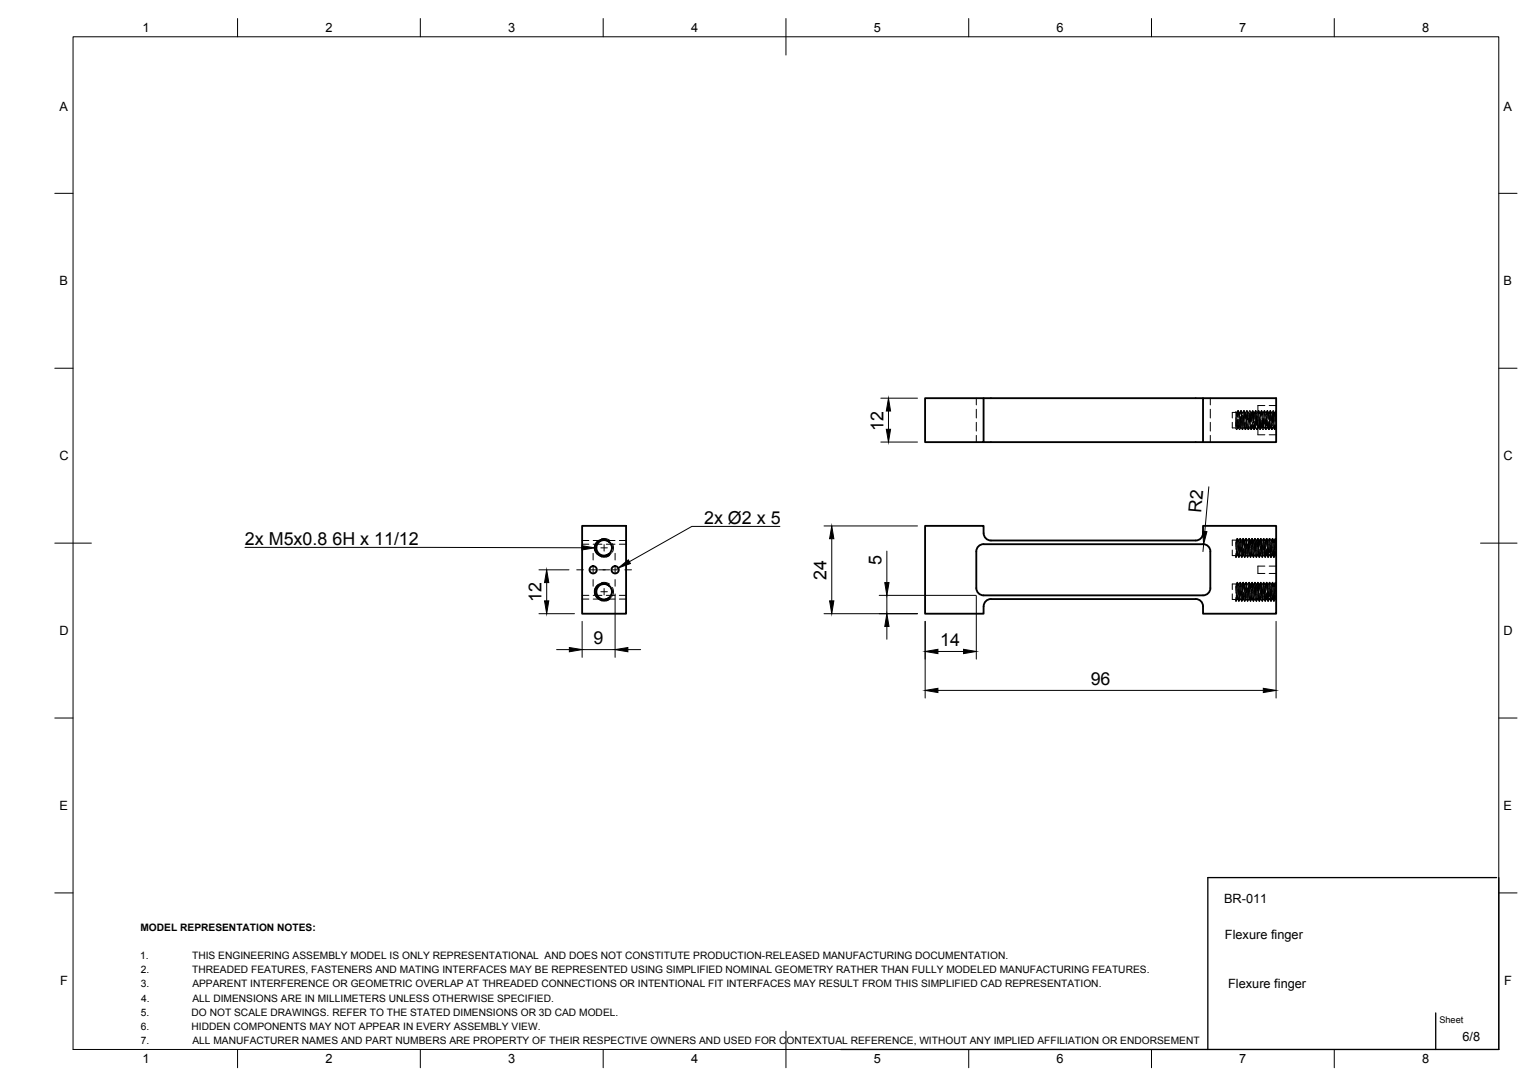
ISO-10303-21;
HEADER;
/* Generated by software containing ST-Developer
 * from STEP Tools, Inc. (www.steptools.com) 
 */

FILE_DESCRIPTION(
/* description */ ('Independent pair of monolithic parallel-leaf compliant finger modules.
 Shared native part/module instances; external gripper actuator outsid
e scope. Whole-mm geometry,1mm webs,56mm straight span,12mm depth,32mm
 nominal contact gap. Undeformed CAD reference; material condition, el
astic range, fatigue and gripping force unassigned.'),
/* implementation_level */ '2;1');

FILE_NAME(
/* name */ 'Flexure finger.step',
/* time_stamp */ '2026-11-07T22:36:16-08:00',
/* author */ (''),
/* organization */ (''),
/* preprocessor_version */ 'ST-DEVELOPER v20.2',
/* originating_system */ 'Autodesk Translation Framework v15.17.0.0',
/* authorisation */ '');

FILE_SCHEMA (('AUTOMOTIVE_DESIGN { 1 0 10303 214 3 1 1 }'));
ENDSEC;

DATA;
#10=MECHANICAL_DESIGN_GEOMETRIC_PRESENTATION_REPRESENTATION('',(#330),#13801);
#56=B_SPLINE_SURFACE_WITH_KNOTS('',3,3,((#7071,#7072,#7073,#7074,#7075,
#7076,#7077,#7078,#7079,#7080,#7081,#7082,#7083,#7084,#7085,#7086,#7087,
#7088,#7089,#7090,#7091,#7092,#7093,#7094,#7095,#7096,#7097,#7098,#7099,
#7100,#7101,#7102,#7103,#7104,#7105,#7106,#7107,#7108,#7109,#7110,#7111,
#7112,#7113,#7114,#7115,#7116,#7117,#7118,#7119,#7120,#7121,#7122,#7123,
#7124,#7125,#7126,#7127,#7128,#7129,#7130,#7131,#7132,#7133,#7134,#7135,
#7136,#7137,#7138,#7139,#7140,#7141,#7142,#7143,#7144,#7145,#7146,#7147,
#7148,#7149,#7150,#7151,#7152,#7153,#7154,#7155,#7156,#7157,#7158,#7159,
#7160,#7161,#7162),(#7163,#7164,#7165,#7166,#7167,#7168,#7169,#7170,#7171,
#7172,#7173,#7174,#7175,#7176,#7177,#7178,#7179,#7180,#7181,#7182,#7183,
#7184,#7185,#7186,#7187,#7188,#7189,#7190,#7191,#7192,#7193,#7194,#7195,
#7196,#7197,#7198,#7199,#7200,#7201,#7202,#7203,#7204,#7205,#7206,#7207,
#7208,#7209,#7210,#7211,#7212,#7213,#7214,#7215,#7216,#7217,#7218,#7219,
#7220,#7221,#7222,#7223,#7224,#7225,#7226,#7227,#7228,#7229,#7230,#7231,
#7232,#7233,#7234,#7235,#7236,#7237,#7238,#7239,#7240,#7241,#7242,#7243,
#7244,#7245,#7246,#7247,#7248,#7249,#7250,#7251,#7252,#7253,#7254),(#7255,
#7256,#7257,#7258,#7259,#7260,#7261,#7262,#7263,#7264,#7265,#7266,#7267,
#7268,#7269,#7270,#7271,#7272,#7273,#7274,#7275,#7276,#7277,#7278,#7279,
#7280,#7281,#7282,#7283,#7284,#7285,#7286,#7287,#7288,#7289,#7290,#7291,
#7292,#7293,#7294,#7295,#7296,#7297,#7298,#7299,#7300,#7301,#7302,#7303,
#7304,#7305,#7306,#7307,#7308,#7309,#7310,#7311,#7312,#7313,#7314,#7315,
#7316,#7317,#7318,#7319,#7320,#7321,#7322,#7323,#7324,#7325,#7326,#7327,
#7328,#7329,#7330,#7331,#7332,#7333,#7334,#7335,#7336,#7337,#7338,#7339,
#7340,#7341,#7342,#7343,#7344,#7345,#7346),(#7347,#7348,#7349,#7350,#7351,
#7352,#7353,#7354,#7355,#7356,#7357,#7358,#7359,#7360,#7361,#7362,#7363,
#7364,#7365,#7366,#7367,#7368,#7369,#7370,#7371,#7372,#7373,#7374,#7375,
#7376,#7377,#7378,#7379,#7380,#7381,#7382,#7383,#7384,#7385,#7386,#7387,
#7388,#7389,#7390,#7391,#7392,#7393,#7394,#7395,#7396,#7397,#7398,#7399,
#7400,#7401,#7402,#7403,#7404,#7405,#7406,#7407,#7408,#7409,#7410,#7411,
#7412,#7413,#7414,#7415,#7416,#7417,#7418,#7419,#7420,#7421,#7422,#7423,
#7424,#7425,#7426,#7427,#7428,#7429,#7430,#7431,#7432,#7433,#7434,#7435,
#7436,#7437,#7438)),.UNSPECIFIED.,.F.,.F.,.F.,(4,4),(4,1,1,1,1,1,1,1,1,
1,1,1,1,1,1,1,1,1,1,1,1,1,1,1,1,1,1,1,1,1,1,1,1,1,1,1,1,1,1,1,1,1,1,1,1,
1,1,1,1,1,1,1,1,1,1,1,1,1,1,1,1,1,1,1,1,1,1,1,1,1,1,1,1,1,1,1,1,1,1,1,1,
1,1,1,1,1,1,1,1,4),(0.,0.0511532338502008),(11.8669242345263,12.8602116589039,
13.8534990832815,14.8467865076592,15.8400739320368,16.8333613564144,17.826648780792,
18.8199362051697,19.8132236295473,20.8065110539249,21.7997984783025,22.7930859026802,
23.7863733270578,24.7796607514354,25.772948175813,26.7662356001907,27.7595230245683,
28.7528104489459,29.7460978733235,30.7393852977012,31.7326727220788,32.7259601464564,
33.719247570834,34.7125349952117,35.7058224195893,36.6991098439669,37.6923972683445,
38.6856846927222,39.6789721170998,40.6722595414774,41.6655469658551,42.6588343902327,
43.6521218146103,44.6454092389879,45.6386966633656,46.6319840877432,47.6252715121208,
48.6185589364984,49.6118463608761,50.6051337852537,51.5984212096313,52.5917086340089,
53.5849960583866,54.5782834827642,55.5715709071418,56.5648583315194,57.5581457558971,
58.5514331802747,59.5447206046523,60.5380080290299,61.5312954534076,62.5245828777852,
63.5178703021628,64.5111577265404,65.5044451509181,66.4977325752957,67.4910199996733,
68.4843074240509,69.4775948484286,70.4708822728062,71.4641696971838,72.4574571215614,
73.4507445459391,74.4440319703167,75.4373193946943,76.430606819072,77.4238942434496,
78.4171816678272,79.4104690922048,80.4037565165825,81.3970439409601,82.3903313653377,
83.3836187897153,84.376906214093,85.3701936384706,86.3634810628482,87.3567684872258,
88.3500559116035,89.3433433359811,90.3366307603587,91.3299181847363,92.323205609114,
93.3164930334916,94.3097804578692,95.3030678822468,96.2963553066245,97.2896427310021,
98.2829301553797,99.2762175797573,100.269505004135),.UNSPECIFIED.);
#57=B_SPLINE_SURFACE_WITH_KNOTS('',3,3,((#7555,#7556,#7557,#7558,#7559,
#7560,#7561,#7562,#7563,#7564,#7565,#7566,#7567,#7568,#7569,#7570,#7571,
#7572,#7573,#7574,#7575,#7576,#7577,#7578,#7579,#7580,#7581,#7582,#7583,
#7584,#7585,#7586,#7587,#7588,#7589,#7590,#7591,#7592,#7593,#7594,#7595,
#7596,#7597,#7598,#7599,#7600,#7601,#7602,#7603,#7604,#7605,#7606,#7607,
#7608,#7609,#7610,#7611,#7612,#7613,#7614,#7615,#7616,#7617,#7618,#7619,
#7620,#7621,#7622,#7623,#7624,#7625,#7626,#7627,#7628,#7629,#7630,#7631,
#7632,#7633,#7634,#7635,#7636,#7637,#7638,#7639,#7640,#7641,#7642,#7643,
#7644,#7645,#7646),(#7647,#7648,#7649,#7650,#7651,#7652,#7653,#7654,#7655,
#7656,#7657,#7658,#7659,#7660,#7661,#7662,#7663,#7664,#7665,#7666,#7667,
#7668,#7669,#7670,#7671,#7672,#7673,#7674,#7675,#7676,#7677,#7678,#7679,
#7680,#7681,#7682,#7683,#7684,#7685,#7686,#7687,#7688,#7689,#7690,#7691,
#7692,#7693,#7694,#7695,#7696,#7697,#7698,#7699,#7700,#7701,#7702,#7703,
#7704,#7705,#7706,#7707,#7708,#7709,#7710,#7711,#7712,#7713,#7714,#7715,
#7716,#7717,#7718,#7719,#7720,#7721,#7722,#7723,#7724,#7725,#7726,#7727,
#7728,#7729,#7730,#7731,#7732,#7733,#7734,#7735,#7736,#7737,#7738),(#7739,
#7740,#7741,#7742,#7743,#7744,#7745,#7746,#7747,#7748,#7749,#7750,#7751,
#7752,#7753,#7754,#7755,#7756,#7757,#7758,#7759,#7760,#7761,#7762,#7763,
#7764,#7765,#7766,#7767,#7768,#7769,#7770,#7771,#7772,#7773,#7774,#7775,
#7776,#7777,#7778,#7779,#7780,#7781,#7782,#7783,#7784,#7785,#7786,#7787,
#7788,#7789,#7790,#7791,#7792,#7793,#7794,#7795,#7796,#7797,#7798,#7799,
#7800,#7801,#7802,#7803,#7804,#7805,#7806,#7807,#7808,#7809,#7810,#7811,
#7812,#7813,#7814,#7815,#7816,#7817,#7818,#7819,#7820,#7821,#7822,#7823,
#7824,#7825,#7826,#7827,#7828,#7829,#7830),(#7831,#7832,#7833,#7834,#7835,
#7836,#7837,#7838,#7839,#7840,#7841,#7842,#7843,#7844,#7845,#7846,#7847,
#7848,#7849,#7850,#7851,#7852,#7853,#7854,#7855,#7856,#7857,#7858,#7859,
#7860,#7861,#7862,#7863,#7864,#7865,#7866,#7867,#7868,#7869,#7870,#7871,
#7872,#7873,#7874,#7875,#7876,#7877,#7878,#7879,#7880,#7881,#7882,#7883,
#7884,#7885,#7886,#7887,#7888,#7889,#7890,#7891,#7892,#7893,#7894,#7895,
#7896,#7897,#7898,#7899,#7900,#7901,#7902,#7903,#7904,#7905,#7906,#7907,
#7908,#7909,#7910,#7911,#7912,#7913,#7914,#7915,#7916,#7917,#7918,#7919,
#7920,#7921,#7922)),.UNSPECIFIED.,.F.,.F.,.F.,(4,4),(4,1,1,1,1,1,1,1,1,
1,1,1,1,1,1,1,1,1,1,1,1,1,1,1,1,1,1,1,1,1,1,1,1,1,1,1,1,1,1,1,1,1,1,1,1,
1,1,1,1,1,1,1,1,1,1,1,1,1,1,1,1,1,1,1,1,1,1,1,1,1,1,1,1,1,1,1,1,1,1,1,1,
1,1,1,1,1,1,1,1,4),(0.,0.0511532338502008),(14.3986268518923,15.3919142762699,
16.3852017006476,17.3784891250252,18.3717765494028,19.3650639737804,20.3583513981581,
21.3516388225357,22.3449262469133,23.3382136712909,24.3315010956686,25.3247885200462,
26.3180759444238,27.3113633688014,28.3046507931791,29.2979382175567,30.2912256419343,
31.284513066312,32.2778004906896,33.2710879150672,34.2643753394448,35.2576627638225,
36.2509501882001,37.2442376125777,38.2375250369553,39.230812461333,40.2240998857106,
41.2173873100882,42.2106747344658,43.2039621588435,44.1972495832211,45.1905370075987,
46.1838244319763,47.177111856354,48.1703992807316,49.1636867051092,50.1569741294868,
51.1502615538645,52.1435489782421,53.1368364026197,54.1301238269973,55.123411251375,
56.1166986757526,57.1099861001302,58.1032735245078,59.0965609488855,60.0898483732631,
61.0831357976407,62.0764232220183,63.069710646396,64.0629980707736,65.0562854951512,
66.0495729195289,67.0428603439065,68.0361477682841,69.0294351926617,70.0227226170393,
71.016010041417,72.0092974657946,73.0025848901722,73.9958723145499,74.9891597389275,
75.9824471633051,76.9757345876827,77.9690220120604,78.962309436438,79.9555968608156,
80.9488842851932,81.9421717095709,82.9354591339485,83.9287465583261,84.9220339827037,
85.9153214070814,86.908608831459,87.9018962558366,88.8951836802142,89.8884711045919,
90.8817585289695,91.8750459533471,92.8683333777248,93.8616208021024,94.85490822648,
95.8481956508576,96.8414830752353,97.8347704996129,98.8280579239905,99.8213453483681,
100.814632772746,101.807920197123,102.801207621501),.UNSPECIFIED.);
#58=B_SPLINE_SURFACE_WITH_KNOTS('',3,3,((#8239,#8240,#8241,#8242,#8243,
#8244,#8245,#8246,#8247,#8248,#8249,#8250,#8251,#8252,#8253,#8254,#8255,
#8256,#8257,#8258,#8259,#8260,#8261,#8262,#8263,#8264,#8265,#8266,#8267,
#8268,#8269,#8270,#8271,#8272,#8273,#8274,#8275,#8276,#8277,#8278,#8279,
#8280,#8281,#8282,#8283,#8284,#8285,#8286,#8287,#8288,#8289,#8290,#8291,
#8292,#8293,#8294,#8295,#8296,#8297,#8298,#8299,#8300,#8301,#8302,#8303,
#8304,#8305,#8306,#8307,#8308,#8309,#8310,#8311,#8312,#8313,#8314,#8315,
#8316,#8317,#8318,#8319,#8320,#8321,#8322,#8323,#8324,#8325,#8326,#8327,
#8328,#8329,#8330),(#8331,#8332,#8333,#8334,#8335,#8336,#8337,#8338,#8339,
#8340,#8341,#8342,#8343,#8344,#8345,#8346,#8347,#8348,#8349,#8350,#8351,
#8352,#8353,#8354,#8355,#8356,#8357,#8358,#8359,#8360,#8361,#8362,#8363,
#8364,#8365,#8366,#8367,#8368,#8369,#8370,#8371,#8372,#8373,#8374,#8375,
#8376,#8377,#8378,#8379,#8380,#8381,#8382,#8383,#8384,#8385,#8386,#8387,
#8388,#8389,#8390,#8391,#8392,#8393,#8394,#8395,#8396,#8397,#8398,#8399,
#8400,#8401,#8402,#8403,#8404,#8405,#8406,#8407,#8408,#8409,#8410,#8411,
#8412,#8413,#8414,#8415,#8416,#8417,#8418,#8419,#8420,#8421,#8422),(#8423,
#8424,#8425,#8426,#8427,#8428,#8429,#8430,#8431,#8432,#8433,#8434,#8435,
#8436,#8437,#8438,#8439,#8440,#8441,#8442,#8443,#8444,#8445,#8446,#8447,
#8448,#8449,#8450,#8451,#8452,#8453,#8454,#8455,#8456,#8457,#8458,#8459,
#8460,#8461,#8462,#8463,#8464,#8465,#8466,#8467,#8468,#8469,#8470,#8471,
#8472,#8473,#8474,#8475,#8476,#8477,#8478,#8479,#8480,#8481,#8482,#8483,
#8484,#8485,#8486,#8487,#8488,#8489,#8490,#8491,#8492,#8493,#8494,#8495,
#8496,#8497,#8498,#8499,#8500,#8501,#8502,#8503,#8504,#8505,#8506,#8507,
#8508,#8509,#8510,#8511,#8512,#8513,#8514),(#8515,#8516,#8517,#8518,#8519,
#8520,#8521,#8522,#8523,#8524,#8525,#8526,#8527,#8528,#8529,#8530,#8531,
#8532,#8533,#8534,#8535,#8536,#8537,#8538,#8539,#8540,#8541,#8542,#8543,
#8544,#8545,#8546,#8547,#8548,#8549,#8550,#8551,#8552,#8553,#8554,#8555,
#8556,#8557,#8558,#8559,#8560,#8561,#8562,#8563,#8564,#8565,#8566,#8567,
#8568,#8569,#8570,#8571,#8572,#8573,#8574,#8575,#8576,#8577,#8578,#8579,
#8580,#8581,#8582,#8583,#8584,#8585,#8586,#8587,#8588,#8589,#8590,#8591,
#8592,#8593,#8594,#8595,#8596,#8597,#8598,#8599,#8600,#8601,#8602,#8603,
#8604,#8605,#8606)),.UNSPECIFIED.,.F.,.F.,.F.,(4,4),(4,1,1,1,1,1,1,1,1,
1,1,1,1,1,1,1,1,1,1,1,1,1,1,1,1,1,1,1,1,1,1,1,1,1,1,1,1,1,1,1,1,1,1,1,1,
1,1,1,1,1,1,1,1,1,1,1,1,1,1,1,1,1,1,1,1,1,1,1,1,1,1,1,1,1,1,1,1,1,1,1,1,
1,1,1,1,1,1,1,1,4),(0.,0.0511532338502008),(11.8669242345263,12.8602116589039,
13.8534990832815,14.8467865076592,15.8400739320368,16.8333613564144,17.826648780792,
18.8199362051697,19.8132236295473,20.8065110539249,21.7997984783025,22.7930859026802,
23.7863733270578,24.7796607514354,25.772948175813,26.7662356001907,27.7595230245683,
28.7528104489459,29.7460978733235,30.7393852977012,31.7326727220788,32.7259601464564,
33.719247570834,34.7125349952117,35.7058224195893,36.6991098439669,37.6923972683445,
38.6856846927222,39.6789721170998,40.6722595414774,41.6655469658551,42.6588343902327,
43.6521218146103,44.6454092389879,45.6386966633656,46.6319840877432,47.6252715121208,
48.6185589364984,49.6118463608761,50.6051337852537,51.5984212096313,52.5917086340089,
53.5849960583866,54.5782834827642,55.5715709071418,56.5648583315194,57.5581457558971,
58.5514331802747,59.5447206046523,60.5380080290299,61.5312954534076,62.5245828777852,
63.5178703021628,64.5111577265404,65.5044451509181,66.4977325752957,67.4910199996733,
68.4843074240509,69.4775948484286,70.4708822728062,71.4641696971838,72.4574571215614,
73.4507445459391,74.4440319703167,75.4373193946943,76.430606819072,77.4238942434496,
78.4171816678272,79.4104690922048,80.4037565165825,81.3970439409601,82.3903313653377,
83.3836187897153,84.376906214093,85.3701936384706,86.3634810628482,87.3567684872258,
88.3500559116035,89.3433433359811,90.3366307603587,91.3299181847363,92.323205609114,
93.3164930334916,94.3097804578692,95.3030678822468,96.2963553066245,97.2896427310021,
98.2829301553797,99.2762175797573,100.269505004135),.UNSPECIFIED.);
#59=B_SPLINE_SURFACE_WITH_KNOTS('',3,3,((#8723,#8724,#8725,#8726,#8727,
#8728,#8729,#8730,#8731,#8732,#8733,#8734,#8735,#8736,#8737,#8738,#8739,
#8740,#8741,#8742,#8743,#8744,#8745,#8746,#8747,#8748,#8749,#8750,#8751,
#8752,#8753,#8754,#8755,#8756,#8757,#8758,#8759,#8760,#8761,#8762,#8763,
#8764,#8765,#8766,#8767,#8768,#8769,#8770,#8771,#8772,#8773,#8774,#8775,
#8776,#8777,#8778,#8779,#8780,#8781,#8782,#8783,#8784,#8785,#8786,#8787,
#8788,#8789,#8790,#8791,#8792,#8793,#8794,#8795,#8796,#8797,#8798,#8799,
#8800,#8801,#8802,#8803,#8804,#8805,#8806,#8807,#8808,#8809,#8810,#8811,
#8812,#8813,#8814),(#8815,#8816,#8817,#8818,#8819,#8820,#8821,#8822,#8823,
#8824,#8825,#8826,#8827,#8828,#8829,#8830,#8831,#8832,#8833,#8834,#8835,
#8836,#8837,#8838,#8839,#8840,#8841,#8842,#8843,#8844,#8845,#8846,#8847,
#8848,#8849,#8850,#8851,#8852,#8853,#8854,#8855,#8856,#8857,#8858,#8859,
#8860,#8861,#8862,#8863,#8864,#8865,#8866,#8867,#8868,#8869,#8870,#8871,
#8872,#8873,#8874,#8875,#8876,#8877,#8878,#8879,#8880,#8881,#8882,#8883,
#8884,#8885,#8886,#8887,#8888,#8889,#8890,#8891,#8892,#8893,#8894,#8895,
#8896,#8897,#8898,#8899,#8900,#8901,#8902,#8903,#8904,#8905,#8906),(#8907,
#8908,#8909,#8910,#8911,#8912,#8913,#8914,#8915,#8916,#8917,#8918,#8919,
#8920,#8921,#8922,#8923,#8924,#8925,#8926,#8927,#8928,#8929,#8930,#8931,
#8932,#8933,#8934,#8935,#8936,#8937,#8938,#8939,#8940,#8941,#8942,#8943,
#8944,#8945,#8946,#8947,#8948,#8949,#8950,#8951,#8952,#8953,#8954,#8955,
#8956,#8957,#8958,#8959,#8960,#8961,#8962,#8963,#8964,#8965,#8966,#8967,
#8968,#8969,#8970,#8971,#8972,#8973,#8974,#8975,#8976,#8977,#8978,#8979,
#8980,#8981,#8982,#8983,#8984,#8985,#8986,#8987,#8988,#8989,#8990,#8991,
#8992,#8993,#8994,#8995,#8996,#8997,#8998),(#8999,#9000,#9001,#9002,#9003,
#9004,#9005,#9006,#9007,#9008,#9009,#9010,#9011,#9012,#9013,#9014,#9015,
#9016,#9017,#9018,#9019,#9020,#9021,#9022,#9023,#9024,#9025,#9026,#9027,
#9028,#9029,#9030,#9031,#9032,#9033,#9034,#9035,#9036,#9037,#9038,#9039,
#9040,#9041,#9042,#9043,#9044,#9045,#9046,#9047,#9048,#9049,#9050,#9051,
#9052,#9053,#9054,#9055,#9056,#9057,#9058,#9059,#9060,#9061,#9062,#9063,
#9064,#9065,#9066,#9067,#9068,#9069,#9070,#9071,#9072,#9073,#9074,#9075,
#9076,#9077,#9078,#9079,#9080,#9081,#9082,#9083,#9084,#9085,#9086,#9087,
#9088,#9089,#9090)),.UNSPECIFIED.,.F.,.F.,.F.,(4,4),(4,1,1,1,1,1,1,1,1,
1,1,1,1,1,1,1,1,1,1,1,1,1,1,1,1,1,1,1,1,1,1,1,1,1,1,1,1,1,1,1,1,1,1,1,1,
1,1,1,1,1,1,1,1,1,1,1,1,1,1,1,1,1,1,1,1,1,1,1,1,1,1,1,1,1,1,1,1,1,1,1,1,
1,1,1,1,1,1,1,1,4),(0.,0.0511532338502008),(14.3986268518923,15.3919142762699,
16.3852017006476,17.3784891250252,18.3717765494028,19.3650639737804,20.3583513981581,
21.3516388225357,22.3449262469133,23.3382136712909,24.3315010956686,25.3247885200462,
26.3180759444238,27.3113633688014,28.3046507931791,29.2979382175567,30.2912256419343,
31.284513066312,32.2778004906896,33.2710879150672,34.2643753394448,35.2576627638225,
36.2509501882001,37.2442376125777,38.2375250369553,39.230812461333,40.2240998857106,
41.2173873100882,42.2106747344658,43.2039621588435,44.1972495832211,45.1905370075987,
46.1838244319763,47.177111856354,48.1703992807316,49.1636867051092,50.1569741294868,
51.1502615538645,52.1435489782421,53.1368364026197,54.1301238269973,55.123411251375,
56.1166986757526,57.1099861001302,58.1032735245078,59.0965609488855,60.0898483732631,
61.0831357976407,62.0764232220183,63.069710646396,64.0629980707736,65.0562854951512,
66.0495729195289,67.0428603439065,68.0361477682841,69.0294351926617,70.0227226170393,
71.016010041417,72.0092974657946,73.0025848901722,73.9958723145499,74.9891597389275,
75.9824471633051,76.9757345876827,77.9690220120604,78.962309436438,79.9555968608156,
80.9488842851932,81.9421717095709,82.9354591339485,83.9287465583261,84.9220339827037,
85.9153214070814,86.908608831459,87.9018962558366,88.8951836802142,89.8884711045919,
90.8817585289695,91.8750459533471,92.8683333777248,93.8616208021024,94.85490822648,
95.8481956508576,96.8414830752353,97.8347704996129,98.8280579239905,99.8213453483681,
100.814632772746,101.807920197123,102.801207621501),.UNSPECIFIED.);
#62=B_SPLINE_CURVE_WITH_KNOTS('',3,(#4900,#4901,#4902,#4903,#4904,#4905,
#4906,#4907,#4908,#4909,#4910,#4911,#4912,#4913,#4914,#4915,#4916,#4917,
#4918),.UNSPECIFIED.,.F.,.F.,(4,3,3,3,3,3,4),(82.9907454093912,83.4361436477206,
84.4294310720982,85.4227184964758,86.4160059208535,87.4092933452311,88.4025807696087),
 .UNSPECIFIED.);
#63=B_SPLINE_CURVE_WITH_KNOTS('',3,(#4922,#4923,#4924,#4925),
 .UNSPECIFIED.,.F.,.F.,(4,4),(-86.3937979737193,-85.5224480267573),
 .UNSPECIFIED.);
#64=B_SPLINE_CURVE_WITH_KNOTS('',3,(#4929,#4930,#4931,#4932,#4933,#4934,
#4935,#4936,#4937,#4938,#4939,#4940,#4941,#4942,#4943,#4944,#4945,#4946,
#4947,#4948,#4949,#4950,#4951,#4952,#4953),.UNSPECIFIED.,.F.,.F.,(4,3,3,
3,3,3,3,3,4),(-85.5224480267573,-85.4227184964758,-84.4294310720982,-83.4361436477206,
-82.442856223343,-81.4495687989653,-80.4562813745877,-79.4629939502101,
-79.2392627195777),.UNSPECIFIED.);
#65=B_SPLINE_CURVE_WITH_KNOTS('',3,(#4958,#4959,#4960,#4961,#4962,#4963,
#4964,#4965,#4966,#4967,#4968,#4969,#4970,#4971,#4972,#4973,#4974,#4975,
#4976,#4977,#4978,#4979),.UNSPECIFIED.,.F.,.F.,(4,3,3,3,3,3,3,4),(76.7075601022116,
77.4764191014548,78.4697065258324,79.4629939502101,80.4562813745877,81.4495687989653,
82.442856223343,82.9907454093912),.UNSPECIFIED.);
#66=B_SPLINE_CURVE_WITH_KNOTS('',3,(#4980,#4981,#4982,#4983,#4984,#4985,
#4986,#4987,#4988,#4989,#4990,#4991,#4992,#4993,#4994,#4995,#4996,#4997,
#4998,#4999,#5000,#5001),.UNSPECIFIED.,.F.,.F.,(4,3,3,3,3,3,3,4),(-79.2392627195777,
-78.4697065258324,-77.4764191014548,-76.4831316770772,-75.4898442526996,
-74.4965568283219,-73.5032694039443,-72.9560774123981),.UNSPECIFIED.);
#67=B_SPLINE_CURVE_WITH_KNOTS('',3,(#5006,#5007,#5008,#5009,#5010,#5011,
#5012,#5013,#5014,#5015,#5016,#5017,#5018,#5019,#5020,#5021,#5022,#5023,
#5024,#5025,#5026,#5027,#5028,#5029,#5030),.UNSPECIFIED.,.F.,.F.,(4,3,3,
3,3,3,3,3,4),(70.424374795032,70.5234071308114,71.516694555189,72.5099819795667,
73.5032694039443,74.4965568283219,75.4898442526996,76.4831316770772,76.7075601022116),
 .UNSPECIFIED.);
#68=B_SPLINE_CURVE_WITH_KNOTS('',3,(#5031,#5032,#5033,#5034,#5035,#5036,
#5037,#5038,#5039,#5040,#5041,#5042,#5043,#5044,#5045,#5046,#5047,#5048,
#5049,#5050,#5051,#5052),.UNSPECIFIED.,.F.,.F.,(4,3,3,3,3,3,3,4),(-72.9560774123981,
-72.5099819795667,-71.516694555189,-70.5234071308114,-69.5301197064338,
-68.5368322820562,-67.5435448576786,-66.6728921052185),.UNSPECIFIED.);
#69=B_SPLINE_CURVE_WITH_KNOTS('',3,(#5057,#5058,#5059,#5060,#5061,#5062,
#5063,#5064,#5065,#5066,#5067,#5068,#5069,#5070,#5071,#5072,#5073,#5074,
#5075,#5076,#5077,#5078),.UNSPECIFIED.,.F.,.F.,(4,3,3,3,3,3,3,4),(64.1411894878524,
64.5636825845457,65.5569700089233,66.5502574333009,67.5435448576786,68.5368322820562,
69.5301197064338,70.424374795032),.UNSPECIFIED.);
#70=B_SPLINE_CURVE_WITH_KNOTS('',3,(#5079,#5080,#5081,#5082,#5083,#5084,
#5085,#5086,#5087,#5088,#5089,#5090,#5091,#5092,#5093,#5094,#5095,#5096,
#5097,#5098,#5099,#5100,#5101,#5102,#5103),.UNSPECIFIED.,.F.,.F.,(4,3,3,
3,3,3,3,3,4),(-66.6728921052185,-66.550257433301,-65.5569700089233,-64.5636825845457,
-63.5703951601681,-62.5771077357904,-61.5838203114128,-60.5905328870352,
-60.3897067980389),.UNSPECIFIED.);
#71=B_SPLINE_CURVE_WITH_KNOTS('',3,(#5108,#5109,#5110,#5111,#5112,#5113,
#5114,#5115,#5116,#5117,#5118,#5119,#5120,#5121,#5122,#5123,#5124,#5125,
#5126,#5127,#5128,#5129),.UNSPECIFIED.,.F.,.F.,(4,3,3,3,3,3,3,4),(57.8580041806728,
58.6039580382799,59.5972454626575,60.5905328870352,61.5838203114128,62.5771077357904,
63.570395160168,64.1411894878524),.UNSPECIFIED.);
#72=B_SPLINE_CURVE_WITH_KNOTS('',3,(#5130,#5131,#5132,#5133,#5134,#5135,
#5136,#5137,#5138,#5139,#5140,#5141,#5142,#5143,#5144,#5145,#5146,#5147,
#5148,#5149,#5150,#5151),.UNSPECIFIED.,.F.,.F.,(4,3,3,3,3,3,3,4),(-60.3897067980389,
-59.5972454626576,-58.6039580382799,-57.6106706139023,-56.6173831895247,
-55.624095765147,-54.6308083407694,-54.1065214908593),.UNSPECIFIED.);
#73=B_SPLINE_CURVE_WITH_KNOTS('',3,(#5156,#5157,#5158,#5159,#5160,#5161,
#5162,#5163,#5164,#5165,#5166,#5167,#5168,#5169,#5170,#5171,#5172,#5173,
#5174,#5175,#5176,#5177,#5178,#5179,#5180),.UNSPECIFIED.,.F.,.F.,(4,3,3,
3,3,3,3,3,4),(51.5748188734932,51.6509460676365,52.6442334920142,53.6375209163918,
54.6308083407694,55.624095765147,56.6173831895247,57.6106706139023,57.8580041806728),
 .UNSPECIFIED.);
#74=B_SPLINE_CURVE_WITH_KNOTS('',3,(#5181,#5182,#5183,#5184,#5185,#5186,
#5187,#5188,#5189,#5190,#5191,#5192,#5193,#5194,#5195,#5196,#5197,#5198,
#5199,#5200,#5201,#5202),.UNSPECIFIED.,.F.,.F.,(4,3,3,3,3,3,3,4),(-54.1065214908593,
-53.6375209163918,-52.6442334920142,-51.6509460676365,-50.6576586432589,
-49.6643712188813,-48.6710837945037,-47.8233361836797),.UNSPECIFIED.);
#75=B_SPLINE_CURVE_WITH_KNOTS('',3,(#5207,#5208,#5209,#5210,#5211,#5212,
#5213,#5214,#5215,#5216,#5217,#5218,#5219,#5220,#5221,#5222,#5223,#5224,
#5225,#5226,#5227,#5228),.UNSPECIFIED.,.F.,.F.,(4,3,3,3,3,3,3,4),(45.2916335663136,
45.6912215213708,46.6845089457484,47.677796370126,48.6710837945037,49.6643712188813,
50.6576586432589,51.5748188734932),.UNSPECIFIED.);
#76=B_SPLINE_CURVE_WITH_KNOTS('',3,(#5229,#5230,#5231,#5232,#5233,#5234,
#5235,#5236,#5237,#5238,#5239,#5240,#5241,#5242,#5243,#5244,#5245,#5246,
#5247,#5248,#5249,#5250,#5251,#5252,#5253),.UNSPECIFIED.,.F.,.F.,(4,3,3,
3,3,3,3,3,4),(-47.8233361836797,-47.677796370126,-46.6845089457484,-45.6912215213708,
-44.6979340969932,-43.7046466726155,-42.7113592482379,-41.7180718238603,
-41.5401508765001),.UNSPECIFIED.);
#77=B_SPLINE_CURVE_WITH_KNOTS('',3,(#5258,#5259,#5260,#5261,#5262,#5263,
#5264,#5265,#5266,#5267,#5268,#5269,#5270,#5271,#5272,#5273,#5274,#5275,
#5276,#5277,#5278,#5279),.UNSPECIFIED.,.F.,.F.,(4,3,3,3,3,3,3,4),(39.008448259134,
39.731496975105,40.7247843994827,41.7180718238603,42.7113592482379,43.7046466726155,
44.6979340969932,45.2916335663136),.UNSPECIFIED.);
#78=B_SPLINE_CURVE_WITH_KNOTS('',3,(#5280,#5281,#5282,#5283,#5284,#5285,
#5286,#5287,#5288,#5289,#5290,#5291,#5292,#5293,#5294,#5295,#5296,#5297,
#5298,#5299,#5300,#5301),.UNSPECIFIED.,.F.,.F.,(4,3,3,3,3,3,3,4),(-41.5401508765001,
-40.7247843994827,-39.731496975105,-38.7382095507274,-37.7449221263498,
-36.7516347019722,-35.7583472775945,-35.2569655693205),.UNSPECIFIED.);
#79=B_SPLINE_CURVE_WITH_KNOTS('',3,(#5306,#5307,#5308,#5309,#5310,#5311,
#5312,#5313,#5314,#5315,#5316,#5317,#5318,#5319,#5320,#5321,#5322,#5323,
#5324,#5325,#5326,#5327,#5328,#5329,#5330),.UNSPECIFIED.,.F.,.F.,(4,3,3,
3,3,3,3,3,4),(32.7252629519544,32.7784850044617,33.7717724288393,34.7650598532169,
35.7583472775945,36.7516347019722,37.7449221263498,38.7382095507274,39.008448259134),
 .UNSPECIFIED.);
#80=B_SPLINE_CURVE_WITH_KNOTS('',3,(#5331,#5332,#5333,#5334,#5335,#5336,
#5337,#5338,#5339,#5340,#5341,#5342,#5343,#5344,#5345,#5346,#5347,#5348,
#5349,#5350,#5351,#5352),.UNSPECIFIED.,.F.,.F.,(4,3,3,3,3,3,3,4),(-35.2569655693205,
-34.7650598532169,-33.7717724288393,-32.7784850044617,-31.785197580084,
-30.7919101557064,-29.7986227313288,-28.973780262141),.UNSPECIFIED.);
#81=B_SPLINE_CURVE_WITH_KNOTS('',3,(#5357,#5358,#5359,#5360,#5361,#5362,
#5363,#5364,#5365,#5366,#5367,#5368,#5369,#5370,#5371,#5372,#5373,#5374,
#5375,#5376,#5377,#5378),.UNSPECIFIED.,.F.,.F.,(4,3,3,3,3,3,3,4),(26.4420776447749,
26.8187604581959,27.8120478825735,28.8053353069512,29.7986227313288,30.7919101557064,
31.785197580084,32.7252629519544),.UNSPECIFIED.);
#82=B_SPLINE_CURVE_WITH_KNOTS('',3,(#5379,#5380,#5381,#5382,#5383,#5384,
#5385,#5386,#5387,#5388,#5389,#5390,#5391,#5392,#5393,#5394,#5395,#5396,
#5397,#5398,#5399,#5400,#5401,#5402,#5403),.UNSPECIFIED.,.F.,.F.,(4,3,3,
3,3,3,3,3,4),(-28.973780262141,-28.8053353069512,-27.8120478825735,-26.8187604581959,
-25.8254730338183,-24.8321856094406,-23.838898185063,-22.8456107606854,
-22.6905949549614),.UNSPECIFIED.);
#83=B_SPLINE_CURVE_WITH_KNOTS('',3,(#5408,#5409,#5410,#5411,#5412,#5413,
#5414,#5415,#5416,#5417,#5418,#5419,#5420,#5421,#5422,#5423,#5424,#5425,
#5426,#5427,#5428,#5429),.UNSPECIFIED.,.F.,.F.,(4,3,3,3,3,3,3,4),(20.1588923375953,
20.8590359119301,21.8523233363078,22.8456107606854,23.838898185063,24.8321856094406,
25.8254730338183,26.4420776447749),.UNSPECIFIED.);
#84=B_SPLINE_CURVE_WITH_KNOTS('',3,(#5430,#5431,#5432,#5433,#5434,#5435,
#5436,#5437,#5438,#5439,#5440,#5441,#5442,#5443,#5444,#5445,#5446,#5447,
#5448,#5449,#5450,#5451),.UNSPECIFIED.,.F.,.F.,(4,3,3,3,3,3,3,4),(-22.6905949549614,
-21.8523233363078,-20.8590359119301,-19.8657484875525,-18.8724610631749,
-17.8791736387973,-16.8858862144196,-16.4074096477818),.UNSPECIFIED.);
#85=B_SPLINE_CURVE_WITH_KNOTS('',3,(#5456,#5457,#5458,#5459,#5460,#5461,
#5462,#5463,#5464,#5465,#5466,#5467,#5468,#5469,#5470,#5471,#5472,#5473,
#5474,#5475,#5476,#5477,#5478,#5479,#5480),.UNSPECIFIED.,.F.,.F.,(4,3,3,
3,3,3,3,3,4),(13.8757070304157,13.9060239412868,14.8993113656644,15.892598790042,
16.8858862144196,17.8791736387973,18.8724610631749,19.8657484875525,20.1588923375953),
 .UNSPECIFIED.);
#86=B_SPLINE_CURVE_WITH_KNOTS('',3,(#5481,#5482,#5483,#5484,#5485,#5486,
#5487,#5488,#5489,#5490,#5491,#5492,#5493,#5494,#5495,#5496,#5497,#5498,
#5499,#5500,#5501,#5502),.UNSPECIFIED.,.F.,.F.,(4,3,3,3,3,3,3,4),(-16.4074096477818,
-15.892598790042,-14.8993113656644,-13.9060239412868,-12.9127365169091,
-11.9194490925315,-10.9261616681539,-10.1242243406022),.UNSPECIFIED.);
#87=B_SPLINE_CURVE_WITH_KNOTS('',3,(#5508,#5509,#5510,#5511,#5512,#5513,
#5514,#5515,#5516,#5517,#5518,#5519,#5520),.UNSPECIFIED.,.F.,.F.,(4,3,3,
3,4),(-3.84103903342261,-2.97986227313288,-1.98657484875525,-0.993287424377625,
0.),.UNSPECIFIED.);
#88=B_SPLINE_CURVE_WITH_KNOTS('',3,(#5523,#5524,#5525,#5526,#5527,#5528,
#5529,#5530,#5531,#5532,#5533,#5534,#5535,#5536,#5537,#5538,#5539,#5540,
#5541),.UNSPECIFIED.,.F.,.F.,(4,3,3,3,3,3,4),(2.00878279588941,2.97986227313288,
3.9731496975105,4.96643712188813,5.95972454626575,6.95301197064338,7.5925217232361),
 .UNSPECIFIED.);
#89=B_SPLINE_CURVE_WITH_KNOTS('',3,(#5547,#5548,#5549,#5550,#5551,#5552),
 .UNSPECIFIED.,.F.,.F.,(4,1,1,4),(97.3893722612836,98.2829301553797,99.2762175797573,
100.269505004135),.UNSPECIFIED.);
#90=B_SPLINE_CURVE_WITH_KNOTS('',3,(#5555,#5556,#5557,#5558,#5559,#5560,
#5561),.UNSPECIFIED.,.F.,.F.,(4,1,1,1,4),(97.3893722612836,97.8347704996129,
98.8280579239905,99.8213453483681,100.792424825612),.UNSPECIFIED.);
#91=B_SPLINE_CURVE_WITH_KNOTS('',3,(#5566,#5567,#5568,#5569,#5570,#5571,
#5572,#5573,#5574,#5575,#5576),.UNSPECIFIED.,.F.,.F.,(4,1,1,1,1,1,1,1,4),
(91.106186954104,91.3299181847363,92.323205609114,93.3164930334916,94.3097804578692,
95.3030678822468,96.2963553066245,97.2896427310021,97.3893722612836),
 .UNSPECIFIED.);
#92=B_SPLINE_CURVE_WITH_KNOTS('',3,(#5577,#5578,#5579,#5580,#5581,#5582,
#5583,#5584,#5585,#5586),.UNSPECIFIED.,.F.,.F.,(4,1,1,1,1,1,1,4),(91.106186954104,
91.8750459533471,92.8683333777248,93.8616208021024,94.85490822648,95.8481956508576,
96.8414830752353,97.3893722612836),.UNSPECIFIED.);
#93=B_SPLINE_CURVE_WITH_KNOTS('',3,(#5591,#5592,#5593,#5594,#5595,#5596,
#5597,#5598,#5599,#5600),.UNSPECIFIED.,.F.,.F.,(4,1,1,1,1,1,1,4),(84.8230016469244,
85.3701936384706,86.3634810628482,87.3567684872258,88.3500559116035,89.3433433359811,
90.3366307603587,91.106186954104),.UNSPECIFIED.);
#94=B_SPLINE_CURVE_WITH_KNOTS('',3,(#5601,#5602,#5603,#5604,#5605,#5606,
#5607,#5608,#5609,#5610,#5611),.UNSPECIFIED.,.F.,.F.,(4,1,1,1,1,1,1,1,4),
(84.8230016469244,84.9220339827037,85.9153214070814,86.908608831459,87.9018962558366,
88.8951836802142,89.8884711045919,90.8817585289695,91.106186954104),
 .UNSPECIFIED.);
#95=B_SPLINE_CURVE_WITH_KNOTS('',3,(#5616,#5617,#5618,#5619,#5620,#5621,
#5622,#5623,#5624,#5625),.UNSPECIFIED.,.F.,.F.,(4,1,1,1,1,1,1,4),(78.5398163397448,
79.4104690922048,80.4037565165825,81.3970439409601,82.3903313653377,83.3836187897153,
84.376906214093,84.8230016469244),.UNSPECIFIED.);
#96=B_SPLINE_CURVE_WITH_KNOTS('',3,(#5626,#5627,#5628,#5629,#5630,#5631,
#5632,#5633,#5634,#5635),.UNSPECIFIED.,.F.,.F.,(4,1,1,1,1,1,1,4),(78.5398163397448,
78.962309436438,79.9555968608156,80.9488842851932,81.9421717095709,82.9354591339485,
83.9287465583261,84.8230016469244),.UNSPECIFIED.);
#97=B_SPLINE_CURVE_WITH_KNOTS('',3,(#5640,#5641,#5642,#5643,#5644,#5645,
#5646,#5647,#5648,#5649,#5650),.UNSPECIFIED.,.F.,.F.,(4,1,1,1,1,1,1,1,4),
(72.2566310325652,72.4574571215614,73.4507445459391,74.4440319703167,75.4373193946943,
76.430606819072,77.4238942434496,78.4171816678272,78.5398163397448),
 .UNSPECIFIED.);
#98=B_SPLINE_CURVE_WITH_KNOTS('',3,(#5651,#5652,#5653,#5654,#5655,#5656,
#5657,#5658,#5659,#5660),.UNSPECIFIED.,.F.,.F.,(4,1,1,1,1,1,1,4),(72.2566310325652,
73.0025848901722,73.9958723145499,74.9891597389275,75.9824471633051,76.9757345876827,
77.9690220120604,78.5398163397448),.UNSPECIFIED.);
#99=B_SPLINE_CURVE_WITH_KNOTS('',3,(#5665,#5666,#5667,#5668,#5669,#5670,
#5671,#5672,#5673,#5674),.UNSPECIFIED.,.F.,.F.,(4,1,1,1,1,1,1,4),(65.9734457253856,
66.4977325752957,67.4910199996733,68.4843074240509,69.4775948484286,70.4708822728062,
71.4641696971838,72.2566310325652),.UNSPECIFIED.);
#100=B_SPLINE_CURVE_WITH_KNOTS('',3,(#5675,#5676,#5677,#5678,#5679,#5680,
#5681,#5682,#5683,#5684,#5685),.UNSPECIFIED.,.F.,.F.,(4,1,1,1,1,1,1,1,4),
(65.9734457253856,66.0495729195289,67.0428603439065,68.0361477682841,69.0294351926617,
70.0227226170393,71.016010041417,72.0092974657946,72.2566310325652),
 .UNSPECIFIED.);
#101=B_SPLINE_CURVE_WITH_KNOTS('',3,(#5690,#5691,#5692,#5693,#5694,#5695,
#5696,#5697,#5698,#5699),.UNSPECIFIED.,.F.,.F.,(4,1,1,1,1,1,1,4),(59.690260418206,
60.5380080290299,61.5312954534076,62.5245828777852,63.5178703021628,64.5111577265404,
65.5044451509181,65.9734457253856),.UNSPECIFIED.);
#102=B_SPLINE_CURVE_WITH_KNOTS('',3,(#5700,#5701,#5702,#5703,#5704,#5705,
#5706,#5707,#5708,#5709),.UNSPECIFIED.,.F.,.F.,(4,1,1,1,1,1,1,4),(59.690260418206,
60.0898483732631,61.0831357976407,62.0764232220183,63.069710646396,64.0629980707736,
65.0562854951512,65.9734457253856),.UNSPECIFIED.);
#103=B_SPLINE_CURVE_WITH_KNOTS('',3,(#5714,#5715,#5716,#5717,#5718,#5719,
#5720,#5721,#5722,#5723,#5724),.UNSPECIFIED.,.F.,.F.,(4,1,1,1,1,1,1,1,4),
(53.4070751110264,53.5849960583866,54.5782834827642,55.5715709071418,56.5648583315194,
57.5581457558971,58.5514331802747,59.5447206046523,59.690260418206),
 .UNSPECIFIED.);
#104=B_SPLINE_CURVE_WITH_KNOTS('',3,(#5725,#5726,#5727,#5728,#5729,#5730,
#5731,#5732,#5733,#5734),.UNSPECIFIED.,.F.,.F.,(4,1,1,1,1,1,1,4),(53.4070751110264,
54.1301238269973,55.123411251375,56.1166986757526,57.1099861001302,58.1032735245078,
59.0965609488855,59.690260418206),.UNSPECIFIED.);
#105=B_SPLINE_CURVE_WITH_KNOTS('',3,(#5739,#5740,#5741,#5742,#5743,#5744,
#5745,#5746,#5747,#5748),.UNSPECIFIED.,.F.,.F.,(4,1,1,1,1,1,1,4),(47.1238898038468,
47.6252715121208,48.6185589364984,49.6118463608761,50.6051337852537,51.5984212096313,
52.5917086340089,53.4070751110264),.UNSPECIFIED.);
#106=B_SPLINE_CURVE_WITH_KNOTS('',3,(#5749,#5750,#5751,#5752,#5753,#5754,
#5755,#5756,#5757,#5758,#5759),.UNSPECIFIED.,.F.,.F.,(4,1,1,1,1,1,1,1,4),
(47.1238898038468,47.177111856354,48.1703992807316,49.1636867051092,50.1569741294868,
51.1502615538645,52.1435489782421,53.1368364026197,53.4070751110264),
 .UNSPECIFIED.);
#107=B_SPLINE_CURVE_WITH_KNOTS('',3,(#5764,#5765,#5766,#5767,#5768,#5769,
#5770,#5771,#5772,#5773),.UNSPECIFIED.,.F.,.F.,(4,1,1,1,1,1,1,4),(40.8407044966673,
41.6655469658551,42.6588343902327,43.6521218146103,44.6454092389879,45.6386966633656,
46.6319840877432,47.1238898038468),.UNSPECIFIED.);
#108=B_SPLINE_CURVE_WITH_KNOTS('',3,(#5774,#5775,#5776,#5777,#5778,#5779,
#5780,#5781,#5782,#5783),.UNSPECIFIED.,.F.,.F.,(4,1,1,1,1,1,1,4),(40.8407044966672,
41.2173873100882,42.2106747344658,43.2039621588435,44.1972495832211,45.1905370075987,
46.1838244319763,47.1238898038468),.UNSPECIFIED.);
#109=B_SPLINE_CURVE_WITH_KNOTS('',3,(#5788,#5789,#5790,#5791,#5792,#5793,
#5794,#5795,#5796,#5797,#5798),.UNSPECIFIED.,.F.,.F.,(4,1,1,1,1,1,1,1,4),
(34.5575191894876,34.7125349952117,35.7058224195893,36.6991098439669,37.6923972683445,
38.6856846927222,39.6789721170998,40.6722595414774,40.8407044966673),
 .UNSPECIFIED.);
#110=B_SPLINE_CURVE_WITH_KNOTS('',3,(#5799,#5800,#5801,#5802,#5803,#5804,
#5805,#5806,#5807,#5808),.UNSPECIFIED.,.F.,.F.,(4,1,1,1,1,1,1,4),(34.5575191894876,
35.2576627638225,36.2509501882001,37.2442376125777,38.2375250369553,39.230812461333,
40.2240998857106,40.8407044966672),.UNSPECIFIED.);
#111=B_SPLINE_CURVE_WITH_KNOTS('',3,(#5813,#5814,#5815,#5816,#5817,#5818,
#5819,#5820,#5821,#5822),.UNSPECIFIED.,.F.,.F.,(4,1,1,1,1,1,1,4),(28.2743338823081,
28.7528104489459,29.7460978733235,30.7393852977012,31.7326727220788,32.7259601464564,
33.719247570834,34.5575191894876),.UNSPECIFIED.);
#112=B_SPLINE_CURVE_WITH_KNOTS('',3,(#5823,#5824,#5825,#5826,#5827,#5828,
#5829,#5830,#5831,#5832,#5833),.UNSPECIFIED.,.F.,.F.,(4,1,1,1,1,1,1,1,4),
(28.2743338823081,28.3046507931791,29.2979382175567,30.2912256419343,31.284513066312,
32.2778004906896,33.2710879150672,34.2643753394448,34.5575191894876),
 .UNSPECIFIED.);
#113=B_SPLINE_CURVE_WITH_KNOTS('',3,(#5838,#5839,#5840,#5841,#5842,#5843,
#5844,#5845,#5846,#5847),.UNSPECIFIED.,.F.,.F.,(4,1,1,1,1,1,1,4),(21.9911485751285,
22.7930859026802,23.7863733270578,24.7796607514354,25.772948175813,26.7662356001907,
27.7595230245683,28.2743338823081),.UNSPECIFIED.);
#114=B_SPLINE_CURVE_WITH_KNOTS('',3,(#5848,#5849,#5850,#5851,#5852,#5853,
#5854,#5855,#5856,#5857),.UNSPECIFIED.,.F.,.F.,(4,1,1,1,1,1,1,4),(21.9911485751285,
22.3449262469133,23.3382136712909,24.3315010956686,25.3247885200462,26.3180759444238,
27.3113633688014,28.2743338823081),.UNSPECIFIED.);
#115=B_SPLINE_CURVE_WITH_KNOTS('',3,(#5863,#5864,#5865,#5866,#5867),
 .UNSPECIFIED.,.F.,.F.,(4,1,4),(14.3986268518923,15.3919142762699,15.7079632679489),
 .UNSPECIFIED.);
#116=B_SPLINE_CURVE_WITH_KNOTS('',3,(#5870,#5871,#5872,#5873,#5874),
 .UNSPECIFIED.,.F.,.F.,(4,1,4),(13.8757070304157,14.8467865076592,15.7079632679489),
 .UNSPECIFIED.);
#117=B_SPLINE_CURVE_WITH_KNOTS('',3,(#5880,#5881,#5882,#5883,#5884,#5885,
#5886,#5887,#5888,#5889,#5890,#5891,#5892,#5893,#5894,#5895,#5896,#5897,
#5898),.UNSPECIFIED.,.F.,.F.,(4,3,3,3,3,3,4),(82.9907454093912,83.4361436477206,
84.4294310720982,85.4227184964758,86.4160059208535,87.4092933452311,88.4025807696087),
 .UNSPECIFIED.);
#118=B_SPLINE_CURVE_WITH_KNOTS('',3,(#5902,#5903,#5904,#5905),
 .UNSPECIFIED.,.F.,.F.,(4,4),(-86.3937979737193,-85.5224480267573),
 .UNSPECIFIED.);
#119=B_SPLINE_CURVE_WITH_KNOTS('',3,(#5909,#5910,#5911,#5912,#5913,#5914,
#5915,#5916,#5917,#5918,#5919,#5920,#5921,#5922,#5923,#5924,#5925,#5926,
#5927,#5928,#5929,#5930,#5931,#5932,#5933),.UNSPECIFIED.,.F.,.F.,(4,3,3,
3,3,3,3,3,4),(-85.5224480267573,-85.4227184964758,-84.4294310720982,-83.4361436477206,
-82.442856223343,-81.4495687989653,-80.4562813745877,-79.4629939502101,
-79.2392627195777),.UNSPECIFIED.);
#120=B_SPLINE_CURVE_WITH_KNOTS('',3,(#5938,#5939,#5940,#5941,#5942,#5943,
#5944,#5945,#5946,#5947,#5948,#5949,#5950,#5951,#5952,#5953,#5954,#5955,
#5956,#5957,#5958,#5959),.UNSPECIFIED.,.F.,.F.,(4,3,3,3,3,3,3,4),(76.7075601022116,
77.4764191014548,78.4697065258324,79.4629939502101,80.4562813745877,81.4495687989653,
82.442856223343,82.9907454093912),.UNSPECIFIED.);
#121=B_SPLINE_CURVE_WITH_KNOTS('',3,(#5960,#5961,#5962,#5963,#5964,#5965,
#5966,#5967,#5968,#5969,#5970,#5971,#5972,#5973,#5974,#5975,#5976,#5977,
#5978,#5979,#5980,#5981),.UNSPECIFIED.,.F.,.F.,(4,3,3,3,3,3,3,4),(-79.2392627195777,
-78.4697065258324,-77.4764191014548,-76.4831316770772,-75.4898442526996,
-74.4965568283219,-73.5032694039443,-72.9560774123981),.UNSPECIFIED.);
#122=B_SPLINE_CURVE_WITH_KNOTS('',3,(#5986,#5987,#5988,#5989,#5990,#5991,
#5992,#5993,#5994,#5995,#5996,#5997,#5998,#5999,#6000,#6001,#6002,#6003,
#6004,#6005,#6006,#6007,#6008,#6009,#6010),.UNSPECIFIED.,.F.,.F.,(4,3,3,
3,3,3,3,3,4),(70.424374795032,70.5234071308114,71.516694555189,72.5099819795667,
73.5032694039443,74.4965568283219,75.4898442526996,76.4831316770772,76.7075601022116),
 .UNSPECIFIED.);
#123=B_SPLINE_CURVE_WITH_KNOTS('',3,(#6011,#6012,#6013,#6014,#6015,#6016,
#6017,#6018,#6019,#6020,#6021,#6022,#6023,#6024,#6025,#6026,#6027,#6028,
#6029,#6030,#6031,#6032),.UNSPECIFIED.,.F.,.F.,(4,3,3,3,3,3,3,4),(-72.9560774123981,
-72.5099819795667,-71.516694555189,-70.5234071308114,-69.5301197064338,
-68.5368322820562,-67.5435448576786,-66.6728921052185),.UNSPECIFIED.);
#124=B_SPLINE_CURVE_WITH_KNOTS('',3,(#6037,#6038,#6039,#6040,#6041,#6042,
#6043,#6044,#6045,#6046,#6047,#6048,#6049,#6050,#6051,#6052,#6053,#6054,
#6055,#6056,#6057,#6058),.UNSPECIFIED.,.F.,.F.,(4,3,3,3,3,3,3,4),(64.1411894878524,
64.5636825845457,65.5569700089233,66.5502574333009,67.5435448576786,68.5368322820562,
69.5301197064338,70.424374795032),.UNSPECIFIED.);
#125=B_SPLINE_CURVE_WITH_KNOTS('',3,(#6059,#6060,#6061,#6062,#6063,#6064,
#6065,#6066,#6067,#6068,#6069,#6070,#6071,#6072,#6073,#6074,#6075,#6076,
#6077,#6078,#6079,#6080,#6081,#6082,#6083),.UNSPECIFIED.,.F.,.F.,(4,3,3,
3,3,3,3,3,4),(-66.6728921052185,-66.550257433301,-65.5569700089233,-64.5636825845457,
-63.5703951601681,-62.5771077357904,-61.5838203114128,-60.5905328870352,
-60.3897067980389),.UNSPECIFIED.);
#126=B_SPLINE_CURVE_WITH_KNOTS('',3,(#6088,#6089,#6090,#6091,#6092,#6093,
#6094,#6095,#6096,#6097,#6098,#6099,#6100,#6101,#6102,#6103,#6104,#6105,
#6106,#6107,#6108,#6109),.UNSPECIFIED.,.F.,.F.,(4,3,3,3,3,3,3,4),(57.8580041806728,
58.6039580382799,59.5972454626575,60.5905328870352,61.5838203114128,62.5771077357904,
63.570395160168,64.1411894878524),.UNSPECIFIED.);
#127=B_SPLINE_CURVE_WITH_KNOTS('',3,(#6110,#6111,#6112,#6113,#6114,#6115,
#6116,#6117,#6118,#6119,#6120,#6121,#6122,#6123,#6124,#6125,#6126,#6127,
#6128,#6129,#6130,#6131),.UNSPECIFIED.,.F.,.F.,(4,3,3,3,3,3,3,4),(-60.3897067980389,
-59.5972454626576,-58.6039580382799,-57.6106706139023,-56.6173831895247,
-55.624095765147,-54.6308083407694,-54.1065214908593),.UNSPECIFIED.);
#128=B_SPLINE_CURVE_WITH_KNOTS('',3,(#6136,#6137,#6138,#6139,#6140,#6141,
#6142,#6143,#6144,#6145,#6146,#6147,#6148,#6149,#6150,#6151,#6152,#6153,
#6154,#6155,#6156,#6157,#6158,#6159,#6160),.UNSPECIFIED.,.F.,.F.,(4,3,3,
3,3,3,3,3,4),(51.5748188734932,51.6509460676365,52.6442334920142,53.6375209163918,
54.6308083407694,55.624095765147,56.6173831895247,57.6106706139023,57.8580041806728),
 .UNSPECIFIED.);
#129=B_SPLINE_CURVE_WITH_KNOTS('',3,(#6161,#6162,#6163,#6164,#6165,#6166,
#6167,#6168,#6169,#6170,#6171,#6172,#6173,#6174,#6175,#6176,#6177,#6178,
#6179,#6180,#6181,#6182),.UNSPECIFIED.,.F.,.F.,(4,3,3,3,3,3,3,4),(-54.1065214908593,
-53.6375209163918,-52.6442334920142,-51.6509460676365,-50.6576586432589,
-49.6643712188813,-48.6710837945037,-47.8233361836797),.UNSPECIFIED.);
#130=B_SPLINE_CURVE_WITH_KNOTS('',3,(#6187,#6188,#6189,#6190,#6191,#6192,
#6193,#6194,#6195,#6196,#6197,#6198,#6199,#6200,#6201,#6202,#6203,#6204,
#6205,#6206,#6207,#6208),.UNSPECIFIED.,.F.,.F.,(4,3,3,3,3,3,3,4),(45.2916335663136,
45.6912215213708,46.6845089457484,47.677796370126,48.6710837945037,49.6643712188813,
50.6576586432589,51.5748188734932),.UNSPECIFIED.);
#131=B_SPLINE_CURVE_WITH_KNOTS('',3,(#6209,#6210,#6211,#6212,#6213,#6214,
#6215,#6216,#6217,#6218,#6219,#6220,#6221,#6222,#6223,#6224,#6225,#6226,
#6227,#6228,#6229,#6230,#6231,#6232,#6233),.UNSPECIFIED.,.F.,.F.,(4,3,3,
3,3,3,3,3,4),(-47.8233361836797,-47.677796370126,-46.6845089457484,-45.6912215213708,
-44.6979340969932,-43.7046466726155,-42.7113592482379,-41.7180718238603,
-41.5401508765001),.UNSPECIFIED.);
#132=B_SPLINE_CURVE_WITH_KNOTS('',3,(#6238,#6239,#6240,#6241,#6242,#6243,
#6244,#6245,#6246,#6247,#6248,#6249,#6250,#6251,#6252,#6253,#6254,#6255,
#6256,#6257,#6258,#6259),.UNSPECIFIED.,.F.,.F.,(4,3,3,3,3,3,3,4),(39.008448259134,
39.731496975105,40.7247843994827,41.7180718238603,42.7113592482379,43.7046466726155,
44.6979340969932,45.2916335663136),.UNSPECIFIED.);
#133=B_SPLINE_CURVE_WITH_KNOTS('',3,(#6260,#6261,#6262,#6263,#6264,#6265,
#6266,#6267,#6268,#6269,#6270,#6271,#6272,#6273,#6274,#6275,#6276,#6277,
#6278,#6279,#6280,#6281),.UNSPECIFIED.,.F.,.F.,(4,3,3,3,3,3,3,4),(-41.5401508765001,
-40.7247843994827,-39.731496975105,-38.7382095507274,-37.7449221263498,
-36.7516347019722,-35.7583472775945,-35.2569655693205),.UNSPECIFIED.);
#134=B_SPLINE_CURVE_WITH_KNOTS('',3,(#6286,#6287,#6288,#6289,#6290,#6291,
#6292,#6293,#6294,#6295,#6296,#6297,#6298,#6299,#6300,#6301,#6302,#6303,
#6304,#6305,#6306,#6307,#6308,#6309,#6310),.UNSPECIFIED.,.F.,.F.,(4,3,3,
3,3,3,3,3,4),(32.7252629519544,32.7784850044617,33.7717724288393,34.7650598532169,
35.7583472775945,36.7516347019722,37.7449221263498,38.7382095507274,39.008448259134),
 .UNSPECIFIED.);
#135=B_SPLINE_CURVE_WITH_KNOTS('',3,(#6311,#6312,#6313,#6314,#6315,#6316,
#6317,#6318,#6319,#6320,#6321,#6322,#6323,#6324,#6325,#6326,#6327,#6328,
#6329,#6330,#6331,#6332),.UNSPECIFIED.,.F.,.F.,(4,3,3,3,3,3,3,4),(-35.2569655693205,
-34.7650598532169,-33.7717724288393,-32.7784850044617,-31.785197580084,
-30.7919101557064,-29.7986227313288,-28.973780262141),.UNSPECIFIED.);
#136=B_SPLINE_CURVE_WITH_KNOTS('',3,(#6337,#6338,#6339,#6340,#6341,#6342,
#6343,#6344,#6345,#6346,#6347,#6348,#6349,#6350,#6351,#6352,#6353,#6354,
#6355,#6356,#6357,#6358),.UNSPECIFIED.,.F.,.F.,(4,3,3,3,3,3,3,4),(26.4420776447749,
26.8187604581959,27.8120478825735,28.8053353069512,29.7986227313288,30.7919101557064,
31.785197580084,32.7252629519544),.UNSPECIFIED.);
#137=B_SPLINE_CURVE_WITH_KNOTS('',3,(#6359,#6360,#6361,#6362,#6363,#6364,
#6365,#6366,#6367,#6368,#6369,#6370,#6371,#6372,#6373,#6374,#6375,#6376,
#6377,#6378,#6379,#6380,#6381,#6382,#6383),.UNSPECIFIED.,.F.,.F.,(4,3,3,
3,3,3,3,3,4),(-28.973780262141,-28.8053353069512,-27.8120478825735,-26.8187604581959,
-25.8254730338183,-24.8321856094406,-23.838898185063,-22.8456107606854,
-22.6905949549614),.UNSPECIFIED.);
#138=B_SPLINE_CURVE_WITH_KNOTS('',3,(#6388,#6389,#6390,#6391,#6392,#6393,
#6394,#6395,#6396,#6397,#6398,#6399,#6400,#6401,#6402,#6403,#6404,#6405,
#6406,#6407,#6408,#6409),.UNSPECIFIED.,.F.,.F.,(4,3,3,3,3,3,3,4),(20.1588923375953,
20.8590359119301,21.8523233363078,22.8456107606854,23.838898185063,24.8321856094406,
25.8254730338183,26.4420776447749),.UNSPECIFIED.);
#139=B_SPLINE_CURVE_WITH_KNOTS('',3,(#6410,#6411,#6412,#6413,#6414,#6415,
#6416,#6417,#6418,#6419,#6420,#6421,#6422,#6423,#6424,#6425,#6426,#6427,
#6428,#6429,#6430,#6431),.UNSPECIFIED.,.F.,.F.,(4,3,3,3,3,3,3,4),(-22.6905949549614,
-21.8523233363078,-20.8590359119301,-19.8657484875525,-18.8724610631749,
-17.8791736387973,-16.8858862144196,-16.4074096477818),.UNSPECIFIED.);
#140=B_SPLINE_CURVE_WITH_KNOTS('',3,(#6436,#6437,#6438,#6439,#6440,#6441,
#6442,#6443,#6444,#6445,#6446,#6447,#6448,#6449,#6450,#6451,#6452,#6453,
#6454,#6455,#6456,#6457,#6458,#6459,#6460),.UNSPECIFIED.,.F.,.F.,(4,3,3,
3,3,3,3,3,4),(13.8757070304157,13.9060239412868,14.8993113656644,15.892598790042,
16.8858862144196,17.8791736387973,18.8724610631749,19.8657484875525,20.1588923375953),
 .UNSPECIFIED.);
#141=B_SPLINE_CURVE_WITH_KNOTS('',3,(#6461,#6462,#6463,#6464,#6465,#6466,
#6467,#6468,#6469,#6470,#6471,#6472,#6473,#6474,#6475,#6476,#6477,#6478,
#6479,#6480,#6481,#6482),.UNSPECIFIED.,.F.,.F.,(4,3,3,3,3,3,3,4),(-16.4074096477818,
-15.892598790042,-14.8993113656644,-13.9060239412868,-12.9127365169091,
-11.9194490925315,-10.9261616681539,-10.1242243406022),.UNSPECIFIED.);
#142=B_SPLINE_CURVE_WITH_KNOTS('',3,(#6488,#6489,#6490,#6491,#6492,#6493,
#6494,#6495,#6496,#6497,#6498,#6499,#6500),.UNSPECIFIED.,.F.,.F.,(4,3,3,
3,4),(-3.84103903342261,-2.97986227313288,-1.98657484875525,-0.993287424377625,
0.),.UNSPECIFIED.);
#143=B_SPLINE_CURVE_WITH_KNOTS('',3,(#6503,#6504,#6505,#6506,#6507,#6508,
#6509,#6510,#6511,#6512,#6513,#6514,#6515,#6516,#6517,#6518,#6519,#6520,
#6521),.UNSPECIFIED.,.F.,.F.,(4,3,3,3,3,3,4),(2.00878279588941,2.97986227313288,
3.9731496975105,4.96643712188813,5.95972454626575,6.95301197064338,7.5925217232361),
 .UNSPECIFIED.);
#144=B_SPLINE_CURVE_WITH_KNOTS('',3,(#6527,#6528,#6529,#6530,#6531,#6532),
 .UNSPECIFIED.,.F.,.F.,(4,1,1,4),(97.3893722612836,98.2829301553797,99.2762175797573,
100.269505004135),.UNSPECIFIED.);
#145=B_SPLINE_CURVE_WITH_KNOTS('',3,(#6535,#6536,#6537,#6538,#6539,#6540,
#6541),.UNSPECIFIED.,.F.,.F.,(4,1,1,1,4),(97.3893722612836,97.8347704996129,
98.8280579239905,99.8213453483681,100.792424825612),.UNSPECIFIED.);
#146=B_SPLINE_CURVE_WITH_KNOTS('',3,(#6546,#6547,#6548,#6549,#6550,#6551,
#6552,#6553,#6554,#6555,#6556),.UNSPECIFIED.,.F.,.F.,(4,1,1,1,1,1,1,1,4),
(91.106186954104,91.3299181847363,92.323205609114,93.3164930334916,94.3097804578692,
95.3030678822468,96.2963553066245,97.2896427310021,97.3893722612836),
 .UNSPECIFIED.);
#147=B_SPLINE_CURVE_WITH_KNOTS('',3,(#6557,#6558,#6559,#6560,#6561,#6562,
#6563,#6564,#6565,#6566),.UNSPECIFIED.,.F.,.F.,(4,1,1,1,1,1,1,4),(91.106186954104,
91.8750459533471,92.8683333777248,93.8616208021024,94.85490822648,95.8481956508576,
96.8414830752353,97.3893722612836),.UNSPECIFIED.);
#148=B_SPLINE_CURVE_WITH_KNOTS('',3,(#6571,#6572,#6573,#6574,#6575,#6576,
#6577,#6578,#6579,#6580),.UNSPECIFIED.,.F.,.F.,(4,1,1,1,1,1,1,4),(84.8230016469244,
85.3701936384706,86.3634810628482,87.3567684872258,88.3500559116035,89.3433433359811,
90.3366307603587,91.106186954104),.UNSPECIFIED.);
#149=B_SPLINE_CURVE_WITH_KNOTS('',3,(#6581,#6582,#6583,#6584,#6585,#6586,
#6587,#6588,#6589,#6590,#6591),.UNSPECIFIED.,.F.,.F.,(4,1,1,1,1,1,1,1,4),
(84.8230016469244,84.9220339827037,85.9153214070814,86.908608831459,87.9018962558366,
88.8951836802142,89.8884711045919,90.8817585289695,91.106186954104),
 .UNSPECIFIED.);
#150=B_SPLINE_CURVE_WITH_KNOTS('',3,(#6596,#6597,#6598,#6599,#6600,#6601,
#6602,#6603,#6604,#6605),.UNSPECIFIED.,.F.,.F.,(4,1,1,1,1,1,1,4),(78.5398163397448,
79.4104690922048,80.4037565165825,81.3970439409601,82.3903313653377,83.3836187897153,
84.376906214093,84.8230016469244),.UNSPECIFIED.);
#151=B_SPLINE_CURVE_WITH_KNOTS('',3,(#6606,#6607,#6608,#6609,#6610,#6611,
#6612,#6613,#6614,#6615),.UNSPECIFIED.,.F.,.F.,(4,1,1,1,1,1,1,4),(78.5398163397448,
78.962309436438,79.9555968608156,80.9488842851932,81.9421717095709,82.9354591339485,
83.9287465583261,84.8230016469244),.UNSPECIFIED.);
#152=B_SPLINE_CURVE_WITH_KNOTS('',3,(#6620,#6621,#6622,#6623,#6624,#6625,
#6626,#6627,#6628,#6629,#6630),.UNSPECIFIED.,.F.,.F.,(4,1,1,1,1,1,1,1,4),
(72.2566310325652,72.4574571215614,73.4507445459391,74.4440319703167,75.4373193946943,
76.430606819072,77.4238942434496,78.4171816678272,78.5398163397448),
 .UNSPECIFIED.);
#153=B_SPLINE_CURVE_WITH_KNOTS('',3,(#6631,#6632,#6633,#6634,#6635,#6636,
#6637,#6638,#6639,#6640),.UNSPECIFIED.,.F.,.F.,(4,1,1,1,1,1,1,4),(72.2566310325652,
73.0025848901722,73.9958723145499,74.9891597389275,75.9824471633051,76.9757345876827,
77.9690220120604,78.5398163397448),.UNSPECIFIED.);
#154=B_SPLINE_CURVE_WITH_KNOTS('',3,(#6645,#6646,#6647,#6648,#6649,#6650,
#6651,#6652,#6653,#6654),.UNSPECIFIED.,.F.,.F.,(4,1,1,1,1,1,1,4),(65.9734457253856,
66.4977325752957,67.4910199996733,68.4843074240509,69.4775948484286,70.4708822728062,
71.4641696971838,72.2566310325652),.UNSPECIFIED.);
#155=B_SPLINE_CURVE_WITH_KNOTS('',3,(#6655,#6656,#6657,#6658,#6659,#6660,
#6661,#6662,#6663,#6664,#6665),.UNSPECIFIED.,.F.,.F.,(4,1,1,1,1,1,1,1,4),
(65.9734457253856,66.0495729195289,67.0428603439065,68.0361477682841,69.0294351926617,
70.0227226170393,71.016010041417,72.0092974657946,72.2566310325652),
 .UNSPECIFIED.);
#156=B_SPLINE_CURVE_WITH_KNOTS('',3,(#6670,#6671,#6672,#6673,#6674,#6675,
#6676,#6677,#6678,#6679),.UNSPECIFIED.,.F.,.F.,(4,1,1,1,1,1,1,4),(59.690260418206,
60.5380080290299,61.5312954534076,62.5245828777852,63.5178703021628,64.5111577265404,
65.5044451509181,65.9734457253856),.UNSPECIFIED.);
#157=B_SPLINE_CURVE_WITH_KNOTS('',3,(#6680,#6681,#6682,#6683,#6684,#6685,
#6686,#6687,#6688,#6689),.UNSPECIFIED.,.F.,.F.,(4,1,1,1,1,1,1,4),(59.690260418206,
60.0898483732631,61.0831357976407,62.0764232220183,63.069710646396,64.0629980707736,
65.0562854951512,65.9734457253856),.UNSPECIFIED.);
#158=B_SPLINE_CURVE_WITH_KNOTS('',3,(#6694,#6695,#6696,#6697,#6698,#6699,
#6700,#6701,#6702,#6703,#6704),.UNSPECIFIED.,.F.,.F.,(4,1,1,1,1,1,1,1,4),
(53.4070751110264,53.5849960583866,54.5782834827642,55.5715709071418,56.5648583315194,
57.5581457558971,58.5514331802747,59.5447206046523,59.690260418206),
 .UNSPECIFIED.);
#159=B_SPLINE_CURVE_WITH_KNOTS('',3,(#6705,#6706,#6707,#6708,#6709,#6710,
#6711,#6712,#6713,#6714),.UNSPECIFIED.,.F.,.F.,(4,1,1,1,1,1,1,4),(53.4070751110264,
54.1301238269973,55.123411251375,56.1166986757526,57.1099861001302,58.1032735245078,
59.0965609488855,59.690260418206),.UNSPECIFIED.);
#160=B_SPLINE_CURVE_WITH_KNOTS('',3,(#6719,#6720,#6721,#6722,#6723,#6724,
#6725,#6726,#6727,#6728),.UNSPECIFIED.,.F.,.F.,(4,1,1,1,1,1,1,4),(47.1238898038468,
47.6252715121208,48.6185589364984,49.6118463608761,50.6051337852537,51.5984212096313,
52.5917086340089,53.4070751110264),.UNSPECIFIED.);
#161=B_SPLINE_CURVE_WITH_KNOTS('',3,(#6729,#6730,#6731,#6732,#6733,#6734,
#6735,#6736,#6737,#6738,#6739),.UNSPECIFIED.,.F.,.F.,(4,1,1,1,1,1,1,1,4),
(47.1238898038468,47.177111856354,48.1703992807316,49.1636867051092,50.1569741294868,
51.1502615538645,52.1435489782421,53.1368364026197,53.4070751110264),
 .UNSPECIFIED.);
#162=B_SPLINE_CURVE_WITH_KNOTS('',3,(#6744,#6745,#6746,#6747,#6748,#6749,
#6750,#6751,#6752,#6753),.UNSPECIFIED.,.F.,.F.,(4,1,1,1,1,1,1,4),(40.8407044966673,
41.6655469658551,42.6588343902327,43.6521218146103,44.6454092389879,45.6386966633656,
46.6319840877432,47.1238898038468),.UNSPECIFIED.);
#163=B_SPLINE_CURVE_WITH_KNOTS('',3,(#6754,#6755,#6756,#6757,#6758,#6759,
#6760,#6761,#6762,#6763),.UNSPECIFIED.,.F.,.F.,(4,1,1,1,1,1,1,4),(40.8407044966672,
41.2173873100882,42.2106747344658,43.2039621588435,44.1972495832211,45.1905370075987,
46.1838244319763,47.1238898038468),.UNSPECIFIED.);
#164=B_SPLINE_CURVE_WITH_KNOTS('',3,(#6768,#6769,#6770,#6771,#6772,#6773,
#6774,#6775,#6776,#6777,#6778),.UNSPECIFIED.,.F.,.F.,(4,1,1,1,1,1,1,1,4),
(34.5575191894876,34.7125349952117,35.7058224195893,36.6991098439669,37.6923972683445,
38.6856846927222,39.6789721170998,40.6722595414774,40.8407044966673),
 .UNSPECIFIED.);
#165=B_SPLINE_CURVE_WITH_KNOTS('',3,(#6779,#6780,#6781,#6782,#6783,#6784,
#6785,#6786,#6787,#6788),.UNSPECIFIED.,.F.,.F.,(4,1,1,1,1,1,1,4),(34.5575191894876,
35.2576627638225,36.2509501882001,37.2442376125777,38.2375250369553,39.230812461333,
40.2240998857106,40.8407044966672),.UNSPECIFIED.);
#166=B_SPLINE_CURVE_WITH_KNOTS('',3,(#6793,#6794,#6795,#6796,#6797,#6798,
#6799,#6800,#6801,#6802),.UNSPECIFIED.,.F.,.F.,(4,1,1,1,1,1,1,4),(28.2743338823081,
28.7528104489459,29.7460978733235,30.7393852977012,31.7326727220788,32.7259601464564,
33.719247570834,34.5575191894876),.UNSPECIFIED.);
#167=B_SPLINE_CURVE_WITH_KNOTS('',3,(#6803,#6804,#6805,#6806,#6807,#6808,
#6809,#6810,#6811,#6812,#6813),.UNSPECIFIED.,.F.,.F.,(4,1,1,1,1,1,1,1,4),
(28.2743338823081,28.3046507931791,29.2979382175567,30.2912256419343,31.284513066312,
32.2778004906896,33.2710879150672,34.2643753394448,34.5575191894876),
 .UNSPECIFIED.);
#168=B_SPLINE_CURVE_WITH_KNOTS('',3,(#6818,#6819,#6820,#6821,#6822,#6823,
#6824,#6825,#6826,#6827),.UNSPECIFIED.,.F.,.F.,(4,1,1,1,1,1,1,4),(21.9911485751285,
22.7930859026802,23.7863733270578,24.7796607514354,25.772948175813,26.7662356001907,
27.7595230245683,28.2743338823081),.UNSPECIFIED.);
#169=B_SPLINE_CURVE_WITH_KNOTS('',3,(#6828,#6829,#6830,#6831,#6832,#6833,
#6834,#6835,#6836,#6837),.UNSPECIFIED.,.F.,.F.,(4,1,1,1,1,1,1,4),(21.9911485751285,
22.3449262469133,23.3382136712909,24.3315010956686,25.3247885200462,26.3180759444238,
27.3113633688014,28.2743338823081),.UNSPECIFIED.);
#170=B_SPLINE_CURVE_WITH_KNOTS('',3,(#6843,#6844,#6845,#6846,#6847),
 .UNSPECIFIED.,.F.,.F.,(4,1,4),(14.3986268518923,15.3919142762699,15.7079632679489),
 .UNSPECIFIED.);
#171=B_SPLINE_CURVE_WITH_KNOTS('',3,(#6850,#6851,#6852,#6853,#6854),
 .UNSPECIFIED.,.F.,.F.,(4,1,4),(13.8757070304157,14.8467865076592,15.7079632679489),
 .UNSPECIFIED.);
#172=B_SPLINE_CURVE_WITH_KNOTS('',3,(#6870,#6871,#6872,#6873,#6874,#6875,
#6876,#6877,#6878,#6879,#6880,#6881,#6882,#6883,#6884,#6885,#6886,#6887,
#6888,#6889,#6890,#6891,#6892,#6893,#6894,#6895,#6896,#6897,#6898,#6899,
#6900,#6901,#6902,#6903,#6904,#6905,#6906,#6907,#6908,#6909,#6910,#6911,
#6912,#6913,#6914,#6915,#6916,#6917,#6918,#6919,#6920,#6921,#6922,#6923,
#6924,#6925,#6926,#6927,#6928,#6929,#6930,#6931,#6932,#6933,#6934,#6935,
#6936,#6937,#6938,#6939,#6940,#6941,#6942,#6943,#6944,#6945,#6946,#6947,
#6948,#6949,#6950,#6951,#6952,#6953,#6954,#6955,#6956,#6957),
 .UNSPECIFIED.,.F.,.F.,(4,3,3,3,3,3,3,3,3,3,3,3,3,3,3,3,3,3,3,3,3,3,3,3,
3,3,3,3,3,4),(-0.474022601254863,-0.451447175941748,-0.428273788597453,
-0.423263601228443,-0.399553812376564,-0.380942280379475,-0.374677880834769,
-0.369385014064713,-0.345072731579855,-0.320408625751709,-0.295981811285532,
-0.286035429877351,-0.281943430084052,-0.25663161347214,-0.250661556399856,
-0.226280185736045,-0.201336866368482,-0.195740838705825,-0.190049717983688,
-0.164715513336959,-0.138863642602314,-0.112826574512041,-0.104606258115944,
-0.0991039006760492,-0.0951662220532652,-0.0685013567711513,-0.0418208873497662,
-0.0157306474362453,-0.00570411484459894,0.),.UNSPECIFIED.);
#173=B_SPLINE_CURVE_WITH_KNOTS('',3,(#6958,#6959,#6960,#6961,#6962,#6963,
#6964,#6965,#6966,#6967,#6968,#6969,#6970,#6971,#6972,#6973,#6974,#6975,
#6976,#6977,#6978,#6979,#6980,#6981,#6982,#6983,#6984,#6985,#6986,#6987,
#6988,#6989,#6990,#6991,#6992,#6993,#6994,#6995,#6996,#6997,#6998,#6999,
#7000,#7001,#7002,#7003,#7004,#7005,#7006,#7007,#7008,#7009,#7010,#7011,
#7012,#7013,#7014,#7015,#7016,#7017,#7018,#7019,#7020,#7021,#7022,#7023,
#7024,#7025,#7026,#7027,#7028,#7029,#7030,#7031,#7032,#7033,#7034,#7035,
#7036,#7037,#7038,#7039,#7040,#7041,#7042,#7043,#7044,#7045,#7046,#7047,
#7048),.UNSPECIFIED.,.F.,.F.,(4,3,3,3,3,3,3,3,3,3,3,3,3,3,3,3,3,3,3,3,3,
3,3,3,3,3,3,3,3,3,4),(-0.472119585381858,-0.44577460207496,-0.418546032433648,
-0.413165251718511,-0.407785600416182,-0.381445798916785,-0.362258329670245,
-0.355369245757151,-0.350800797401284,-0.32505688895012,-0.29982216759042,
-0.275104705363238,-0.267797971074288,-0.262198851065717,-0.258325702856778,
-0.233810691839444,-0.227946044944466,-0.20299171843274,-0.178209571955242,
-0.172135092187495,-0.168338367316375,-0.143931769623782,-0.119575292467824,
-0.0956609071136006,-0.085488047709299,-0.0813672853715775,-0.0579089720113479,
-0.0348587622710651,-0.0125514055137675,-0.00473454661276074,0.),
 .UNSPECIFIED.);
#174=B_SPLINE_CURVE_WITH_KNOTS('',3,(#7050,#7051,#7052,#7053,#7054,#7055,
#7056,#7057,#7058,#7059,#7060),.UNSPECIFIED.,.F.,.F.,(4,1,1,1,1,1,1,1,4),
(15.7079632679489,15.8400739320368,16.8333613564144,17.826648780792,18.8199362051697,
19.8132236295473,20.8065110539249,21.7997984783025,21.9911485751285),
 .UNSPECIFIED.);
#175=B_SPLINE_CURVE_WITH_KNOTS('',3,(#7061,#7062,#7063,#7064,#7065,#7066,
#7067,#7068,#7069,#7070),.UNSPECIFIED.,.F.,.F.,(4,1,1,1,1,1,1,4),(15.7079632679489,
16.3852017006476,17.3784891250252,18.3717765494028,19.3650639737804,20.3583513981581,
21.3516388225357,21.9911485751285),.UNSPECIFIED.);
#176=B_SPLINE_CURVE_WITH_KNOTS('',3,(#7439,#7440,#7441,#7442,#7443,#7444,
#7445,#7446,#7447,#7448,#7449,#7450,#7451,#7452,#7453,#7454,#7455,#7456,
#7457,#7458,#7459,#7460,#7461,#7462,#7463,#7464,#7465,#7466,#7467,#7468,
#7469,#7470,#7471,#7472,#7473,#7474,#7475,#7476,#7477,#7478,#7479,#7480,
#7481,#7482,#7483,#7484,#7485,#7486,#7487,#7488,#7489,#7490,#7491,#7492,
#7493,#7494,#7495,#7496,#7497,#7498,#7499,#7500,#7501,#7502,#7503,#7504,
#7505,#7506,#7507,#7508,#7509,#7510,#7511,#7512,#7513,#7514,#7515,#7516,
#7517,#7518,#7519,#7520,#7521,#7522,#7523,#7524,#7525,#7526,#7527,#7528,
#7529),.UNSPECIFIED.,.F.,.F.,(4,3,3,3,3,3,3,3,3,3,3,3,3,3,3,3,3,3,3,3,3,
3,3,3,3,3,3,3,3,3,4),(0.,0.0222952799330679,0.0452097945174155,0.0673981627831887,
0.0771055738994644,0.0835930447079554,0.0876186285667832,0.111617824771073,
0.135994295972414,0.157674907140211,0.166068223331749,0.170734301358664,
0.174713848522195,0.199787338407663,0.222716740643601,0.247155303462719,
0.256497618171605,0.26074445324338,0.264505632816036,0.289747052399726,
0.315274931436527,0.341051827552776,0.351578296876228,0.358096975465089,
0.385181978970206,0.405495731599044,0.412526368251741,0.41821220868089,
0.444807422955841,0.466436989485556,0.472119585381884),.UNSPECIFIED.);
#177=B_SPLINE_CURVE_WITH_KNOTS('',3,(#7530,#7531,#7532,#7533,#7534,#7535,
#7536,#7537,#7538,#7539,#7540,#7541,#7542,#7543,#7544,#7545,#7546,#7547,
#7548,#7549,#7550,#7551,#7552,#7553,#7554),.UNSPECIFIED.,.F.,.F.,(4,3,3,
3,3,3,3,3,4),(-10.1242243406022,-9.93287424377626,-8.93958681939863,-7.946299395021,
-6.95301197064338,-5.95972454626575,-4.96643712188813,-3.9731496975105,
-3.84103903342261),.UNSPECIFIED.);
#178=B_SPLINE_CURVE_WITH_KNOTS('',3,(#7923,#7924,#7925,#7926,#7927,#7928,
#7929,#7930,#7931,#7932,#7933,#7934,#7935,#7936,#7937,#7938,#7939,#7940,
#7941,#7942,#7943,#7944),.UNSPECIFIED.,.F.,.F.,(4,3,3,3,3,3,3,4),(7.5925217232361,
7.946299395021,8.93958681939863,9.93287424377626,10.9261616681539,11.9194490925315,
12.9127365169091,13.8757070304157),.UNSPECIFIED.);
#179=B_SPLINE_CURVE_WITH_KNOTS('',3,(#7945,#7946,#7947,#7948,#7949,#7950,
#7951,#7952,#7953,#7954,#7955,#7956,#7957,#7958,#7959,#7960,#7961,#7962,
#7963,#7964,#7965,#7966,#7967,#7968,#7969,#7970,#7971,#7972,#7973,#7974,
#7975,#7976,#7977,#7978,#7979,#7980,#7981,#7982,#7983,#7984,#7985,#7986,
#7987,#7988,#7989,#7990,#7991,#7992,#7993,#7994,#7995,#7996,#7997,#7998,
#7999,#8000,#8001,#8002,#8003,#8004,#8005,#8006,#8007,#8008,#8009,#8010,
#8011,#8012,#8013,#8014,#8015,#8016,#8017,#8018,#8019,#8020,#8021,#8022,
#8023,#8024,#8025,#8026,#8027,#8028,#8029,#8030,#8031,#8032,#8033,#8034,
#8035),.UNSPECIFIED.,.F.,.F.,(4,3,3,3,3,3,3,3,3,3,3,3,3,3,3,3,3,3,3,3,3,
3,3,3,3,3,3,3,3,3,4),(0.,0.0259340516234306,0.053368683612658,0.077373986603232,
0.0889343286239471,0.0962033318415016,0.100907449948929,0.126912276034724,
0.152761874310813,0.175924182617423,0.186282013485412,0.191317187370802,
0.195407257095002,0.220409182316126,0.24541110753725,0.270731737634532,
0.279140838448213,0.283746551506711,0.287674236654677,0.312284916819144,
0.336926589907284,0.36117345873944,0.370907512364279,0.37536825313801,0.399043742409906,
0.416600959495802,0.422836588536135,0.427178020979947,0.449946450206982,
0.46927261075349,0.474022601254828),.UNSPECIFIED.);
#180=B_SPLINE_CURVE_WITH_KNOTS('',3,(#8038,#8039,#8040,#8041,#8042,#8043,
#8044,#8045,#8046,#8047,#8048,#8049,#8050,#8051,#8052,#8053,#8054,#8055,
#8056,#8057,#8058,#8059,#8060,#8061,#8062,#8063,#8064,#8065,#8066,#8067,
#8068,#8069,#8070,#8071,#8072,#8073,#8074,#8075,#8076,#8077,#8078,#8079,
#8080,#8081,#8082,#8083,#8084,#8085,#8086,#8087,#8088,#8089,#8090,#8091,
#8092,#8093,#8094,#8095,#8096,#8097,#8098,#8099,#8100,#8101,#8102,#8103,
#8104,#8105,#8106,#8107,#8108,#8109,#8110,#8111,#8112,#8113,#8114,#8115,
#8116,#8117,#8118,#8119,#8120,#8121,#8122,#8123,#8124,#8125),
 .UNSPECIFIED.,.F.,.F.,(4,3,3,3,3,3,3,3,3,3,3,3,3,3,3,3,3,3,3,3,3,3,3,3,
3,3,3,3,3,4),(-0.474022601254861,-0.451447164140717,-0.428273767136123,
-0.423263579545402,-0.399553781970167,-0.380942253773878,-0.374677666863019,
-0.369384940914017,-0.34507264958386,-0.320408545071338,-0.295981736703132,
-0.286035177673738,-0.281943454875479,-0.256631639402781,-0.250661556399858,
-0.226280193777327,-0.201336878994557,-0.195740857792063,-0.190049717577327,
-0.164715519332485,-0.138863651462101,-0.112826583581217,-0.104606275686148,
-0.0991040164814279,-0.0951663280195914,-0.0685014645407558,-0.0418209943289155,
-0.0157307547741264,-0.00570411484459894,0.),.UNSPECIFIED.);
#181=B_SPLINE_CURVE_WITH_KNOTS('',3,(#8126,#8127,#8128,#8129,#8130,#8131,
#8132,#8133,#8134,#8135,#8136,#8137,#8138,#8139,#8140,#8141,#8142,#8143,
#8144,#8145,#8146,#8147,#8148,#8149,#8150,#8151,#8152,#8153,#8154,#8155,
#8156,#8157,#8158,#8159,#8160,#8161,#8162,#8163,#8164,#8165,#8166,#8167,
#8168,#8169,#8170,#8171,#8172,#8173,#8174,#8175,#8176,#8177,#8178,#8179,
#8180,#8181,#8182,#8183,#8184,#8185,#8186,#8187,#8188,#8189,#8190,#8191,
#8192,#8193,#8194,#8195,#8196,#8197,#8198,#8199,#8200,#8201,#8202,#8203,
#8204,#8205,#8206,#8207,#8208,#8209,#8210,#8211,#8212,#8213,#8214,#8215,
#8216),.UNSPECIFIED.,.F.,.F.,(4,3,3,3,3,3,3,3,3,3,3,3,3,3,3,3,3,3,3,3,3,
3,3,3,3,3,3,3,3,3,4),(-0.472119585381859,-0.445774611141889,-0.41854604036721,
-0.413165258086392,-0.407785602596351,-0.381445800212958,-0.362258330804396,
-0.355369248347035,-0.350800798519935,-0.325056888599833,-0.299822162923893,
-0.275104697414975,-0.267797956175982,-0.262198802438247,-0.258325632397721,
-0.233810617962332,-0.227946044944459,-0.202991718039396,-0.178209571611067,
-0.172135088823669,-0.168338364331946,-0.143931766984762,-0.119575288853072,
-0.095660898841475,-0.0854880154494424,-0.081367290874658,-0.057908974539604,
-0.0348587585203453,-0.0125513914292997,-0.00473454661275771,0.),
 .UNSPECIFIED.);
#182=B_SPLINE_CURVE_WITH_KNOTS('',3,(#8218,#8219,#8220,#8221,#8222,#8223,
#8224,#8225,#8226,#8227,#8228),.UNSPECIFIED.,.F.,.F.,(4,1,1,1,1,1,1,1,4),
(15.7079632679489,15.8400739320368,16.8333613564144,17.826648780792,18.8199362051697,
19.8132236295473,20.8065110539249,21.7997984783025,21.9911485751285),
 .UNSPECIFIED.);
#183=B_SPLINE_CURVE_WITH_KNOTS('',3,(#8229,#8230,#8231,#8232,#8233,#8234,
#8235,#8236,#8237,#8238),.UNSPECIFIED.,.F.,.F.,(4,1,1,1,1,1,1,4),(15.7079632679489,
16.3852017006476,17.3784891250252,18.3717765494028,19.3650639737804,20.3583513981581,
21.3516388225357,21.9911485751285),.UNSPECIFIED.);
#184=B_SPLINE_CURVE_WITH_KNOTS('',3,(#8607,#8608,#8609,#8610,#8611,#8612,
#8613,#8614,#8615,#8616,#8617,#8618,#8619,#8620,#8621,#8622,#8623,#8624,
#8625,#8626,#8627,#8628,#8629,#8630,#8631,#8632,#8633,#8634,#8635,#8636,
#8637,#8638,#8639,#8640,#8641,#8642,#8643,#8644,#8645,#8646,#8647,#8648,
#8649,#8650,#8651,#8652,#8653,#8654,#8655,#8656,#8657,#8658,#8659,#8660,
#8661,#8662,#8663,#8664,#8665,#8666,#8667,#8668,#8669,#8670,#8671,#8672,
#8673,#8674,#8675,#8676,#8677,#8678,#8679,#8680,#8681,#8682,#8683,#8684,
#8685,#8686,#8687,#8688,#8689,#8690,#8691,#8692,#8693,#8694,#8695,#8696,
#8697),.UNSPECIFIED.,.F.,.F.,(4,3,3,3,3,3,3,3,3,3,3,3,3,3,3,3,3,3,3,3,3,
3,3,3,3,3,3,3,3,3,4),(0.,0.0222952651137365,0.0452097666204725,0.0673981383733636,
0.0771055510152534,0.08359300396032,0.0876186186491862,0.111617805012605,
0.135994272391414,0.157674889454461,0.166068200672421,0.170733863879555,
0.174713775562166,0.199787267862165,0.222716740643601,0.247155310880047,
0.256497643401853,0.260744554886893,0.264505835070973,0.289747229372796,
0.315275115498424,0.341052012614648,0.351578318626618,0.358096973365246,
0.385181977395323,0.405495730417882,0.412526370937833,0.418212210551543,
0.444807425042136,0.466436989485556,0.472119585381884),.UNSPECIFIED.);
#185=B_SPLINE_CURVE_WITH_KNOTS('',3,(#8698,#8699,#8700,#8701,#8702,#8703,
#8704,#8705,#8706,#8707,#8708,#8709,#8710,#8711,#8712,#8713,#8714,#8715,
#8716,#8717,#8718,#8719,#8720,#8721,#8722),.UNSPECIFIED.,.F.,.F.,(4,3,3,
3,3,3,3,3,4),(-10.1242243406022,-9.93287424377626,-8.93958681939863,-7.946299395021,
-6.95301197064338,-5.95972454626575,-4.96643712188813,-3.9731496975105,
-3.84103903342261),.UNSPECIFIED.);
#186=B_SPLINE_CURVE_WITH_KNOTS('',3,(#9091,#9092,#9093,#9094,#9095,#9096,
#9097,#9098,#9099,#9100,#9101,#9102,#9103,#9104,#9105,#9106,#9107,#9108,
#9109,#9110,#9111,#9112),.UNSPECIFIED.,.F.,.F.,(4,3,3,3,3,3,3,4),(7.5925217232361,
7.946299395021,8.93958681939863,9.93287424377626,10.9261616681539,11.9194490925315,
12.9127365169091,13.8757070304157),.UNSPECIFIED.);
#187=B_SPLINE_CURVE_WITH_KNOTS('',3,(#9113,#9114,#9115,#9116,#9117,#9118,
#9119,#9120,#9121,#9122,#9123,#9124,#9125,#9126,#9127,#9128,#9129,#9130,
#9131,#9132,#9133,#9134,#9135,#9136,#9137,#9138,#9139,#9140,#9141,#9142,
#9143,#9144,#9145,#9146,#9147,#9148,#9149,#9150,#9151,#9152,#9153,#9154,
#9155,#9156,#9157,#9158,#9159,#9160,#9161,#9162,#9163,#9164,#9165,#9166,
#9167,#9168,#9169,#9170,#9171,#9172,#9173,#9174,#9175,#9176,#9177,#9178,
#9179,#9180,#9181,#9182,#9183,#9184,#9185,#9186,#9187,#9188,#9189,#9190,
#9191,#9192,#9193,#9194,#9195,#9196,#9197,#9198,#9199,#9200,#9201,#9202,
#9203),.UNSPECIFIED.,.F.,.F.,(4,3,3,3,3,3,3,3,3,3,3,3,3,3,3,3,3,3,3,3,3,
3,3,3,3,3,3,3,3,3,4),(0.,0.0259340620084641,0.0533686926995623,0.0773739945542733,
0.0889343332539756,0.0962033282984184,0.100907449205028,0.126912275229181,
0.152761870371554,0.175924179662978,0.186282012481782,0.191317190306999,
0.195407257920147,0.220409182728698,0.24541110753725,0.270731737938341,
0.279140836043757,0.28374654253246,0.287674221295602,0.312284901472548,
0.336926574293682,0.36117344014891,0.370907500046057,0.37536825002033,0.399043735515415,
0.416600954324934,0.422836562863072,0.427177984470413,0.449946407582691,
0.46927261075349,0.474022601254827),.UNSPECIFIED.);
#318=SHAPE_REPRESENTATION_RELATIONSHIP('SRR','None',#13836,#324);
#324=ADVANCED_BREP_SHAPE_REPRESENTATION('',(#336),#13796);
#330=STYLED_ITEM('',(#13879),#336);
#336=MANIFOLD_SOLID_BREP('Body1',#3695);
#355=FACE_BOUND('',#740,.T.);
#356=FACE_BOUND('',#741,.T.);
#357=FACE_BOUND('',#742,.T.);
#358=FACE_BOUND('',#743,.T.);
#359=FACE_BOUND('',#747,.T.);
#360=FACE_BOUND('',#749,.T.);
#373=PLANE('',#3870);
#374=PLANE('',#3874);
#375=PLANE('',#3875);
#376=PLANE('',#3878);
#377=PLANE('',#3881);
#378=PLANE('',#3882);
#379=PLANE('',#3883);
#380=PLANE('',#3887);
#381=PLANE('',#3891);
#382=PLANE('',#3895);
#383=PLANE('',#3902);
#384=PLANE('',#3906);
#385=PLANE('',#3907);
#386=PLANE('',#3908);
#387=PLANE('',#3909);
#388=PLANE('',#3910);
#389=PLANE('',#3914);
#390=PLANE('',#3918);
#391=PLANE('',#3919);
#392=PLANE('',#3920);
#393=PLANE('',#3921);
#394=PLANE('',#3922);
#395=PLANE('',#3923);
#396=PLANE('',#3924);
#433=FACE_OUTER_BOUND('',#648,.T.);
#434=FACE_OUTER_BOUND('',#649,.T.);
#435=FACE_OUTER_BOUND('',#650,.T.);
#436=FACE_OUTER_BOUND('',#651,.T.);
#437=FACE_OUTER_BOUND('',#652,.T.);
#438=FACE_OUTER_BOUND('',#653,.T.);
#439=FACE_OUTER_BOUND('',#654,.T.);
#440=FACE_OUTER_BOUND('',#655,.T.);
#441=FACE_OUTER_BOUND('',#656,.T.);
#442=FACE_OUTER_BOUND('',#657,.T.);
#443=FACE_OUTER_BOUND('',#658,.T.);
#444=FACE_OUTER_BOUND('',#659,.T.);
#445=FACE_OUTER_BOUND('',#660,.T.);
#446=FACE_OUTER_BOUND('',#661,.T.);
#447=FACE_OUTER_BOUND('',#662,.T.);
#448=FACE_OUTER_BOUND('',#663,.T.);
#449=FACE_OUTER_BOUND('',#664,.T.);
#450=FACE_OUTER_BOUND('',#665,.T.);
#451=FACE_OUTER_BOUND('',#666,.T.);
#452=FACE_OUTER_BOUND('',#667,.T.);
#453=FACE_OUTER_BOUND('',#668,.T.);
#454=FACE_OUTER_BOUND('',#669,.T.);
#455=FACE_OUTER_BOUND('',#670,.T.);
#456=FACE_OUTER_BOUND('',#671,.T.);
#457=FACE_OUTER_BOUND('',#672,.T.);
#458=FACE_OUTER_BOUND('',#673,.T.);
#459=FACE_OUTER_BOUND('',#674,.T.);
#460=FACE_OUTER_BOUND('',#675,.T.);
#461=FACE_OUTER_BOUND('',#676,.T.);
#462=FACE_OUTER_BOUND('',#677,.T.);
#463=FACE_OUTER_BOUND('',#678,.T.);
#464=FACE_OUTER_BOUND('',#679,.T.);
#465=FACE_OUTER_BOUND('',#680,.T.);
#466=FACE_OUTER_BOUND('',#681,.T.);
#467=FACE_OUTER_BOUND('',#682,.T.);
#468=FACE_OUTER_BOUND('',#683,.T.);
#469=FACE_OUTER_BOUND('',#684,.T.);
#470=FACE_OUTER_BOUND('',#685,.T.);
#471=FACE_OUTER_BOUND('',#686,.T.);
#472=FACE_OUTER_BOUND('',#687,.T.);
#473=FACE_OUTER_BOUND('',#688,.T.);
#474=FACE_OUTER_BOUND('',#689,.T.);
#475=FACE_OUTER_BOUND('',#690,.T.);
#476=FACE_OUTER_BOUND('',#691,.T.);
#477=FACE_OUTER_BOUND('',#692,.T.);
#478=FACE_OUTER_BOUND('',#693,.T.);
#479=FACE_OUTER_BOUND('',#694,.T.);
#480=FACE_OUTER_BOUND('',#695,.T.);
#481=FACE_OUTER_BOUND('',#696,.T.);
#482=FACE_OUTER_BOUND('',#697,.T.);
#483=FACE_OUTER_BOUND('',#698,.T.);
#484=FACE_OUTER_BOUND('',#699,.T.);
#485=FACE_OUTER_BOUND('',#700,.T.);
#486=FACE_OUTER_BOUND('',#701,.T.);
#487=FACE_OUTER_BOUND('',#702,.T.);
#488=FACE_OUTER_BOUND('',#703,.T.);
#489=FACE_OUTER_BOUND('',#704,.T.);
#490=FACE_OUTER_BOUND('',#705,.T.);
#491=FACE_OUTER_BOUND('',#706,.T.);
#492=FACE_OUTER_BOUND('',#707,.T.);
#493=FACE_OUTER_BOUND('',#708,.T.);
#494=FACE_OUTER_BOUND('',#709,.T.);
#495=FACE_OUTER_BOUND('',#710,.T.);
#496=FACE_OUTER_BOUND('',#711,.T.);
#497=FACE_OUTER_BOUND('',#712,.T.);
#498=FACE_OUTER_BOUND('',#713,.T.);
#499=FACE_OUTER_BOUND('',#714,.T.);
#500=FACE_OUTER_BOUND('',#715,.T.);
#501=FACE_OUTER_BOUND('',#716,.T.);
#502=FACE_OUTER_BOUND('',#717,.T.);
#503=FACE_OUTER_BOUND('',#718,.T.);
#504=FACE_OUTER_BOUND('',#719,.T.);
#505=FACE_OUTER_BOUND('',#720,.T.);
#506=FACE_OUTER_BOUND('',#721,.T.);
#507=FACE_OUTER_BOUND('',#722,.T.);
#508=FACE_OUTER_BOUND('',#723,.T.);
#509=FACE_OUTER_BOUND('',#724,.T.);
#510=FACE_OUTER_BOUND('',#725,.T.);
#511=FACE_OUTER_BOUND('',#726,.T.);
#512=FACE_OUTER_BOUND('',#727,.T.);
#513=FACE_OUTER_BOUND('',#728,.T.);
#514=FACE_OUTER_BOUND('',#729,.T.);
#515=FACE_OUTER_BOUND('',#730,.T.);
#516=FACE_OUTER_BOUND('',#731,.T.);
#517=FACE_OUTER_BOUND('',#732,.T.);
#518=FACE_OUTER_BOUND('',#733,.T.);
#519=FACE_OUTER_BOUND('',#734,.T.);
#520=FACE_OUTER_BOUND('',#735,.T.);
#521=FACE_OUTER_BOUND('',#736,.T.);
#522=FACE_OUTER_BOUND('',#737,.T.);
#523=FACE_OUTER_BOUND('',#738,.T.);
#524=FACE_OUTER_BOUND('',#739,.T.);
#525=FACE_OUTER_BOUND('',#744,.T.);
#526=FACE_OUTER_BOUND('',#745,.T.);
#527=FACE_OUTER_BOUND('',#746,.T.);
#528=FACE_OUTER_BOUND('',#748,.T.);
#648=EDGE_LOOP('',(#2337,#2338,#2339,#2340,#2341,#2342,#2343,#2344));
#649=EDGE_LOOP('',(#2345,#2346,#2347,#2348));
#650=EDGE_LOOP('',(#2349,#2350,#2351,#2352));
#651=EDGE_LOOP('',(#2353,#2354,#2355,#2356));
#652=EDGE_LOOP('',(#2357,#2358,#2359,#2360));
#653=EDGE_LOOP('',(#2361,#2362,#2363,#2364));
#654=EDGE_LOOP('',(#2365,#2366,#2367,#2368));
#655=EDGE_LOOP('',(#2369,#2370,#2371,#2372));
#656=EDGE_LOOP('',(#2373,#2374,#2375,#2376));
#657=EDGE_LOOP('',(#2377,#2378,#2379,#2380));
#658=EDGE_LOOP('',(#2381,#2382,#2383,#2384));
#659=EDGE_LOOP('',(#2385,#2386,#2387,#2388));
#660=EDGE_LOOP('',(#2389,#2390,#2391,#2392));
#661=EDGE_LOOP('',(#2393,#2394,#2395,#2396));
#662=EDGE_LOOP('',(#2397,#2398,#2399,#2400));
#663=EDGE_LOOP('',(#2401,#2402,#2403,#2404));
#664=EDGE_LOOP('',(#2405,#2406,#2407,#2408));
#665=EDGE_LOOP('',(#2409,#2410,#2411,#2412));
#666=EDGE_LOOP('',(#2413,#2414,#2415,#2416));
#667=EDGE_LOOP('',(#2417,#2418,#2419,#2420));
#668=EDGE_LOOP('',(#2421,#2422,#2423,#2424));
#669=EDGE_LOOP('',(#2425,#2426,#2427,#2428));
#670=EDGE_LOOP('',(#2429,#2430,#2431,#2432));
#671=EDGE_LOOP('',(#2433,#2434,#2435,#2436));
#672=EDGE_LOOP('',(#2437,#2438,#2439,#2440));
#673=EDGE_LOOP('',(#2441,#2442,#2443,#2444));
#674=EDGE_LOOP('',(#2445,#2446,#2447,#2448));
#675=EDGE_LOOP('',(#2449,#2450,#2451,#2452,#2453,#2454,#2455,#2456));
#676=EDGE_LOOP('',(#2457,#2458,#2459,#2460));
#677=EDGE_LOOP('',(#2461,#2462,#2463,#2464));
#678=EDGE_LOOP('',(#2465,#2466,#2467,#2468));
#679=EDGE_LOOP('',(#2469,#2470,#2471,#2472));
#680=EDGE_LOOP('',(#2473,#2474,#2475,#2476));
#681=EDGE_LOOP('',(#2477,#2478,#2479,#2480));
#682=EDGE_LOOP('',(#2481,#2482,#2483,#2484));
#683=EDGE_LOOP('',(#2485,#2486,#2487,#2488));
#684=EDGE_LOOP('',(#2489,#2490,#2491,#2492));
#685=EDGE_LOOP('',(#2493,#2494,#2495,#2496));
#686=EDGE_LOOP('',(#2497,#2498,#2499,#2500));
#687=EDGE_LOOP('',(#2501,#2502,#2503,#2504));
#688=EDGE_LOOP('',(#2505,#2506,#2507,#2508));
#689=EDGE_LOOP('',(#2509,#2510,#2511,#2512));
#690=EDGE_LOOP('',(#2513,#2514,#2515,#2516));
#691=EDGE_LOOP('',(#2517,#2518,#2519,#2520));
#692=EDGE_LOOP('',(#2521,#2522,#2523,#2524));
#693=EDGE_LOOP('',(#2525,#2526,#2527,#2528));
#694=EDGE_LOOP('',(#2529,#2530,#2531,#2532));
#695=EDGE_LOOP('',(#2533,#2534,#2535,#2536));
#696=EDGE_LOOP('',(#2537,#2538,#2539,#2540));
#697=EDGE_LOOP('',(#2541,#2542,#2543,#2544));
#698=EDGE_LOOP('',(#2545,#2546,#2547,#2548));
#699=EDGE_LOOP('',(#2549,#2550,#2551,#2552));
#700=EDGE_LOOP('',(#2553,#2554,#2555,#2556));
#701=EDGE_LOOP('',(#2557,#2558,#2559,#2560));
#702=EDGE_LOOP('',(#2561,#2562,#2563,#2564));
#703=EDGE_LOOP('',(#2565));
#704=EDGE_LOOP('',(#2566,#2567,#2568,#2569));
#705=EDGE_LOOP('',(#2570));
#706=EDGE_LOOP('',(#2571,#2572,#2573,#2574));
#707=EDGE_LOOP('',(#2575,#2576,#2577,#2578));
#708=EDGE_LOOP('',(#2579,#2580,#2581,#2582,#2583,#2584,#2585,#2586,#2587,
#2588,#2589,#2590,#2591,#2592,#2593,#2594,#2595,#2596,#2597,#2598,#2599,
#2600,#2601,#2602,#2603,#2604,#2605,#2606,#2607,#2608,#2609,#2610));
#709=EDGE_LOOP('',(#2611,#2612,#2613,#2614,#2615,#2616,#2617,#2618,#2619,
#2620,#2621,#2622,#2623,#2624,#2625,#2626,#2627,#2628,#2629,#2630,#2631,
#2632,#2633,#2634,#2635,#2636,#2637,#2638,#2639,#2640,#2641));
#710=EDGE_LOOP('',(#2642,#2643,#2644,#2645));
#711=EDGE_LOOP('',(#2646,#2647,#2648,#2649));
#712=EDGE_LOOP('',(#2650,#2651,#2652,#2653));
#713=EDGE_LOOP('',(#2654,#2655,#2656,#2657,#2658,#2659,#2660,#2661,#2662,
#2663,#2664,#2665,#2666,#2667,#2668,#2669,#2670,#2671,#2672,#2673,#2674,
#2675,#2676,#2677,#2678,#2679,#2680,#2681,#2682,#2683,#2684,#2685));
#714=EDGE_LOOP('',(#2686,#2687,#2688,#2689,#2690,#2691,#2692,#2693,#2694,
#2695,#2696,#2697,#2698,#2699,#2700,#2701,#2702,#2703,#2704,#2705,#2706,
#2707,#2708,#2709,#2710,#2711,#2712,#2713,#2714,#2715,#2716));
#715=EDGE_LOOP('',(#2717,#2718,#2719,#2720));
#716=EDGE_LOOP('',(#2721));
#717=EDGE_LOOP('',(#2722));
#718=EDGE_LOOP('',(#2723,#2724,#2725,#2726));
#719=EDGE_LOOP('',(#2727,#2728,#2729,#2730));
#720=EDGE_LOOP('',(#2731,#2732,#2733,#2734));
#721=EDGE_LOOP('',(#2735,#2736,#2737,#2738));
#722=EDGE_LOOP('',(#2739,#2740,#2741,#2742));
#723=EDGE_LOOP('',(#2743,#2744,#2745,#2746));
#724=EDGE_LOOP('',(#2747,#2748,#2749,#2750));
#725=EDGE_LOOP('',(#2751,#2752,#2753,#2754));
#726=EDGE_LOOP('',(#2755,#2756,#2757,#2758));
#727=EDGE_LOOP('',(#2759,#2760,#2761,#2762));
#728=EDGE_LOOP('',(#2763,#2764,#2765,#2766));
#729=EDGE_LOOP('',(#2767,#2768,#2769,#2770));
#730=EDGE_LOOP('',(#2771,#2772,#2773,#2774));
#731=EDGE_LOOP('',(#2775,#2776,#2777,#2778));
#732=EDGE_LOOP('',(#2779,#2780,#2781,#2782));
#733=EDGE_LOOP('',(#2783,#2784,#2785,#2786));
#734=EDGE_LOOP('',(#2787,#2788,#2789,#2790));
#735=EDGE_LOOP('',(#2791,#2792,#2793,#2794));
#736=EDGE_LOOP('',(#2795,#2796,#2797,#2798));
#737=EDGE_LOOP('',(#2799,#2800,#2801,#2802));
#738=EDGE_LOOP('',(#2803,#2804,#2805,#2806));
#739=EDGE_LOOP('',(#2807,#2808,#2809,#2810));
#740=EDGE_LOOP('',(#2811));
#741=EDGE_LOOP('',(#2812));
#742=EDGE_LOOP('',(#2813,#2814,#2815,#2816));
#743=EDGE_LOOP('',(#2817,#2818,#2819,#2820));
#744=EDGE_LOOP('',(#2821,#2822,#2823,#2824));
#745=EDGE_LOOP('',(#2825,#2826,#2827,#2828));
#746=EDGE_LOOP('',(#2829,#2830,#2831,#2832,#2833,#2834,#2835,#2836,#2837,
#2838,#2839,#2840,#2841,#2842,#2843,#2844));
#747=EDGE_LOOP('',(#2845,#2846,#2847,#2848,#2849,#2850,#2851,#2852));
#748=EDGE_LOOP('',(#2853,#2854,#2855,#2856,#2857,#2858,#2859,#2860,#2861,
#2862,#2863,#2864,#2865,#2866,#2867,#2868));
#749=EDGE_LOOP('',(#2869,#2870,#2871,#2872,#2873,#2874,#2875,#2876));
#863=LINE('',#4898,#1092);
#864=LINE('',#4927,#1093);
#865=LINE('',#4957,#1094);
#866=LINE('',#5005,#1095);
#867=LINE('',#5056,#1096);
#868=LINE('',#5107,#1097);
#869=LINE('',#5155,#1098);
#870=LINE('',#5206,#1099);
#871=LINE('',#5257,#1100);
#872=LINE('',#5305,#1101);
#873=LINE('',#5356,#1102);
#874=LINE('',#5407,#1103);
#875=LINE('',#5455,#1104);
#876=LINE('',#5506,#1105);
#877=LINE('',#5545,#1106);
#878=LINE('',#5565,#1107);
#879=LINE('',#5590,#1108);
#880=LINE('',#5615,#1109);
#881=LINE('',#5639,#1110);
#882=LINE('',#5664,#1111);
#883=LINE('',#5689,#1112);
#884=LINE('',#5713,#1113);
#885=LINE('',#5738,#1114);
#886=LINE('',#5763,#1115);
#887=LINE('',#5787,#1116);
#888=LINE('',#5812,#1117);
#889=LINE('',#5837,#1118);
#890=LINE('',#5861,#1119);
#891=LINE('',#5878,#1120);
#892=LINE('',#5907,#1121);
#893=LINE('',#5937,#1122);
#894=LINE('',#5985,#1123);
#895=LINE('',#6036,#1124);
#896=LINE('',#6087,#1125);
#897=LINE('',#6135,#1126);
#898=LINE('',#6186,#1127);
#899=LINE('',#6237,#1128);
#900=LINE('',#6285,#1129);
#901=LINE('',#6336,#1130);
#902=LINE('',#6387,#1131);
#903=LINE('',#6435,#1132);
#904=LINE('',#6486,#1133);
#905=LINE('',#6525,#1134);
#906=LINE('',#6545,#1135);
#907=LINE('',#6570,#1136);
#908=LINE('',#6595,#1137);
#909=LINE('',#6619,#1138);
#910=LINE('',#6644,#1139);
#911=LINE('',#6669,#1140);
#912=LINE('',#6693,#1141);
#913=LINE('',#6718,#1142);
#914=LINE('',#6743,#1143);
#915=LINE('',#6767,#1144);
#916=LINE('',#6792,#1145);
#917=LINE('',#6817,#1146);
#918=LINE('',#6841,#1147);
#919=LINE('',#6859,#1148);
#920=LINE('',#6866,#1149);
#921=LINE('',#9210,#1150);
#922=LINE('',#9212,#1151);
#923=LINE('',#9214,#1152);
#924=LINE('',#9215,#1153);
#925=LINE('',#9221,#1154);
#926=LINE('',#9224,#1155);
#927=LINE('',#9226,#1156);
#928=LINE('',#9227,#1157);
#929=LINE('',#9233,#1158);
#930=LINE('',#9236,#1159);
#931=LINE('',#9238,#1160);
#932=LINE('',#9239,#1161);
#933=LINE('',#9245,#1162);
#934=LINE('',#9248,#1163);
#935=LINE('',#9250,#1164);
#936=LINE('',#9251,#1165);
#937=LINE('',#9260,#1166);
#938=LINE('',#9263,#1167);
#939=LINE('',#9266,#1168);
#940=LINE('',#9268,#1169);
#941=LINE('',#9269,#1170);
#942=LINE('',#9275,#1171);
#943=LINE('',#9278,#1172);
#944=LINE('',#9280,#1173);
#945=LINE('',#9281,#1174);
#946=LINE('',#9284,#1175);
#947=LINE('',#9286,#1176);
#948=LINE('',#9287,#1177);
#949=LINE('',#9290,#1178);
#950=LINE('',#9292,#1179);
#951=LINE('',#9293,#1180);
#952=LINE('',#9296,#1181);
#953=LINE('',#9298,#1182);
#954=LINE('',#9299,#1183);
#955=LINE('',#9302,#1184);
#956=LINE('',#9304,#1185);
#957=LINE('',#9305,#1186);
#958=LINE('',#9311,#1187);
#959=LINE('',#9314,#1188);
#960=LINE('',#9316,#1189);
#961=LINE('',#9317,#1190);
#962=LINE('',#9323,#1191);
#963=LINE('',#9326,#1192);
#964=LINE('',#9328,#1193);
#965=LINE('',#9329,#1194);
#966=LINE('',#9332,#1195);
#967=LINE('',#9334,#1196);
#968=LINE('',#9335,#1197);
#969=LINE('',#9338,#1198);
#970=LINE('',#9340,#1199);
#971=LINE('',#9341,#1200);
#972=LINE('',#9344,#1201);
#973=LINE('',#9346,#1202);
#974=LINE('',#9347,#1203);
#975=LINE('',#9349,#1204);
#976=LINE('',#9350,#1205);
#1092=VECTOR('',#4134,2.5);
#1093=VECTOR('',#4137,2.5);
#1094=VECTOR('',#4142,2.5);
#1095=VECTOR('',#4145,2.5);
#1096=VECTOR('',#4148,2.5);
#1097=VECTOR('',#4151,2.5);
#1098=VECTOR('',#4154,2.5);
#1099=VECTOR('',#4157,2.5);
#1100=VECTOR('',#4160,2.5);
#1101=VECTOR('',#4163,2.5);
#1102=VECTOR('',#4166,2.5);
#1103=VECTOR('',#4169,2.5);
#1104=VECTOR('',#4172,2.5);
#1105=VECTOR('',#4175,2.5);
#1106=VECTOR('',#4180,2.56);
#1107=VECTOR('',#4185,2.56);
#1108=VECTOR('',#4188,2.56);
#1109=VECTOR('',#4191,2.56);
#1110=VECTOR('',#4194,2.56);
#1111=VECTOR('',#4197,2.56);
#1112=VECTOR('',#4200,2.56);
#1113=VECTOR('',#4203,2.56);
#1114=VECTOR('',#4206,2.56);
#1115=VECTOR('',#4209,2.56);
#1116=VECTOR('',#4212,2.56);
#1117=VECTOR('',#4215,2.56);
#1118=VECTOR('',#4218,2.56);
#1119=VECTOR('',#4221,2.56);
#1120=VECTOR('',#4226,2.5);
#1121=VECTOR('',#4229,2.5);
#1122=VECTOR('',#4234,2.5);
#1123=VECTOR('',#4237,2.5);
#1124=VECTOR('',#4240,2.5);
#1125=VECTOR('',#4243,2.5);
#1126=VECTOR('',#4246,2.5);
#1127=VECTOR('',#4249,2.5);
#1128=VECTOR('',#4252,2.5);
#1129=VECTOR('',#4255,2.5);
#1130=VECTOR('',#4258,2.5);
#1131=VECTOR('',#4261,2.5);
#1132=VECTOR('',#4264,2.5);
#1133=VECTOR('',#4267,2.5);
#1134=VECTOR('',#4272,2.56);
#1135=VECTOR('',#4277,2.56);
#1136=VECTOR('',#4280,2.56);
#1137=VECTOR('',#4283,2.56);
#1138=VECTOR('',#4286,2.56);
#1139=VECTOR('',#4289,2.56);
#1140=VECTOR('',#4292,2.56);
#1141=VECTOR('',#4295,2.56);
#1142=VECTOR('',#4298,2.56);
#1143=VECTOR('',#4301,2.56);
#1144=VECTOR('',#4304,2.56);
#1145=VECTOR('',#4307,2.56);
#1146=VECTOR('',#4310,2.56);
#1147=VECTOR('',#4313,2.56);
#1148=VECTOR('',#4320,1.);
#1149=VECTOR('',#4329,1.);
#1150=VECTOR('',#4352,10.);
#1151=VECTOR('',#4353,10.);
#1152=VECTOR('',#4354,10.);
#1153=VECTOR('',#4355,10.);
#1154=VECTOR('',#4362,10.);
#1155=VECTOR('',#4365,10.);
#1156=VECTOR('',#4366,10.);
#1157=VECTOR('',#4367,10.);
#1158=VECTOR('',#4374,10.);
#1159=VECTOR('',#4377,10.);
#1160=VECTOR('',#4378,10.);
#1161=VECTOR('',#4379,10.);
#1162=VECTOR('',#4386,10.);
#1163=VECTOR('',#4389,10.);
#1164=VECTOR('',#4390,10.);
#1165=VECTOR('',#4391,10.);
#1166=VECTOR('',#4402,10.);
#1167=VECTOR('',#4405,10.);
#1168=VECTOR('',#4408,10.);
#1169=VECTOR('',#4409,10.);
#1170=VECTOR('',#4410,10.);
#1171=VECTOR('',#4417,10.);
#1172=VECTOR('',#4420,10.);
#1173=VECTOR('',#4421,10.);
#1174=VECTOR('',#4422,10.);
#1175=VECTOR('',#4425,10.);
#1176=VECTOR('',#4426,10.);
#1177=VECTOR('',#4427,10.);
#1178=VECTOR('',#4430,10.);
#1179=VECTOR('',#4431,10.);
#1180=VECTOR('',#4432,10.);
#1181=VECTOR('',#4435,10.);
#1182=VECTOR('',#4436,10.);
#1183=VECTOR('',#4437,10.);
#1184=VECTOR('',#4440,10.);
#1185=VECTOR('',#4441,10.);
#1186=VECTOR('',#4442,10.);
#1187=VECTOR('',#4449,10.);
#1188=VECTOR('',#4452,10.);
#1189=VECTOR('',#4453,10.);
#1190=VECTOR('',#4454,10.);
#1191=VECTOR('',#4461,10.);
#1192=VECTOR('',#4464,10.);
#1193=VECTOR('',#4465,10.);
#1194=VECTOR('',#4466,10.);
#1195=VECTOR('',#4469,10.);
#1196=VECTOR('',#4470,10.);
#1197=VECTOR('',#4471,10.);
#1198=VECTOR('',#4474,10.);
#1199=VECTOR('',#4475,10.);
#1200=VECTOR('',#4476,10.);
#1201=VECTOR('',#4479,10.);
#1202=VECTOR('',#4480,10.);
#1203=VECTOR('',#4481,10.);
#1204=VECTOR('',#4484,10.);
#1205=VECTOR('',#4485,10.);
#1317=CIRCLE('',#3804,2.117);
#1318=CIRCLE('',#3805,2.117);
#1319=CIRCLE('',#3818,2.117);
#1320=CIRCLE('',#3820,2.56);
#1321=CIRCLE('',#3834,2.56);
#1322=CIRCLE('',#3836,2.117);
#1323=CIRCLE('',#3837,2.117);
#1324=CIRCLE('',#3850,2.117);
#1325=CIRCLE('',#3852,2.56);
#1326=CIRCLE('',#3866,2.56);
#1327=CIRCLE('',#3868,1.);
#1328=CIRCLE('',#3869,1.);
#1329=CIRCLE('',#3872,1.);
#1330=CIRCLE('',#3873,1.);
#1331=CIRCLE('',#3885,1.99999999999999);
#1332=CIRCLE('',#3886,1.99999999999999);
#1333=CIRCLE('',#3889,1.99999999999999);
#1334=CIRCLE('',#3890,1.99999999999999);
#1335=CIRCLE('',#3893,2.);
#1336=CIRCLE('',#3894,2.);
#1337=CIRCLE('',#3897,2.);
#1338=CIRCLE('',#3898,2.);
#1339=CIRCLE('',#3900,2.);
#1340=CIRCLE('',#3901,2.);
#1341=CIRCLE('',#3904,2.00000000000001);
#1342=CIRCLE('',#3905,2.00000000000001);
#1343=CIRCLE('',#3912,2.00000000000001);
#1344=CIRCLE('',#3913,2.00000000000001);
#1345=CIRCLE('',#3916,2.);
#1346=CIRCLE('',#3917,2.);
#1384=VERTEX_POINT('',#4896);
#1385=VERTEX_POINT('',#4897);
#1386=VERTEX_POINT('',#4899);
#1387=VERTEX_POINT('',#4919);
#1388=VERTEX_POINT('',#4921);
#1389=VERTEX_POINT('',#4926);
#1390=VERTEX_POINT('',#4955);
#1391=VERTEX_POINT('',#4956);
#1392=VERTEX_POINT('',#5003);
#1393=VERTEX_POINT('',#5004);
#1394=VERTEX_POINT('',#5054);
#1395=VERTEX_POINT('',#5055);
#1396=VERTEX_POINT('',#5105);
#1397=VERTEX_POINT('',#5106);
#1398=VERTEX_POINT('',#5153);
#1399=VERTEX_POINT('',#5154);
#1400=VERTEX_POINT('',#5204);
#1401=VERTEX_POINT('',#5205);
#1402=VERTEX_POINT('',#5255);
#1403=VERTEX_POINT('',#5256);
#1404=VERTEX_POINT('',#5303);
#1405=VERTEX_POINT('',#5304);
#1406=VERTEX_POINT('',#5354);
#1407=VERTEX_POINT('',#5355);
#1408=VERTEX_POINT('',#5405);
#1409=VERTEX_POINT('',#5406);
#1410=VERTEX_POINT('',#5453);
#1411=VERTEX_POINT('',#5454);
#1412=VERTEX_POINT('',#5504);
#1413=VERTEX_POINT('',#5505);
#1414=VERTEX_POINT('',#5507);
#1415=VERTEX_POINT('',#5521);
#1416=VERTEX_POINT('',#5543);
#1417=VERTEX_POINT('',#5544);
#1418=VERTEX_POINT('',#5546);
#1419=VERTEX_POINT('',#5553);
#1420=VERTEX_POINT('',#5563);
#1421=VERTEX_POINT('',#5564);
#1422=VERTEX_POINT('',#5588);
#1423=VERTEX_POINT('',#5589);
#1424=VERTEX_POINT('',#5613);
#1425=VERTEX_POINT('',#5614);
#1426=VERTEX_POINT('',#5637);
#1427=VERTEX_POINT('',#5638);
#1428=VERTEX_POINT('',#5662);
#1429=VERTEX_POINT('',#5663);
#1430=VERTEX_POINT('',#5687);
#1431=VERTEX_POINT('',#5688);
#1432=VERTEX_POINT('',#5711);
#1433=VERTEX_POINT('',#5712);
#1434=VERTEX_POINT('',#5736);
#1435=VERTEX_POINT('',#5737);
#1436=VERTEX_POINT('',#5761);
#1437=VERTEX_POINT('',#5762);
#1438=VERTEX_POINT('',#5785);
#1439=VERTEX_POINT('',#5786);
#1440=VERTEX_POINT('',#5810);
#1441=VERTEX_POINT('',#5811);
#1442=VERTEX_POINT('',#5835);
#1443=VERTEX_POINT('',#5836);
#1444=VERTEX_POINT('',#5859);
#1445=VERTEX_POINT('',#5860);
#1446=VERTEX_POINT('',#5862);
#1447=VERTEX_POINT('',#5868);
#1448=VERTEX_POINT('',#5876);
#1449=VERTEX_POINT('',#5877);
#1450=VERTEX_POINT('',#5879);
#1451=VERTEX_POINT('',#5899);
#1452=VERTEX_POINT('',#5901);
#1453=VERTEX_POINT('',#5906);
#1454=VERTEX_POINT('',#5935);
#1455=VERTEX_POINT('',#5936);
#1456=VERTEX_POINT('',#5983);
#1457=VERTEX_POINT('',#5984);
#1458=VERTEX_POINT('',#6034);
#1459=VERTEX_POINT('',#6035);
#1460=VERTEX_POINT('',#6085);
#1461=VERTEX_POINT('',#6086);
#1462=VERTEX_POINT('',#6133);
#1463=VERTEX_POINT('',#6134);
#1464=VERTEX_POINT('',#6184);
#1465=VERTEX_POINT('',#6185);
#1466=VERTEX_POINT('',#6235);
#1467=VERTEX_POINT('',#6236);
#1468=VERTEX_POINT('',#6283);
#1469=VERTEX_POINT('',#6284);
#1470=VERTEX_POINT('',#6334);
#1471=VERTEX_POINT('',#6335);
#1472=VERTEX_POINT('',#6385);
#1473=VERTEX_POINT('',#6386);
#1474=VERTEX_POINT('',#6433);
#1475=VERTEX_POINT('',#6434);
#1476=VERTEX_POINT('',#6484);
#1477=VERTEX_POINT('',#6485);
#1478=VERTEX_POINT('',#6487);
#1479=VERTEX_POINT('',#6501);
#1480=VERTEX_POINT('',#6523);
#1481=VERTEX_POINT('',#6524);
#1482=VERTEX_POINT('',#6526);
#1483=VERTEX_POINT('',#6533);
#1484=VERTEX_POINT('',#6543);
#1485=VERTEX_POINT('',#6544);
#1486=VERTEX_POINT('',#6568);
#1487=VERTEX_POINT('',#6569);
#1488=VERTEX_POINT('',#6593);
#1489=VERTEX_POINT('',#6594);
#1490=VERTEX_POINT('',#6617);
#1491=VERTEX_POINT('',#6618);
#1492=VERTEX_POINT('',#6642);
#1493=VERTEX_POINT('',#6643);
#1494=VERTEX_POINT('',#6667);
#1495=VERTEX_POINT('',#6668);
#1496=VERTEX_POINT('',#6691);
#1497=VERTEX_POINT('',#6692);
#1498=VERTEX_POINT('',#6716);
#1499=VERTEX_POINT('',#6717);
#1500=VERTEX_POINT('',#6741);
#1501=VERTEX_POINT('',#6742);
#1502=VERTEX_POINT('',#6765);
#1503=VERTEX_POINT('',#6766);
#1504=VERTEX_POINT('',#6790);
#1505=VERTEX_POINT('',#6791);
#1506=VERTEX_POINT('',#6815);
#1507=VERTEX_POINT('',#6816);
#1508=VERTEX_POINT('',#6839);
#1509=VERTEX_POINT('',#6840);
#1510=VERTEX_POINT('',#6842);
#1511=VERTEX_POINT('',#6848);
#1512=VERTEX_POINT('',#6856);
#1513=VERTEX_POINT('',#6858);
#1514=VERTEX_POINT('',#6863);
#1515=VERTEX_POINT('',#6865);
#1516=VERTEX_POINT('',#9208);
#1517=VERTEX_POINT('',#9209);
#1518=VERTEX_POINT('',#9211);
#1519=VERTEX_POINT('',#9213);
#1520=VERTEX_POINT('',#9217);
#1521=VERTEX_POINT('',#9219);
#1522=VERTEX_POINT('',#9223);
#1523=VERTEX_POINT('',#9225);
#1524=VERTEX_POINT('',#9229);
#1525=VERTEX_POINT('',#9231);
#1526=VERTEX_POINT('',#9235);
#1527=VERTEX_POINT('',#9237);
#1528=VERTEX_POINT('',#9241);
#1529=VERTEX_POINT('',#9243);
#1530=VERTEX_POINT('',#9247);
#1531=VERTEX_POINT('',#9249);
#1532=VERTEX_POINT('',#9256);
#1533=VERTEX_POINT('',#9257);
#1534=VERTEX_POINT('',#9259);
#1535=VERTEX_POINT('',#9261);
#1536=VERTEX_POINT('',#9265);
#1537=VERTEX_POINT('',#9267);
#1538=VERTEX_POINT('',#9271);
#1539=VERTEX_POINT('',#9273);
#1540=VERTEX_POINT('',#9277);
#1541=VERTEX_POINT('',#9279);
#1542=VERTEX_POINT('',#9283);
#1543=VERTEX_POINT('',#9285);
#1544=VERTEX_POINT('',#9289);
#1545=VERTEX_POINT('',#9291);
#1546=VERTEX_POINT('',#9295);
#1547=VERTEX_POINT('',#9297);
#1548=VERTEX_POINT('',#9301);
#1549=VERTEX_POINT('',#9303);
#1550=VERTEX_POINT('',#9307);
#1551=VERTEX_POINT('',#9309);
#1552=VERTEX_POINT('',#9313);
#1553=VERTEX_POINT('',#9315);
#1554=VERTEX_POINT('',#9319);
#1555=VERTEX_POINT('',#9321);
#1556=VERTEX_POINT('',#9325);
#1557=VERTEX_POINT('',#9327);
#1558=VERTEX_POINT('',#9331);
#1559=VERTEX_POINT('',#9333);
#1560=VERTEX_POINT('',#9337);
#1561=VERTEX_POINT('',#9339);
#1562=VERTEX_POINT('',#9343);
#1563=VERTEX_POINT('',#9345);
#1758=EDGE_CURVE('',#1384,#1385,#863,.T.);
#1759=EDGE_CURVE('',#1385,#1386,#62,.T.);
#1760=EDGE_CURVE('',#1386,#1387,#1317,.T.);
#1761=EDGE_CURVE('',#1387,#1388,#63,.T.);
#1762=EDGE_CURVE('',#1388,#1389,#864,.T.);
#1763=EDGE_CURVE('',#1389,#1389,#1318,.F.);
#1764=EDGE_CURVE('',#1388,#1384,#64,.T.);
#1765=EDGE_CURVE('',#1390,#1391,#865,.T.);
#1766=EDGE_CURVE('',#1391,#1385,#65,.T.);
#1767=EDGE_CURVE('',#1384,#1390,#66,.T.);
#1768=EDGE_CURVE('',#1392,#1393,#866,.T.);
#1769=EDGE_CURVE('',#1393,#1391,#67,.T.);
#1770=EDGE_CURVE('',#1390,#1392,#68,.T.);
#1771=EDGE_CURVE('',#1394,#1395,#867,.T.);
#1772=EDGE_CURVE('',#1395,#1393,#69,.T.);
#1773=EDGE_CURVE('',#1392,#1394,#70,.T.);
#1774=EDGE_CURVE('',#1396,#1397,#868,.T.);
#1775=EDGE_CURVE('',#1397,#1395,#71,.T.);
#1776=EDGE_CURVE('',#1394,#1396,#72,.T.);
#1777=EDGE_CURVE('',#1398,#1399,#869,.T.);
#1778=EDGE_CURVE('',#1399,#1397,#73,.T.);
#1779=EDGE_CURVE('',#1396,#1398,#74,.T.);
#1780=EDGE_CURVE('',#1400,#1401,#870,.T.);
#1781=EDGE_CURVE('',#1401,#1399,#75,.T.);
#1782=EDGE_CURVE('',#1398,#1400,#76,.T.);
#1783=EDGE_CURVE('',#1402,#1403,#871,.T.);
#1784=EDGE_CURVE('',#1403,#1401,#77,.T.);
#1785=EDGE_CURVE('',#1400,#1402,#78,.T.);
#1786=EDGE_CURVE('',#1404,#1405,#872,.T.);
#1787=EDGE_CURVE('',#1405,#1403,#79,.T.);
#1788=EDGE_CURVE('',#1402,#1404,#80,.T.);
#1789=EDGE_CURVE('',#1406,#1407,#873,.T.);
#1790=EDGE_CURVE('',#1407,#1405,#81,.T.);
#1791=EDGE_CURVE('',#1404,#1406,#82,.T.);
#1792=EDGE_CURVE('',#1408,#1409,#874,.T.);
#1793=EDGE_CURVE('',#1409,#1407,#83,.T.);
#1794=EDGE_CURVE('',#1406,#1408,#84,.T.);
#1795=EDGE_CURVE('',#1410,#1411,#875,.T.);
#1796=EDGE_CURVE('',#1411,#1409,#85,.T.);
#1797=EDGE_CURVE('',#1408,#1410,#86,.T.);
#1798=EDGE_CURVE('',#1412,#1413,#876,.T.);
#1799=EDGE_CURVE('',#1412,#1414,#87,.T.);
#1800=EDGE_CURVE('',#1415,#1414,#1319,.T.);
#1801=EDGE_CURVE('',#1415,#1413,#88,.T.);
#1802=EDGE_CURVE('',#1416,#1417,#877,.T.);
#1803=EDGE_CURVE('',#1417,#1418,#89,.T.);
#1804=EDGE_CURVE('',#1419,#1418,#1320,.T.);
#1805=EDGE_CURVE('',#1416,#1419,#90,.T.);
#1806=EDGE_CURVE('',#1420,#1421,#878,.T.);
#1807=EDGE_CURVE('',#1421,#1417,#91,.T.);
#1808=EDGE_CURVE('',#1420,#1416,#92,.T.);
#1809=EDGE_CURVE('',#1422,#1423,#879,.T.);
#1810=EDGE_CURVE('',#1423,#1421,#93,.T.);
#1811=EDGE_CURVE('',#1422,#1420,#94,.T.);
#1812=EDGE_CURVE('',#1424,#1425,#880,.T.);
#1813=EDGE_CURVE('',#1425,#1423,#95,.T.);
#1814=EDGE_CURVE('',#1424,#1422,#96,.T.);
#1815=EDGE_CURVE('',#1426,#1427,#881,.T.);
#1816=EDGE_CURVE('',#1427,#1425,#97,.T.);
#1817=EDGE_CURVE('',#1426,#1424,#98,.T.);
#1818=EDGE_CURVE('',#1428,#1429,#882,.T.);
#1819=EDGE_CURVE('',#1429,#1427,#99,.T.);
#1820=EDGE_CURVE('',#1428,#1426,#100,.T.);
#1821=EDGE_CURVE('',#1430,#1431,#883,.T.);
#1822=EDGE_CURVE('',#1431,#1429,#101,.T.);
#1823=EDGE_CURVE('',#1430,#1428,#102,.T.);
#1824=EDGE_CURVE('',#1432,#1433,#884,.T.);
#1825=EDGE_CURVE('',#1433,#1431,#103,.T.);
#1826=EDGE_CURVE('',#1432,#1430,#104,.T.);
#1827=EDGE_CURVE('',#1434,#1435,#885,.T.);
#1828=EDGE_CURVE('',#1435,#1433,#105,.T.);
#1829=EDGE_CURVE('',#1434,#1432,#106,.T.);
#1830=EDGE_CURVE('',#1436,#1437,#886,.T.);
#1831=EDGE_CURVE('',#1437,#1435,#107,.T.);
#1832=EDGE_CURVE('',#1436,#1434,#108,.T.);
#1833=EDGE_CURVE('',#1438,#1439,#887,.T.);
#1834=EDGE_CURVE('',#1439,#1437,#109,.T.);
#1835=EDGE_CURVE('',#1438,#1436,#110,.T.);
#1836=EDGE_CURVE('',#1440,#1441,#888,.T.);
#1837=EDGE_CURVE('',#1441,#1439,#111,.T.);
#1838=EDGE_CURVE('',#1440,#1438,#112,.T.);
#1839=EDGE_CURVE('',#1442,#1443,#889,.T.);
#1840=EDGE_CURVE('',#1443,#1441,#113,.T.);
#1841=EDGE_CURVE('',#1442,#1440,#114,.T.);
#1842=EDGE_CURVE('',#1444,#1445,#890,.T.);
#1843=EDGE_CURVE('',#1446,#1444,#115,.T.);
#1844=EDGE_CURVE('',#1447,#1446,#1321,.T.);
#1845=EDGE_CURVE('',#1447,#1445,#116,.T.);
#1846=EDGE_CURVE('',#1448,#1449,#891,.T.);
#1847=EDGE_CURVE('',#1449,#1450,#117,.T.);
#1848=EDGE_CURVE('',#1450,#1451,#1322,.T.);
#1849=EDGE_CURVE('',#1451,#1452,#118,.T.);
#1850=EDGE_CURVE('',#1452,#1453,#892,.T.);
#1851=EDGE_CURVE('',#1453,#1453,#1323,.F.);
#1852=EDGE_CURVE('',#1452,#1448,#119,.T.);
#1853=EDGE_CURVE('',#1454,#1455,#893,.T.);
#1854=EDGE_CURVE('',#1455,#1449,#120,.T.);
#1855=EDGE_CURVE('',#1448,#1454,#121,.T.);
#1856=EDGE_CURVE('',#1456,#1457,#894,.T.);
#1857=EDGE_CURVE('',#1457,#1455,#122,.T.);
#1858=EDGE_CURVE('',#1454,#1456,#123,.T.);
#1859=EDGE_CURVE('',#1458,#1459,#895,.T.);
#1860=EDGE_CURVE('',#1459,#1457,#124,.T.);
#1861=EDGE_CURVE('',#1456,#1458,#125,.T.);
#1862=EDGE_CURVE('',#1460,#1461,#896,.T.);
#1863=EDGE_CURVE('',#1461,#1459,#126,.T.);
#1864=EDGE_CURVE('',#1458,#1460,#127,.T.);
#1865=EDGE_CURVE('',#1462,#1463,#897,.T.);
#1866=EDGE_CURVE('',#1463,#1461,#128,.T.);
#1867=EDGE_CURVE('',#1460,#1462,#129,.T.);
#1868=EDGE_CURVE('',#1464,#1465,#898,.T.);
#1869=EDGE_CURVE('',#1465,#1463,#130,.T.);
#1870=EDGE_CURVE('',#1462,#1464,#131,.T.);
#1871=EDGE_CURVE('',#1466,#1467,#899,.T.);
#1872=EDGE_CURVE('',#1467,#1465,#132,.T.);
#1873=EDGE_CURVE('',#1464,#1466,#133,.T.);
#1874=EDGE_CURVE('',#1468,#1469,#900,.T.);
#1875=EDGE_CURVE('',#1469,#1467,#134,.T.);
#1876=EDGE_CURVE('',#1466,#1468,#135,.T.);
#1877=EDGE_CURVE('',#1470,#1471,#901,.T.);
#1878=EDGE_CURVE('',#1471,#1469,#136,.T.);
#1879=EDGE_CURVE('',#1468,#1470,#137,.T.);
#1880=EDGE_CURVE('',#1472,#1473,#902,.T.);
#1881=EDGE_CURVE('',#1473,#1471,#138,.T.);
#1882=EDGE_CURVE('',#1470,#1472,#139,.T.);
#1883=EDGE_CURVE('',#1474,#1475,#903,.T.);
#1884=EDGE_CURVE('',#1475,#1473,#140,.T.);
#1885=EDGE_CURVE('',#1472,#1474,#141,.T.);
#1886=EDGE_CURVE('',#1476,#1477,#904,.T.);
#1887=EDGE_CURVE('',#1476,#1478,#142,.T.);
#1888=EDGE_CURVE('',#1479,#1478,#1324,.T.);
#1889=EDGE_CURVE('',#1479,#1477,#143,.T.);
#1890=EDGE_CURVE('',#1480,#1481,#905,.T.);
#1891=EDGE_CURVE('',#1481,#1482,#144,.T.);
#1892=EDGE_CURVE('',#1483,#1482,#1325,.T.);
#1893=EDGE_CURVE('',#1480,#1483,#145,.T.);
#1894=EDGE_CURVE('',#1484,#1485,#906,.T.);
#1895=EDGE_CURVE('',#1485,#1481,#146,.T.);
#1896=EDGE_CURVE('',#1484,#1480,#147,.T.);
#1897=EDGE_CURVE('',#1486,#1487,#907,.T.);
#1898=EDGE_CURVE('',#1487,#1485,#148,.T.);
#1899=EDGE_CURVE('',#1486,#1484,#149,.T.);
#1900=EDGE_CURVE('',#1488,#1489,#908,.T.);
#1901=EDGE_CURVE('',#1489,#1487,#150,.T.);
#1902=EDGE_CURVE('',#1488,#1486,#151,.T.);
#1903=EDGE_CURVE('',#1490,#1491,#909,.T.);
#1904=EDGE_CURVE('',#1491,#1489,#152,.T.);
#1905=EDGE_CURVE('',#1490,#1488,#153,.T.);
#1906=EDGE_CURVE('',#1492,#1493,#910,.T.);
#1907=EDGE_CURVE('',#1493,#1491,#154,.T.);
#1908=EDGE_CURVE('',#1492,#1490,#155,.T.);
#1909=EDGE_CURVE('',#1494,#1495,#911,.T.);
#1910=EDGE_CURVE('',#1495,#1493,#156,.T.);
#1911=EDGE_CURVE('',#1494,#1492,#157,.T.);
#1912=EDGE_CURVE('',#1496,#1497,#912,.T.);
#1913=EDGE_CURVE('',#1497,#1495,#158,.T.);
#1914=EDGE_CURVE('',#1496,#1494,#159,.T.);
#1915=EDGE_CURVE('',#1498,#1499,#913,.T.);
#1916=EDGE_CURVE('',#1499,#1497,#160,.T.);
#1917=EDGE_CURVE('',#1498,#1496,#161,.T.);
#1918=EDGE_CURVE('',#1500,#1501,#914,.T.);
#1919=EDGE_CURVE('',#1501,#1499,#162,.T.);
#1920=EDGE_CURVE('',#1500,#1498,#163,.T.);
#1921=EDGE_CURVE('',#1502,#1503,#915,.T.);
#1922=EDGE_CURVE('',#1503,#1501,#164,.T.);
#1923=EDGE_CURVE('',#1502,#1500,#165,.T.);
#1924=EDGE_CURVE('',#1504,#1505,#916,.T.);
#1925=EDGE_CURVE('',#1505,#1503,#166,.T.);
#1926=EDGE_CURVE('',#1504,#1502,#167,.T.);
#1927=EDGE_CURVE('',#1506,#1507,#917,.T.);
#1928=EDGE_CURVE('',#1507,#1505,#168,.T.);
#1929=EDGE_CURVE('',#1506,#1504,#169,.T.);
#1930=EDGE_CURVE('',#1508,#1509,#918,.T.);
#1931=EDGE_CURVE('',#1510,#1508,#170,.T.);
#1932=EDGE_CURVE('',#1511,#1510,#1326,.T.);
#1933=EDGE_CURVE('',#1511,#1509,#171,.T.);
#1934=EDGE_CURVE('',#1512,#1512,#1327,.T.);
#1935=EDGE_CURVE('',#1512,#1513,#919,.T.);
#1936=EDGE_CURVE('',#1513,#1513,#1328,.T.);
#1937=EDGE_CURVE('',#1514,#1514,#1329,.T.);
#1938=EDGE_CURVE('',#1514,#1515,#920,.T.);
#1939=EDGE_CURVE('',#1515,#1515,#1330,.T.);
#1940=EDGE_CURVE('',#1450,#1483,#172,.T.);
#1941=EDGE_CURVE('',#1482,#1451,#173,.T.);
#1942=EDGE_CURVE('',#1509,#1507,#174,.T.);
#1943=EDGE_CURVE('',#1508,#1506,#175,.T.);
#1944=EDGE_CURVE('',#1478,#1511,#176,.T.);
#1945=EDGE_CURVE('',#1474,#1476,#177,.T.);
#1946=EDGE_CURVE('',#1477,#1475,#178,.T.);
#1947=EDGE_CURVE('',#1510,#1479,#179,.T.);
#1948=EDGE_CURVE('',#1386,#1419,#180,.T.);
#1949=EDGE_CURVE('',#1418,#1387,#181,.T.);
#1950=EDGE_CURVE('',#1445,#1443,#182,.T.);
#1951=EDGE_CURVE('',#1444,#1442,#183,.T.);
#1952=EDGE_CURVE('',#1414,#1447,#184,.T.);
#1953=EDGE_CURVE('',#1410,#1412,#185,.T.);
#1954=EDGE_CURVE('',#1413,#1411,#186,.T.);
#1955=EDGE_CURVE('',#1446,#1415,#187,.T.);
#1956=EDGE_CURVE('',#1516,#1517,#921,.T.);
#1957=EDGE_CURVE('',#1517,#1518,#922,.T.);
#1958=EDGE_CURVE('',#1519,#1518,#923,.T.);
#1959=EDGE_CURVE('',#1516,#1519,#924,.T.);
#1960=EDGE_CURVE('',#1520,#1516,#1331,.T.);
#1961=EDGE_CURVE('',#1521,#1519,#1332,.T.);
#1962=EDGE_CURVE('',#1520,#1521,#925,.T.);
#1963=EDGE_CURVE('',#1522,#1520,#926,.T.);
#1964=EDGE_CURVE('',#1523,#1521,#927,.T.);
#1965=EDGE_CURVE('',#1522,#1523,#928,.T.);
#1966=EDGE_CURVE('',#1524,#1522,#1333,.T.);
#1967=EDGE_CURVE('',#1525,#1523,#1334,.T.);
#1968=EDGE_CURVE('',#1524,#1525,#929,.T.);
#1969=EDGE_CURVE('',#1526,#1524,#930,.T.);
#1970=EDGE_CURVE('',#1527,#1525,#931,.T.);
#1971=EDGE_CURVE('',#1526,#1527,#932,.T.);
#1972=EDGE_CURVE('',#1528,#1526,#1335,.T.);
#1973=EDGE_CURVE('',#1529,#1527,#1336,.T.);
#1974=EDGE_CURVE('',#1528,#1529,#933,.T.);
#1975=EDGE_CURVE('',#1530,#1528,#934,.T.);
#1976=EDGE_CURVE('',#1531,#1529,#935,.T.);
#1977=EDGE_CURVE('',#1530,#1531,#936,.T.);
#1978=EDGE_CURVE('',#1517,#1530,#1337,.T.);
#1979=EDGE_CURVE('',#1518,#1531,#1338,.T.);
#1980=EDGE_CURVE('',#1532,#1533,#1339,.T.);
#1981=EDGE_CURVE('',#1532,#1534,#937,.T.);
#1982=EDGE_CURVE('',#1535,#1534,#1340,.T.);
#1983=EDGE_CURVE('',#1533,#1535,#938,.T.);
#1984=EDGE_CURVE('',#1536,#1533,#939,.T.);
#1985=EDGE_CURVE('',#1537,#1535,#940,.T.);
#1986=EDGE_CURVE('',#1536,#1537,#941,.T.);
#1987=EDGE_CURVE('',#1536,#1538,#1341,.T.);
#1988=EDGE_CURVE('',#1539,#1537,#1342,.T.);
#1989=EDGE_CURVE('',#1538,#1539,#942,.T.);
#1990=EDGE_CURVE('',#1540,#1538,#943,.T.);
#1991=EDGE_CURVE('',#1541,#1539,#944,.T.);
#1992=EDGE_CURVE('',#1540,#1541,#945,.T.);
#1993=EDGE_CURVE('',#1542,#1540,#946,.T.);
#1994=EDGE_CURVE('',#1543,#1541,#947,.T.);
#1995=EDGE_CURVE('',#1542,#1543,#948,.T.);
#1996=EDGE_CURVE('',#1544,#1542,#949,.T.);
#1997=EDGE_CURVE('',#1545,#1543,#950,.T.);
#1998=EDGE_CURVE('',#1544,#1545,#951,.T.);
#1999=EDGE_CURVE('',#1546,#1544,#952,.T.);
#2000=EDGE_CURVE('',#1547,#1545,#953,.T.);
#2001=EDGE_CURVE('',#1546,#1547,#954,.T.);
#2002=EDGE_CURVE('',#1548,#1546,#955,.T.);
#2003=EDGE_CURVE('',#1549,#1547,#956,.T.);
#2004=EDGE_CURVE('',#1548,#1549,#957,.T.);
#2005=EDGE_CURVE('',#1548,#1550,#1343,.T.);
#2006=EDGE_CURVE('',#1551,#1549,#1344,.T.);
#2007=EDGE_CURVE('',#1550,#1551,#958,.T.);
#2008=EDGE_CURVE('',#1552,#1550,#959,.T.);
#2009=EDGE_CURVE('',#1553,#1551,#960,.T.);
#2010=EDGE_CURVE('',#1552,#1553,#961,.T.);
#2011=EDGE_CURVE('',#1552,#1554,#1345,.T.);
#2012=EDGE_CURVE('',#1555,#1553,#1346,.T.);
#2013=EDGE_CURVE('',#1554,#1555,#962,.T.);
#2014=EDGE_CURVE('',#1556,#1554,#963,.T.);
#2015=EDGE_CURVE('',#1557,#1555,#964,.T.);
#2016=EDGE_CURVE('',#1556,#1557,#965,.T.);
#2017=EDGE_CURVE('',#1558,#1556,#966,.T.);
#2018=EDGE_CURVE('',#1559,#1557,#967,.T.);
#2019=EDGE_CURVE('',#1558,#1559,#968,.T.);
#2020=EDGE_CURVE('',#1560,#1558,#969,.T.);
#2021=EDGE_CURVE('',#1561,#1559,#970,.T.);
#2022=EDGE_CURVE('',#1560,#1561,#971,.T.);
#2023=EDGE_CURVE('',#1562,#1560,#972,.T.);
#2024=EDGE_CURVE('',#1563,#1561,#973,.T.);
#2025=EDGE_CURVE('',#1562,#1563,#974,.T.);
#2026=EDGE_CURVE('',#1532,#1562,#975,.T.);
#2027=EDGE_CURVE('',#1534,#1563,#976,.T.);
#2337=ORIENTED_EDGE('',*,*,#1758,.T.);
#2338=ORIENTED_EDGE('',*,*,#1759,.T.);
#2339=ORIENTED_EDGE('',*,*,#1760,.T.);
#2340=ORIENTED_EDGE('',*,*,#1761,.T.);
#2341=ORIENTED_EDGE('',*,*,#1762,.T.);
#2342=ORIENTED_EDGE('',*,*,#1763,.T.);
#2343=ORIENTED_EDGE('',*,*,#1762,.F.);
#2344=ORIENTED_EDGE('',*,*,#1764,.T.);
#2345=ORIENTED_EDGE('',*,*,#1765,.T.);
#2346=ORIENTED_EDGE('',*,*,#1766,.T.);
#2347=ORIENTED_EDGE('',*,*,#1758,.F.);
#2348=ORIENTED_EDGE('',*,*,#1767,.T.);
#2349=ORIENTED_EDGE('',*,*,#1768,.T.);
#2350=ORIENTED_EDGE('',*,*,#1769,.T.);
#2351=ORIENTED_EDGE('',*,*,#1765,.F.);
#2352=ORIENTED_EDGE('',*,*,#1770,.T.);
#2353=ORIENTED_EDGE('',*,*,#1771,.T.);
#2354=ORIENTED_EDGE('',*,*,#1772,.T.);
#2355=ORIENTED_EDGE('',*,*,#1768,.F.);
#2356=ORIENTED_EDGE('',*,*,#1773,.T.);
#2357=ORIENTED_EDGE('',*,*,#1774,.T.);
#2358=ORIENTED_EDGE('',*,*,#1775,.T.);
#2359=ORIENTED_EDGE('',*,*,#1771,.F.);
#2360=ORIENTED_EDGE('',*,*,#1776,.T.);
#2361=ORIENTED_EDGE('',*,*,#1777,.T.);
#2362=ORIENTED_EDGE('',*,*,#1778,.T.);
#2363=ORIENTED_EDGE('',*,*,#1774,.F.);
#2364=ORIENTED_EDGE('',*,*,#1779,.T.);
#2365=ORIENTED_EDGE('',*,*,#1780,.T.);
#2366=ORIENTED_EDGE('',*,*,#1781,.T.);
#2367=ORIENTED_EDGE('',*,*,#1777,.F.);
#2368=ORIENTED_EDGE('',*,*,#1782,.T.);
#2369=ORIENTED_EDGE('',*,*,#1783,.T.);
#2370=ORIENTED_EDGE('',*,*,#1784,.T.);
#2371=ORIENTED_EDGE('',*,*,#1780,.F.);
#2372=ORIENTED_EDGE('',*,*,#1785,.T.);
#2373=ORIENTED_EDGE('',*,*,#1786,.T.);
#2374=ORIENTED_EDGE('',*,*,#1787,.T.);
#2375=ORIENTED_EDGE('',*,*,#1783,.F.);
#2376=ORIENTED_EDGE('',*,*,#1788,.T.);
#2377=ORIENTED_EDGE('',*,*,#1789,.T.);
#2378=ORIENTED_EDGE('',*,*,#1790,.T.);
#2379=ORIENTED_EDGE('',*,*,#1786,.F.);
#2380=ORIENTED_EDGE('',*,*,#1791,.T.);
#2381=ORIENTED_EDGE('',*,*,#1792,.T.);
#2382=ORIENTED_EDGE('',*,*,#1793,.T.);
#2383=ORIENTED_EDGE('',*,*,#1789,.F.);
#2384=ORIENTED_EDGE('',*,*,#1794,.T.);
#2385=ORIENTED_EDGE('',*,*,#1795,.T.);
#2386=ORIENTED_EDGE('',*,*,#1796,.T.);
#2387=ORIENTED_EDGE('',*,*,#1792,.F.);
#2388=ORIENTED_EDGE('',*,*,#1797,.T.);
#2389=ORIENTED_EDGE('',*,*,#1798,.F.);
#2390=ORIENTED_EDGE('',*,*,#1799,.T.);
#2391=ORIENTED_EDGE('',*,*,#1800,.F.);
#2392=ORIENTED_EDGE('',*,*,#1801,.T.);
#2393=ORIENTED_EDGE('',*,*,#1802,.T.);
#2394=ORIENTED_EDGE('',*,*,#1803,.T.);
#2395=ORIENTED_EDGE('',*,*,#1804,.F.);
#2396=ORIENTED_EDGE('',*,*,#1805,.F.);
#2397=ORIENTED_EDGE('',*,*,#1806,.T.);
#2398=ORIENTED_EDGE('',*,*,#1807,.T.);
#2399=ORIENTED_EDGE('',*,*,#1802,.F.);
#2400=ORIENTED_EDGE('',*,*,#1808,.F.);
#2401=ORIENTED_EDGE('',*,*,#1809,.T.);
#2402=ORIENTED_EDGE('',*,*,#1810,.T.);
#2403=ORIENTED_EDGE('',*,*,#1806,.F.);
#2404=ORIENTED_EDGE('',*,*,#1811,.F.);
#2405=ORIENTED_EDGE('',*,*,#1812,.T.);
#2406=ORIENTED_EDGE('',*,*,#1813,.T.);
#2407=ORIENTED_EDGE('',*,*,#1809,.F.);
#2408=ORIENTED_EDGE('',*,*,#1814,.F.);
#2409=ORIENTED_EDGE('',*,*,#1815,.T.);
#2410=ORIENTED_EDGE('',*,*,#1816,.T.);
#2411=ORIENTED_EDGE('',*,*,#1812,.F.);
#2412=ORIENTED_EDGE('',*,*,#1817,.F.);
#2413=ORIENTED_EDGE('',*,*,#1818,.T.);
#2414=ORIENTED_EDGE('',*,*,#1819,.T.);
#2415=ORIENTED_EDGE('',*,*,#1815,.F.);
#2416=ORIENTED_EDGE('',*,*,#1820,.F.);
#2417=ORIENTED_EDGE('',*,*,#1821,.T.);
#2418=ORIENTED_EDGE('',*,*,#1822,.T.);
#2419=ORIENTED_EDGE('',*,*,#1818,.F.);
#2420=ORIENTED_EDGE('',*,*,#1823,.F.);
#2421=ORIENTED_EDGE('',*,*,#1824,.T.);
#2422=ORIENTED_EDGE('',*,*,#1825,.T.);
#2423=ORIENTED_EDGE('',*,*,#1821,.F.);
#2424=ORIENTED_EDGE('',*,*,#1826,.F.);
#2425=ORIENTED_EDGE('',*,*,#1827,.T.);
#2426=ORIENTED_EDGE('',*,*,#1828,.T.);
#2427=ORIENTED_EDGE('',*,*,#1824,.F.);
#2428=ORIENTED_EDGE('',*,*,#1829,.F.);
#2429=ORIENTED_EDGE('',*,*,#1830,.T.);
#2430=ORIENTED_EDGE('',*,*,#1831,.T.);
#2431=ORIENTED_EDGE('',*,*,#1827,.F.);
#2432=ORIENTED_EDGE('',*,*,#1832,.F.);
#2433=ORIENTED_EDGE('',*,*,#1833,.T.);
#2434=ORIENTED_EDGE('',*,*,#1834,.T.);
#2435=ORIENTED_EDGE('',*,*,#1830,.F.);
#2436=ORIENTED_EDGE('',*,*,#1835,.F.);
#2437=ORIENTED_EDGE('',*,*,#1836,.T.);
#2438=ORIENTED_EDGE('',*,*,#1837,.T.);
#2439=ORIENTED_EDGE('',*,*,#1833,.F.);
#2440=ORIENTED_EDGE('',*,*,#1838,.F.);
#2441=ORIENTED_EDGE('',*,*,#1839,.T.);
#2442=ORIENTED_EDGE('',*,*,#1840,.T.);
#2443=ORIENTED_EDGE('',*,*,#1836,.F.);
#2444=ORIENTED_EDGE('',*,*,#1841,.F.);
#2445=ORIENTED_EDGE('',*,*,#1842,.F.);
#2446=ORIENTED_EDGE('',*,*,#1843,.F.);
#2447=ORIENTED_EDGE('',*,*,#1844,.F.);
#2448=ORIENTED_EDGE('',*,*,#1845,.T.);
#2449=ORIENTED_EDGE('',*,*,#1846,.T.);
#2450=ORIENTED_EDGE('',*,*,#1847,.T.);
#2451=ORIENTED_EDGE('',*,*,#1848,.T.);
#2452=ORIENTED_EDGE('',*,*,#1849,.T.);
#2453=ORIENTED_EDGE('',*,*,#1850,.T.);
#2454=ORIENTED_EDGE('',*,*,#1851,.T.);
#2455=ORIENTED_EDGE('',*,*,#1850,.F.);
#2456=ORIENTED_EDGE('',*,*,#1852,.T.);
#2457=ORIENTED_EDGE('',*,*,#1853,.T.);
#2458=ORIENTED_EDGE('',*,*,#1854,.T.);
#2459=ORIENTED_EDGE('',*,*,#1846,.F.);
#2460=ORIENTED_EDGE('',*,*,#1855,.T.);
#2461=ORIENTED_EDGE('',*,*,#1856,.T.);
#2462=ORIENTED_EDGE('',*,*,#1857,.T.);
#2463=ORIENTED_EDGE('',*,*,#1853,.F.);
#2464=ORIENTED_EDGE('',*,*,#1858,.T.);
#2465=ORIENTED_EDGE('',*,*,#1859,.T.);
#2466=ORIENTED_EDGE('',*,*,#1860,.T.);
#2467=ORIENTED_EDGE('',*,*,#1856,.F.);
#2468=ORIENTED_EDGE('',*,*,#1861,.T.);
#2469=ORIENTED_EDGE('',*,*,#1862,.T.);
#2470=ORIENTED_EDGE('',*,*,#1863,.T.);
#2471=ORIENTED_EDGE('',*,*,#1859,.F.);
#2472=ORIENTED_EDGE('',*,*,#1864,.T.);
#2473=ORIENTED_EDGE('',*,*,#1865,.T.);
#2474=ORIENTED_EDGE('',*,*,#1866,.T.);
#2475=ORIENTED_EDGE('',*,*,#1862,.F.);
#2476=ORIENTED_EDGE('',*,*,#1867,.T.);
#2477=ORIENTED_EDGE('',*,*,#1868,.T.);
#2478=ORIENTED_EDGE('',*,*,#1869,.T.);
#2479=ORIENTED_EDGE('',*,*,#1865,.F.);
#2480=ORIENTED_EDGE('',*,*,#1870,.T.);
#2481=ORIENTED_EDGE('',*,*,#1871,.T.);
#2482=ORIENTED_EDGE('',*,*,#1872,.T.);
#2483=ORIENTED_EDGE('',*,*,#1868,.F.);
#2484=ORIENTED_EDGE('',*,*,#1873,.T.);
#2485=ORIENTED_EDGE('',*,*,#1874,.T.);
#2486=ORIENTED_EDGE('',*,*,#1875,.T.);
#2487=ORIENTED_EDGE('',*,*,#1871,.F.);
#2488=ORIENTED_EDGE('',*,*,#1876,.T.);
#2489=ORIENTED_EDGE('',*,*,#1877,.T.);
#2490=ORIENTED_EDGE('',*,*,#1878,.T.);
#2491=ORIENTED_EDGE('',*,*,#1874,.F.);
#2492=ORIENTED_EDGE('',*,*,#1879,.T.);
#2493=ORIENTED_EDGE('',*,*,#1880,.T.);
#2494=ORIENTED_EDGE('',*,*,#1881,.T.);
#2495=ORIENTED_EDGE('',*,*,#1877,.F.);
#2496=ORIENTED_EDGE('',*,*,#1882,.T.);
#2497=ORIENTED_EDGE('',*,*,#1883,.T.);
#2498=ORIENTED_EDGE('',*,*,#1884,.T.);
#2499=ORIENTED_EDGE('',*,*,#1880,.F.);
#2500=ORIENTED_EDGE('',*,*,#1885,.T.);
#2501=ORIENTED_EDGE('',*,*,#1886,.F.);
#2502=ORIENTED_EDGE('',*,*,#1887,.T.);
#2503=ORIENTED_EDGE('',*,*,#1888,.F.);
#2504=ORIENTED_EDGE('',*,*,#1889,.T.);
#2505=ORIENTED_EDGE('',*,*,#1890,.T.);
#2506=ORIENTED_EDGE('',*,*,#1891,.T.);
#2507=ORIENTED_EDGE('',*,*,#1892,.F.);
#2508=ORIENTED_EDGE('',*,*,#1893,.F.);
#2509=ORIENTED_EDGE('',*,*,#1894,.T.);
#2510=ORIENTED_EDGE('',*,*,#1895,.T.);
#2511=ORIENTED_EDGE('',*,*,#1890,.F.);
#2512=ORIENTED_EDGE('',*,*,#1896,.F.);
#2513=ORIENTED_EDGE('',*,*,#1897,.T.);
#2514=ORIENTED_EDGE('',*,*,#1898,.T.);
#2515=ORIENTED_EDGE('',*,*,#1894,.F.);
#2516=ORIENTED_EDGE('',*,*,#1899,.F.);
#2517=ORIENTED_EDGE('',*,*,#1900,.T.);
#2518=ORIENTED_EDGE('',*,*,#1901,.T.);
#2519=ORIENTED_EDGE('',*,*,#1897,.F.);
#2520=ORIENTED_EDGE('',*,*,#1902,.F.);
#2521=ORIENTED_EDGE('',*,*,#1903,.T.);
#2522=ORIENTED_EDGE('',*,*,#1904,.T.);
#2523=ORIENTED_EDGE('',*,*,#1900,.F.);
#2524=ORIENTED_EDGE('',*,*,#1905,.F.);
#2525=ORIENTED_EDGE('',*,*,#1906,.T.);
#2526=ORIENTED_EDGE('',*,*,#1907,.T.);
#2527=ORIENTED_EDGE('',*,*,#1903,.F.);
#2528=ORIENTED_EDGE('',*,*,#1908,.F.);
#2529=ORIENTED_EDGE('',*,*,#1909,.T.);
#2530=ORIENTED_EDGE('',*,*,#1910,.T.);
#2531=ORIENTED_EDGE('',*,*,#1906,.F.);
#2532=ORIENTED_EDGE('',*,*,#1911,.F.);
#2533=ORIENTED_EDGE('',*,*,#1912,.T.);
#2534=ORIENTED_EDGE('',*,*,#1913,.T.);
#2535=ORIENTED_EDGE('',*,*,#1909,.F.);
#2536=ORIENTED_EDGE('',*,*,#1914,.F.);
#2537=ORIENTED_EDGE('',*,*,#1915,.T.);
#2538=ORIENTED_EDGE('',*,*,#1916,.T.);
#2539=ORIENTED_EDGE('',*,*,#1912,.F.);
#2540=ORIENTED_EDGE('',*,*,#1917,.F.);
#2541=ORIENTED_EDGE('',*,*,#1918,.T.);
#2542=ORIENTED_EDGE('',*,*,#1919,.T.);
#2543=ORIENTED_EDGE('',*,*,#1915,.F.);
#2544=ORIENTED_EDGE('',*,*,#1920,.F.);
#2545=ORIENTED_EDGE('',*,*,#1921,.T.);
#2546=ORIENTED_EDGE('',*,*,#1922,.T.);
#2547=ORIENTED_EDGE('',*,*,#1918,.F.);
#2548=ORIENTED_EDGE('',*,*,#1923,.F.);
#2549=ORIENTED_EDGE('',*,*,#1924,.T.);
#2550=ORIENTED_EDGE('',*,*,#1925,.T.);
#2551=ORIENTED_EDGE('',*,*,#1921,.F.);
#2552=ORIENTED_EDGE('',*,*,#1926,.F.);
#2553=ORIENTED_EDGE('',*,*,#1927,.T.);
#2554=ORIENTED_EDGE('',*,*,#1928,.T.);
#2555=ORIENTED_EDGE('',*,*,#1924,.F.);
#2556=ORIENTED_EDGE('',*,*,#1929,.F.);
#2557=ORIENTED_EDGE('',*,*,#1930,.F.);
#2558=ORIENTED_EDGE('',*,*,#1931,.F.);
#2559=ORIENTED_EDGE('',*,*,#1932,.F.);
#2560=ORIENTED_EDGE('',*,*,#1933,.T.);
#2561=ORIENTED_EDGE('',*,*,#1934,.F.);
#2562=ORIENTED_EDGE('',*,*,#1935,.T.);
#2563=ORIENTED_EDGE('',*,*,#1936,.T.);
#2564=ORIENTED_EDGE('',*,*,#1935,.F.);
#2565=ORIENTED_EDGE('',*,*,#1936,.F.);
#2566=ORIENTED_EDGE('',*,*,#1937,.F.);
#2567=ORIENTED_EDGE('',*,*,#1938,.T.);
#2568=ORIENTED_EDGE('',*,*,#1939,.T.);
#2569=ORIENTED_EDGE('',*,*,#1938,.F.);
#2570=ORIENTED_EDGE('',*,*,#1939,.F.);
#2571=ORIENTED_EDGE('',*,*,#1848,.F.);
#2572=ORIENTED_EDGE('',*,*,#1940,.T.);
#2573=ORIENTED_EDGE('',*,*,#1892,.T.);
#2574=ORIENTED_EDGE('',*,*,#1941,.T.);
#2575=ORIENTED_EDGE('',*,*,#1930,.T.);
#2576=ORIENTED_EDGE('',*,*,#1942,.T.);
#2577=ORIENTED_EDGE('',*,*,#1927,.F.);
#2578=ORIENTED_EDGE('',*,*,#1943,.F.);
#2579=ORIENTED_EDGE('',*,*,#1941,.F.);
#2580=ORIENTED_EDGE('',*,*,#1891,.F.);
#2581=ORIENTED_EDGE('',*,*,#1895,.F.);
#2582=ORIENTED_EDGE('',*,*,#1898,.F.);
#2583=ORIENTED_EDGE('',*,*,#1901,.F.);
#2584=ORIENTED_EDGE('',*,*,#1904,.F.);
#2585=ORIENTED_EDGE('',*,*,#1907,.F.);
#2586=ORIENTED_EDGE('',*,*,#1910,.F.);
#2587=ORIENTED_EDGE('',*,*,#1913,.F.);
#2588=ORIENTED_EDGE('',*,*,#1916,.F.);
#2589=ORIENTED_EDGE('',*,*,#1919,.F.);
#2590=ORIENTED_EDGE('',*,*,#1922,.F.);
#2591=ORIENTED_EDGE('',*,*,#1925,.F.);
#2592=ORIENTED_EDGE('',*,*,#1928,.F.);
#2593=ORIENTED_EDGE('',*,*,#1942,.F.);
#2594=ORIENTED_EDGE('',*,*,#1933,.F.);
#2595=ORIENTED_EDGE('',*,*,#1944,.F.);
#2596=ORIENTED_EDGE('',*,*,#1887,.F.);
#2597=ORIENTED_EDGE('',*,*,#1945,.F.);
#2598=ORIENTED_EDGE('',*,*,#1885,.F.);
#2599=ORIENTED_EDGE('',*,*,#1882,.F.);
#2600=ORIENTED_EDGE('',*,*,#1879,.F.);
#2601=ORIENTED_EDGE('',*,*,#1876,.F.);
#2602=ORIENTED_EDGE('',*,*,#1873,.F.);
#2603=ORIENTED_EDGE('',*,*,#1870,.F.);
#2604=ORIENTED_EDGE('',*,*,#1867,.F.);
#2605=ORIENTED_EDGE('',*,*,#1864,.F.);
#2606=ORIENTED_EDGE('',*,*,#1861,.F.);
#2607=ORIENTED_EDGE('',*,*,#1858,.F.);
#2608=ORIENTED_EDGE('',*,*,#1855,.F.);
#2609=ORIENTED_EDGE('',*,*,#1852,.F.);
#2610=ORIENTED_EDGE('',*,*,#1849,.F.);
#2611=ORIENTED_EDGE('',*,*,#1940,.F.);
#2612=ORIENTED_EDGE('',*,*,#1847,.F.);
#2613=ORIENTED_EDGE('',*,*,#1854,.F.);
#2614=ORIENTED_EDGE('',*,*,#1857,.F.);
#2615=ORIENTED_EDGE('',*,*,#1860,.F.);
#2616=ORIENTED_EDGE('',*,*,#1863,.F.);
#2617=ORIENTED_EDGE('',*,*,#1866,.F.);
#2618=ORIENTED_EDGE('',*,*,#1869,.F.);
#2619=ORIENTED_EDGE('',*,*,#1872,.F.);
#2620=ORIENTED_EDGE('',*,*,#1875,.F.);
#2621=ORIENTED_EDGE('',*,*,#1878,.F.);
#2622=ORIENTED_EDGE('',*,*,#1881,.F.);
#2623=ORIENTED_EDGE('',*,*,#1884,.F.);
#2624=ORIENTED_EDGE('',*,*,#1946,.F.);
#2625=ORIENTED_EDGE('',*,*,#1889,.F.);
#2626=ORIENTED_EDGE('',*,*,#1947,.F.);
#2627=ORIENTED_EDGE('',*,*,#1931,.T.);
#2628=ORIENTED_EDGE('',*,*,#1943,.T.);
#2629=ORIENTED_EDGE('',*,*,#1929,.T.);
#2630=ORIENTED_EDGE('',*,*,#1926,.T.);
#2631=ORIENTED_EDGE('',*,*,#1923,.T.);
#2632=ORIENTED_EDGE('',*,*,#1920,.T.);
#2633=ORIENTED_EDGE('',*,*,#1917,.T.);
#2634=ORIENTED_EDGE('',*,*,#1914,.T.);
#2635=ORIENTED_EDGE('',*,*,#1911,.T.);
#2636=ORIENTED_EDGE('',*,*,#1908,.T.);
#2637=ORIENTED_EDGE('',*,*,#1905,.T.);
#2638=ORIENTED_EDGE('',*,*,#1902,.T.);
#2639=ORIENTED_EDGE('',*,*,#1899,.T.);
#2640=ORIENTED_EDGE('',*,*,#1896,.T.);
#2641=ORIENTED_EDGE('',*,*,#1893,.T.);
#2642=ORIENTED_EDGE('',*,*,#1886,.T.);
#2643=ORIENTED_EDGE('',*,*,#1946,.T.);
#2644=ORIENTED_EDGE('',*,*,#1883,.F.);
#2645=ORIENTED_EDGE('',*,*,#1945,.T.);
#2646=ORIENTED_EDGE('',*,*,#1760,.F.);
#2647=ORIENTED_EDGE('',*,*,#1948,.T.);
#2648=ORIENTED_EDGE('',*,*,#1804,.T.);
#2649=ORIENTED_EDGE('',*,*,#1949,.T.);
#2650=ORIENTED_EDGE('',*,*,#1842,.T.);
#2651=ORIENTED_EDGE('',*,*,#1950,.T.);
#2652=ORIENTED_EDGE('',*,*,#1839,.F.);
#2653=ORIENTED_EDGE('',*,*,#1951,.F.);
#2654=ORIENTED_EDGE('',*,*,#1949,.F.);
#2655=ORIENTED_EDGE('',*,*,#1803,.F.);
#2656=ORIENTED_EDGE('',*,*,#1807,.F.);
#2657=ORIENTED_EDGE('',*,*,#1810,.F.);
#2658=ORIENTED_EDGE('',*,*,#1813,.F.);
#2659=ORIENTED_EDGE('',*,*,#1816,.F.);
#2660=ORIENTED_EDGE('',*,*,#1819,.F.);
#2661=ORIENTED_EDGE('',*,*,#1822,.F.);
#2662=ORIENTED_EDGE('',*,*,#1825,.F.);
#2663=ORIENTED_EDGE('',*,*,#1828,.F.);
#2664=ORIENTED_EDGE('',*,*,#1831,.F.);
#2665=ORIENTED_EDGE('',*,*,#1834,.F.);
#2666=ORIENTED_EDGE('',*,*,#1837,.F.);
#2667=ORIENTED_EDGE('',*,*,#1840,.F.);
#2668=ORIENTED_EDGE('',*,*,#1950,.F.);
#2669=ORIENTED_EDGE('',*,*,#1845,.F.);
#2670=ORIENTED_EDGE('',*,*,#1952,.F.);
#2671=ORIENTED_EDGE('',*,*,#1799,.F.);
#2672=ORIENTED_EDGE('',*,*,#1953,.F.);
#2673=ORIENTED_EDGE('',*,*,#1797,.F.);
#2674=ORIENTED_EDGE('',*,*,#1794,.F.);
#2675=ORIENTED_EDGE('',*,*,#1791,.F.);
#2676=ORIENTED_EDGE('',*,*,#1788,.F.);
#2677=ORIENTED_EDGE('',*,*,#1785,.F.);
#2678=ORIENTED_EDGE('',*,*,#1782,.F.);
#2679=ORIENTED_EDGE('',*,*,#1779,.F.);
#2680=ORIENTED_EDGE('',*,*,#1776,.F.);
#2681=ORIENTED_EDGE('',*,*,#1773,.F.);
#2682=ORIENTED_EDGE('',*,*,#1770,.F.);
#2683=ORIENTED_EDGE('',*,*,#1767,.F.);
#2684=ORIENTED_EDGE('',*,*,#1764,.F.);
#2685=ORIENTED_EDGE('',*,*,#1761,.F.);
#2686=ORIENTED_EDGE('',*,*,#1948,.F.);
#2687=ORIENTED_EDGE('',*,*,#1759,.F.);
#2688=ORIENTED_EDGE('',*,*,#1766,.F.);
#2689=ORIENTED_EDGE('',*,*,#1769,.F.);
#2690=ORIENTED_EDGE('',*,*,#1772,.F.);
#2691=ORIENTED_EDGE('',*,*,#1775,.F.);
#2692=ORIENTED_EDGE('',*,*,#1778,.F.);
#2693=ORIENTED_EDGE('',*,*,#1781,.F.);
#2694=ORIENTED_EDGE('',*,*,#1784,.F.);
#2695=ORIENTED_EDGE('',*,*,#1787,.F.);
#2696=ORIENTED_EDGE('',*,*,#1790,.F.);
#2697=ORIENTED_EDGE('',*,*,#1793,.F.);
#2698=ORIENTED_EDGE('',*,*,#1796,.F.);
#2699=ORIENTED_EDGE('',*,*,#1954,.F.);
#2700=ORIENTED_EDGE('',*,*,#1801,.F.);
#2701=ORIENTED_EDGE('',*,*,#1955,.F.);
#2702=ORIENTED_EDGE('',*,*,#1843,.T.);
#2703=ORIENTED_EDGE('',*,*,#1951,.T.);
#2704=ORIENTED_EDGE('',*,*,#1841,.T.);
#2705=ORIENTED_EDGE('',*,*,#1838,.T.);
#2706=ORIENTED_EDGE('',*,*,#1835,.T.);
#2707=ORIENTED_EDGE('',*,*,#1832,.T.);
#2708=ORIENTED_EDGE('',*,*,#1829,.T.);
#2709=ORIENTED_EDGE('',*,*,#1826,.T.);
#2710=ORIENTED_EDGE('',*,*,#1823,.T.);
#2711=ORIENTED_EDGE('',*,*,#1820,.T.);
#2712=ORIENTED_EDGE('',*,*,#1817,.T.);
#2713=ORIENTED_EDGE('',*,*,#1814,.T.);
#2714=ORIENTED_EDGE('',*,*,#1811,.T.);
#2715=ORIENTED_EDGE('',*,*,#1808,.T.);
#2716=ORIENTED_EDGE('',*,*,#1805,.T.);
#2717=ORIENTED_EDGE('',*,*,#1798,.T.);
#2718=ORIENTED_EDGE('',*,*,#1954,.T.);
#2719=ORIENTED_EDGE('',*,*,#1795,.F.);
#2720=ORIENTED_EDGE('',*,*,#1953,.T.);
#2721=ORIENTED_EDGE('',*,*,#1763,.F.);
#2722=ORIENTED_EDGE('',*,*,#1851,.F.);
#2723=ORIENTED_EDGE('',*,*,#1956,.T.);
#2724=ORIENTED_EDGE('',*,*,#1957,.T.);
#2725=ORIENTED_EDGE('',*,*,#1958,.F.);
#2726=ORIENTED_EDGE('',*,*,#1959,.F.);
#2727=ORIENTED_EDGE('',*,*,#1960,.T.);
#2728=ORIENTED_EDGE('',*,*,#1959,.T.);
#2729=ORIENTED_EDGE('',*,*,#1961,.F.);
#2730=ORIENTED_EDGE('',*,*,#1962,.F.);
#2731=ORIENTED_EDGE('',*,*,#1963,.T.);
#2732=ORIENTED_EDGE('',*,*,#1962,.T.);
#2733=ORIENTED_EDGE('',*,*,#1964,.F.);
#2734=ORIENTED_EDGE('',*,*,#1965,.F.);
#2735=ORIENTED_EDGE('',*,*,#1966,.T.);
#2736=ORIENTED_EDGE('',*,*,#1965,.T.);
#2737=ORIENTED_EDGE('',*,*,#1967,.F.);
#2738=ORIENTED_EDGE('',*,*,#1968,.F.);
#2739=ORIENTED_EDGE('',*,*,#1969,.T.);
#2740=ORIENTED_EDGE('',*,*,#1968,.T.);
#2741=ORIENTED_EDGE('',*,*,#1970,.F.);
#2742=ORIENTED_EDGE('',*,*,#1971,.F.);
#2743=ORIENTED_EDGE('',*,*,#1972,.T.);
#2744=ORIENTED_EDGE('',*,*,#1971,.T.);
#2745=ORIENTED_EDGE('',*,*,#1973,.F.);
#2746=ORIENTED_EDGE('',*,*,#1974,.F.);
#2747=ORIENTED_EDGE('',*,*,#1975,.T.);
#2748=ORIENTED_EDGE('',*,*,#1974,.T.);
#2749=ORIENTED_EDGE('',*,*,#1976,.F.);
#2750=ORIENTED_EDGE('',*,*,#1977,.F.);
#2751=ORIENTED_EDGE('',*,*,#1978,.T.);
#2752=ORIENTED_EDGE('',*,*,#1977,.T.);
#2753=ORIENTED_EDGE('',*,*,#1979,.F.);
#2754=ORIENTED_EDGE('',*,*,#1957,.F.);
#2755=ORIENTED_EDGE('',*,*,#1980,.F.);
#2756=ORIENTED_EDGE('',*,*,#1981,.T.);
#2757=ORIENTED_EDGE('',*,*,#1982,.F.);
#2758=ORIENTED_EDGE('',*,*,#1983,.F.);
#2759=ORIENTED_EDGE('',*,*,#1984,.T.);
#2760=ORIENTED_EDGE('',*,*,#1983,.T.);
#2761=ORIENTED_EDGE('',*,*,#1985,.F.);
#2762=ORIENTED_EDGE('',*,*,#1986,.F.);
#2763=ORIENTED_EDGE('',*,*,#1987,.F.);
#2764=ORIENTED_EDGE('',*,*,#1986,.T.);
#2765=ORIENTED_EDGE('',*,*,#1988,.F.);
#2766=ORIENTED_EDGE('',*,*,#1989,.F.);
#2767=ORIENTED_EDGE('',*,*,#1990,.T.);
#2768=ORIENTED_EDGE('',*,*,#1989,.T.);
#2769=ORIENTED_EDGE('',*,*,#1991,.F.);
#2770=ORIENTED_EDGE('',*,*,#1992,.F.);
#2771=ORIENTED_EDGE('',*,*,#1993,.T.);
#2772=ORIENTED_EDGE('',*,*,#1992,.T.);
#2773=ORIENTED_EDGE('',*,*,#1994,.F.);
#2774=ORIENTED_EDGE('',*,*,#1995,.F.);
#2775=ORIENTED_EDGE('',*,*,#1996,.T.);
#2776=ORIENTED_EDGE('',*,*,#1995,.T.);
#2777=ORIENTED_EDGE('',*,*,#1997,.F.);
#2778=ORIENTED_EDGE('',*,*,#1998,.F.);
#2779=ORIENTED_EDGE('',*,*,#1999,.T.);
#2780=ORIENTED_EDGE('',*,*,#1998,.T.);
#2781=ORIENTED_EDGE('',*,*,#2000,.F.);
#2782=ORIENTED_EDGE('',*,*,#2001,.F.);
#2783=ORIENTED_EDGE('',*,*,#2002,.T.);
#2784=ORIENTED_EDGE('',*,*,#2001,.T.);
#2785=ORIENTED_EDGE('',*,*,#2003,.F.);
#2786=ORIENTED_EDGE('',*,*,#2004,.F.);
#2787=ORIENTED_EDGE('',*,*,#2005,.F.);
#2788=ORIENTED_EDGE('',*,*,#2004,.T.);
#2789=ORIENTED_EDGE('',*,*,#2006,.F.);
#2790=ORIENTED_EDGE('',*,*,#2007,.F.);
#2791=ORIENTED_EDGE('',*,*,#2008,.T.);
#2792=ORIENTED_EDGE('',*,*,#2007,.T.);
#2793=ORIENTED_EDGE('',*,*,#2009,.F.);
#2794=ORIENTED_EDGE('',*,*,#2010,.F.);
#2795=ORIENTED_EDGE('',*,*,#2011,.F.);
#2796=ORIENTED_EDGE('',*,*,#2010,.T.);
#2797=ORIENTED_EDGE('',*,*,#2012,.F.);
#2798=ORIENTED_EDGE('',*,*,#2013,.F.);
#2799=ORIENTED_EDGE('',*,*,#2014,.T.);
#2800=ORIENTED_EDGE('',*,*,#2013,.T.);
#2801=ORIENTED_EDGE('',*,*,#2015,.F.);
#2802=ORIENTED_EDGE('',*,*,#2016,.F.);
#2803=ORIENTED_EDGE('',*,*,#2017,.T.);
#2804=ORIENTED_EDGE('',*,*,#2016,.T.);
#2805=ORIENTED_EDGE('',*,*,#2018,.F.);
#2806=ORIENTED_EDGE('',*,*,#2019,.F.);
#2807=ORIENTED_EDGE('',*,*,#2020,.T.);
#2808=ORIENTED_EDGE('',*,*,#2019,.T.);
#2809=ORIENTED_EDGE('',*,*,#2021,.F.);
#2810=ORIENTED_EDGE('',*,*,#2022,.F.);
#2811=ORIENTED_EDGE('',*,*,#1934,.T.);
#2812=ORIENTED_EDGE('',*,*,#1937,.T.);
#2813=ORIENTED_EDGE('',*,*,#1947,.T.);
#2814=ORIENTED_EDGE('',*,*,#1888,.T.);
#2815=ORIENTED_EDGE('',*,*,#1944,.T.);
#2816=ORIENTED_EDGE('',*,*,#1932,.T.);
#2817=ORIENTED_EDGE('',*,*,#1955,.T.);
#2818=ORIENTED_EDGE('',*,*,#1800,.T.);
#2819=ORIENTED_EDGE('',*,*,#1952,.T.);
#2820=ORIENTED_EDGE('',*,*,#1844,.T.);
#2821=ORIENTED_EDGE('',*,*,#2023,.T.);
#2822=ORIENTED_EDGE('',*,*,#2022,.T.);
#2823=ORIENTED_EDGE('',*,*,#2024,.F.);
#2824=ORIENTED_EDGE('',*,*,#2025,.F.);
#2825=ORIENTED_EDGE('',*,*,#2026,.T.);
#2826=ORIENTED_EDGE('',*,*,#2025,.T.);
#2827=ORIENTED_EDGE('',*,*,#2027,.F.);
#2828=ORIENTED_EDGE('',*,*,#1981,.F.);
#2829=ORIENTED_EDGE('',*,*,#2027,.T.);
#2830=ORIENTED_EDGE('',*,*,#2024,.T.);
#2831=ORIENTED_EDGE('',*,*,#2021,.T.);
#2832=ORIENTED_EDGE('',*,*,#2018,.T.);
#2833=ORIENTED_EDGE('',*,*,#2015,.T.);
#2834=ORIENTED_EDGE('',*,*,#2012,.T.);
#2835=ORIENTED_EDGE('',*,*,#2009,.T.);
#2836=ORIENTED_EDGE('',*,*,#2006,.T.);
#2837=ORIENTED_EDGE('',*,*,#2003,.T.);
#2838=ORIENTED_EDGE('',*,*,#2000,.T.);
#2839=ORIENTED_EDGE('',*,*,#1997,.T.);
#2840=ORIENTED_EDGE('',*,*,#1994,.T.);
#2841=ORIENTED_EDGE('',*,*,#1991,.T.);
#2842=ORIENTED_EDGE('',*,*,#1988,.T.);
#2843=ORIENTED_EDGE('',*,*,#1985,.T.);
#2844=ORIENTED_EDGE('',*,*,#1982,.T.);
#2845=ORIENTED_EDGE('',*,*,#1979,.T.);
#2846=ORIENTED_EDGE('',*,*,#1976,.T.);
#2847=ORIENTED_EDGE('',*,*,#1973,.T.);
#2848=ORIENTED_EDGE('',*,*,#1970,.T.);
#2849=ORIENTED_EDGE('',*,*,#1967,.T.);
#2850=ORIENTED_EDGE('',*,*,#1964,.T.);
#2851=ORIENTED_EDGE('',*,*,#1961,.T.);
#2852=ORIENTED_EDGE('',*,*,#1958,.T.);
#2853=ORIENTED_EDGE('',*,*,#2026,.F.);
#2854=ORIENTED_EDGE('',*,*,#1980,.T.);
#2855=ORIENTED_EDGE('',*,*,#1984,.F.);
#2856=ORIENTED_EDGE('',*,*,#1987,.T.);
#2857=ORIENTED_EDGE('',*,*,#1990,.F.);
#2858=ORIENTED_EDGE('',*,*,#1993,.F.);
#2859=ORIENTED_EDGE('',*,*,#1996,.F.);
#2860=ORIENTED_EDGE('',*,*,#1999,.F.);
#2861=ORIENTED_EDGE('',*,*,#2002,.F.);
#2862=ORIENTED_EDGE('',*,*,#2005,.T.);
#2863=ORIENTED_EDGE('',*,*,#2008,.F.);
#2864=ORIENTED_EDGE('',*,*,#2011,.T.);
#2865=ORIENTED_EDGE('',*,*,#2014,.F.);
#2866=ORIENTED_EDGE('',*,*,#2017,.F.);
#2867=ORIENTED_EDGE('',*,*,#2020,.F.);
#2868=ORIENTED_EDGE('',*,*,#2023,.F.);
#2869=ORIENTED_EDGE('',*,*,#1978,.F.);
#2870=ORIENTED_EDGE('',*,*,#1956,.F.);
#2871=ORIENTED_EDGE('',*,*,#1960,.F.);
#2872=ORIENTED_EDGE('',*,*,#1963,.F.);
#2873=ORIENTED_EDGE('',*,*,#1966,.F.);
#2874=ORIENTED_EDGE('',*,*,#1969,.F.);
#2875=ORIENTED_EDGE('',*,*,#1972,.F.);
#2876=ORIENTED_EDGE('',*,*,#1975,.F.);
#3359=CYLINDRICAL_SURFACE('',#3803,2.117);
#3360=CYLINDRICAL_SURFACE('',#3806,2.117);
#3361=CYLINDRICAL_SURFACE('',#3807,2.117);
#3362=CYLINDRICAL_SURFACE('',#3808,2.117);
#3363=CYLINDRICAL_SURFACE('',#3809,2.117);
#3364=CYLINDRICAL_SURFACE('',#3810,2.117);
#3365=CYLINDRICAL_SURFACE('',#3811,2.117);
#3366=CYLINDRICAL_SURFACE('',#3812,2.117);
#3367=CYLINDRICAL_SURFACE('',#3813,2.117);
#3368=CYLINDRICAL_SURFACE('',#3814,2.117);
#3369=CYLINDRICAL_SURFACE('',#3815,2.117);
#3370=CYLINDRICAL_SURFACE('',#3816,2.117);
#3371=CYLINDRICAL_SURFACE('',#3817,2.117);
#3372=CYLINDRICAL_SURFACE('',#3819,2.56);
#3373=CYLINDRICAL_SURFACE('',#3821,2.56);
#3374=CYLINDRICAL_SURFACE('',#3822,2.56);
#3375=CYLINDRICAL_SURFACE('',#3823,2.56);
#3376=CYLINDRICAL_SURFACE('',#3824,2.56);
#3377=CYLINDRICAL_SURFACE('',#3825,2.56);
#3378=CYLINDRICAL_SURFACE('',#3826,2.56);
#3379=CYLINDRICAL_SURFACE('',#3827,2.56);
#3380=CYLINDRICAL_SURFACE('',#3828,2.56);
#3381=CYLINDRICAL_SURFACE('',#3829,2.56);
#3382=CYLINDRICAL_SURFACE('',#3830,2.56);
#3383=CYLINDRICAL_SURFACE('',#3831,2.56);
#3384=CYLINDRICAL_SURFACE('',#3832,2.56);
#3385=CYLINDRICAL_SURFACE('',#3833,2.56);
#3386=CYLINDRICAL_SURFACE('',#3835,2.117);
#3387=CYLINDRICAL_SURFACE('',#3838,2.117);
#3388=CYLINDRICAL_SURFACE('',#3839,2.117);
#3389=CYLINDRICAL_SURFACE('',#3840,2.117);
#3390=CYLINDRICAL_SURFACE('',#3841,2.117);
#3391=CYLINDRICAL_SURFACE('',#3842,2.117);
#3392=CYLINDRICAL_SURFACE('',#3843,2.117);
#3393=CYLINDRICAL_SURFACE('',#3844,2.117);
#3394=CYLINDRICAL_SURFACE('',#3845,2.117);
#3395=CYLINDRICAL_SURFACE('',#3846,2.117);
#3396=CYLINDRICAL_SURFACE('',#3847,2.117);
#3397=CYLINDRICAL_SURFACE('',#3848,2.117);
#3398=CYLINDRICAL_SURFACE('',#3849,2.117);
#3399=CYLINDRICAL_SURFACE('',#3851,2.56);
#3400=CYLINDRICAL_SURFACE('',#3853,2.56);
#3401=CYLINDRICAL_SURFACE('',#3854,2.56);
#3402=CYLINDRICAL_SURFACE('',#3855,2.56);
#3403=CYLINDRICAL_SURFACE('',#3856,2.56);
#3404=CYLINDRICAL_SURFACE('',#3857,2.56);
#3405=CYLINDRICAL_SURFACE('',#3858,2.56);
#3406=CYLINDRICAL_SURFACE('',#3859,2.56);
#3407=CYLINDRICAL_SURFACE('',#3860,2.56);
#3408=CYLINDRICAL_SURFACE('',#3861,2.56);
#3409=CYLINDRICAL_SURFACE('',#3862,2.56);
#3410=CYLINDRICAL_SURFACE('',#3863,2.56);
#3411=CYLINDRICAL_SURFACE('',#3864,2.56);
#3412=CYLINDRICAL_SURFACE('',#3865,2.56);
#3413=CYLINDRICAL_SURFACE('',#3867,1.);
#3414=CYLINDRICAL_SURFACE('',#3871,1.);
#3415=CYLINDRICAL_SURFACE('',#3876,2.56);
#3416=CYLINDRICAL_SURFACE('',#3877,2.117);
#3417=CYLINDRICAL_SURFACE('',#3879,2.56);
#3418=CYLINDRICAL_SURFACE('',#3880,2.117);
#3419=CYLINDRICAL_SURFACE('',#3884,1.99999999999999);
#3420=CYLINDRICAL_SURFACE('',#3888,1.99999999999999);
#3421=CYLINDRICAL_SURFACE('',#3892,2.);
#3422=CYLINDRICAL_SURFACE('',#3896,2.);
#3423=CYLINDRICAL_SURFACE('',#3899,2.);
#3424=CYLINDRICAL_SURFACE('',#3903,2.00000000000001);
#3425=CYLINDRICAL_SURFACE('',#3911,2.00000000000001);
#3426=CYLINDRICAL_SURFACE('',#3915,2.);
#3509=ADVANCED_FACE('',(#433),#3359,.F.);
#3510=ADVANCED_FACE('',(#434),#3360,.F.);
#3511=ADVANCED_FACE('',(#435),#3361,.F.);
#3512=ADVANCED_FACE('',(#436),#3362,.F.);
#3513=ADVANCED_FACE('',(#437),#3363,.F.);
#3514=ADVANCED_FACE('',(#438),#3364,.F.);
#3515=ADVANCED_FACE('',(#439),#3365,.F.);
#3516=ADVANCED_FACE('',(#440),#3366,.F.);
#3517=ADVANCED_FACE('',(#441),#3367,.F.);
#3518=ADVANCED_FACE('',(#442),#3368,.F.);
#3519=ADVANCED_FACE('',(#443),#3369,.F.);
#3520=ADVANCED_FACE('',(#444),#3370,.F.);
#3521=ADVANCED_FACE('',(#445),#3371,.F.);
#3522=ADVANCED_FACE('',(#446),#3372,.F.);
#3523=ADVANCED_FACE('',(#447),#3373,.F.);
#3524=ADVANCED_FACE('',(#448),#3374,.F.);
#3525=ADVANCED_FACE('',(#449),#3375,.F.);
#3526=ADVANCED_FACE('',(#450),#3376,.F.);
#3527=ADVANCED_FACE('',(#451),#3377,.F.);
#3528=ADVANCED_FACE('',(#452),#3378,.F.);
#3529=ADVANCED_FACE('',(#453),#3379,.F.);
#3530=ADVANCED_FACE('',(#454),#3380,.F.);
#3531=ADVANCED_FACE('',(#455),#3381,.F.);
#3532=ADVANCED_FACE('',(#456),#3382,.F.);
#3533=ADVANCED_FACE('',(#457),#3383,.F.);
#3534=ADVANCED_FACE('',(#458),#3384,.F.);
#3535=ADVANCED_FACE('',(#459),#3385,.F.);
#3536=ADVANCED_FACE('',(#460),#3386,.F.);
#3537=ADVANCED_FACE('',(#461),#3387,.F.);
#3538=ADVANCED_FACE('',(#462),#3388,.F.);
#3539=ADVANCED_FACE('',(#463),#3389,.F.);
#3540=ADVANCED_FACE('',(#464),#3390,.F.);
#3541=ADVANCED_FACE('',(#465),#3391,.F.);
#3542=ADVANCED_FACE('',(#466),#3392,.F.);
#3543=ADVANCED_FACE('',(#467),#3393,.F.);
#3544=ADVANCED_FACE('',(#468),#3394,.F.);
#3545=ADVANCED_FACE('',(#469),#3395,.F.);
#3546=ADVANCED_FACE('',(#470),#3396,.F.);
#3547=ADVANCED_FACE('',(#471),#3397,.F.);
#3548=ADVANCED_FACE('',(#472),#3398,.F.);
#3549=ADVANCED_FACE('',(#473),#3399,.F.);
#3550=ADVANCED_FACE('',(#474),#3400,.F.);
#3551=ADVANCED_FACE('',(#475),#3401,.F.);
#3552=ADVANCED_FACE('',(#476),#3402,.F.);
#3553=ADVANCED_FACE('',(#477),#3403,.F.);
#3554=ADVANCED_FACE('',(#478),#3404,.F.);
#3555=ADVANCED_FACE('',(#479),#3405,.F.);
#3556=ADVANCED_FACE('',(#480),#3406,.F.);
#3557=ADVANCED_FACE('',(#481),#3407,.F.);
#3558=ADVANCED_FACE('',(#482),#3408,.F.);
#3559=ADVANCED_FACE('',(#483),#3409,.F.);
#3560=ADVANCED_FACE('',(#484),#3410,.F.);
#3561=ADVANCED_FACE('',(#485),#3411,.F.);
#3562=ADVANCED_FACE('',(#486),#3412,.F.);
#3563=ADVANCED_FACE('',(#487),#3413,.F.);
#3564=ADVANCED_FACE('',(#488),#373,.F.);
#3565=ADVANCED_FACE('',(#489),#3414,.F.);
#3566=ADVANCED_FACE('',(#490),#374,.F.);
#3567=ADVANCED_FACE('',(#491),#375,.F.);
#3568=ADVANCED_FACE('',(#492),#3415,.F.);
#3569=ADVANCED_FACE('',(#493),#56,.F.);
#3570=ADVANCED_FACE('',(#494),#57,.F.);
#3571=ADVANCED_FACE('',(#495),#3416,.F.);
#3572=ADVANCED_FACE('',(#496),#376,.F.);
#3573=ADVANCED_FACE('',(#497),#3417,.F.);
#3574=ADVANCED_FACE('',(#498),#58,.F.);
#3575=ADVANCED_FACE('',(#499),#59,.F.);
#3576=ADVANCED_FACE('',(#500),#3418,.F.);
#3577=ADVANCED_FACE('',(#501),#377,.F.);
#3578=ADVANCED_FACE('',(#502),#378,.F.);
#3579=ADVANCED_FACE('',(#503),#379,.T.);
#3580=ADVANCED_FACE('',(#504),#3419,.F.);
#3581=ADVANCED_FACE('',(#505),#380,.T.);
#3582=ADVANCED_FACE('',(#506),#3420,.F.);
#3583=ADVANCED_FACE('',(#507),#381,.T.);
#3584=ADVANCED_FACE('',(#508),#3421,.F.);
#3585=ADVANCED_FACE('',(#509),#382,.T.);
#3586=ADVANCED_FACE('',(#510),#3422,.F.);
#3587=ADVANCED_FACE('',(#511),#3423,.F.);
#3588=ADVANCED_FACE('',(#512),#383,.T.);
#3589=ADVANCED_FACE('',(#513),#3424,.F.);
#3590=ADVANCED_FACE('',(#514),#384,.T.);
#3591=ADVANCED_FACE('',(#515),#385,.T.);
#3592=ADVANCED_FACE('',(#516),#386,.T.);
#3593=ADVANCED_FACE('',(#517),#387,.T.);
#3594=ADVANCED_FACE('',(#518),#388,.T.);
#3595=ADVANCED_FACE('',(#519),#3425,.F.);
#3596=ADVANCED_FACE('',(#520),#389,.T.);
#3597=ADVANCED_FACE('',(#521),#3426,.F.);
#3598=ADVANCED_FACE('',(#522),#390,.T.);
#3599=ADVANCED_FACE('',(#523),#391,.T.);
#3600=ADVANCED_FACE('',(#524,#355,#356,#357,#358),#392,.T.);
#3601=ADVANCED_FACE('',(#525),#393,.T.);
#3602=ADVANCED_FACE('',(#526),#394,.T.);
#3603=ADVANCED_FACE('',(#527,#359),#395,.T.);
#3604=ADVANCED_FACE('',(#528,#360),#396,.F.);
#3695=CLOSED_SHELL('',(#3509,#3510,#3511,#3512,#3513,#3514,#3515,#3516,
#3517,#3518,#3519,#3520,#3521,#3522,#3523,#3524,#3525,#3526,#3527,#3528,
#3529,#3530,#3531,#3532,#3533,#3534,#3535,#3536,#3537,#3538,#3539,#3540,
#3541,#3542,#3543,#3544,#3545,#3546,#3547,#3548,#3549,#3550,#3551,#3552,
#3553,#3554,#3555,#3556,#3557,#3558,#3559,#3560,#3561,#3562,#3563,#3564,
#3565,#3566,#3567,#3568,#3569,#3570,#3571,#3572,#3573,#3574,#3575,#3576,
#3577,#3578,#3579,#3580,#3581,#3582,#3583,#3584,#3585,#3586,#3587,#3588,
#3589,#3590,#3591,#3592,#3593,#3594,#3595,#3596,#3597,#3598,#3599,#3600,
#3601,#3602,#3603,#3604));
#3802=AXIS2_PLACEMENT_3D('',#4894,#4130,#4131);
#3803=AXIS2_PLACEMENT_3D('',#4895,#4132,#4133);
#3804=AXIS2_PLACEMENT_3D('',#4920,#4135,#4136);
#3805=AXIS2_PLACEMENT_3D('',#4928,#4138,#4139);
#3806=AXIS2_PLACEMENT_3D('',#4954,#4140,#4141);
#3807=AXIS2_PLACEMENT_3D('',#5002,#4143,#4144);
#3808=AXIS2_PLACEMENT_3D('',#5053,#4146,#4147);
#3809=AXIS2_PLACEMENT_3D('',#5104,#4149,#4150);
#3810=AXIS2_PLACEMENT_3D('',#5152,#4152,#4153);
#3811=AXIS2_PLACEMENT_3D('',#5203,#4155,#4156);
#3812=AXIS2_PLACEMENT_3D('',#5254,#4158,#4159);
#3813=AXIS2_PLACEMENT_3D('',#5302,#4161,#4162);
#3814=AXIS2_PLACEMENT_3D('',#5353,#4164,#4165);
#3815=AXIS2_PLACEMENT_3D('',#5404,#4167,#4168);
#3816=AXIS2_PLACEMENT_3D('',#5452,#4170,#4171);
#3817=AXIS2_PLACEMENT_3D('',#5503,#4173,#4174);
#3818=AXIS2_PLACEMENT_3D('',#5522,#4176,#4177);
#3819=AXIS2_PLACEMENT_3D('',#5542,#4178,#4179);
#3820=AXIS2_PLACEMENT_3D('',#5554,#4181,#4182);
#3821=AXIS2_PLACEMENT_3D('',#5562,#4183,#4184);
#3822=AXIS2_PLACEMENT_3D('',#5587,#4186,#4187);
#3823=AXIS2_PLACEMENT_3D('',#5612,#4189,#4190);
#3824=AXIS2_PLACEMENT_3D('',#5636,#4192,#4193);
#3825=AXIS2_PLACEMENT_3D('',#5661,#4195,#4196);
#3826=AXIS2_PLACEMENT_3D('',#5686,#4198,#4199);
#3827=AXIS2_PLACEMENT_3D('',#5710,#4201,#4202);
#3828=AXIS2_PLACEMENT_3D('',#5735,#4204,#4205);
#3829=AXIS2_PLACEMENT_3D('',#5760,#4207,#4208);
#3830=AXIS2_PLACEMENT_3D('',#5784,#4210,#4211);
#3831=AXIS2_PLACEMENT_3D('',#5809,#4213,#4214);
#3832=AXIS2_PLACEMENT_3D('',#5834,#4216,#4217);
#3833=AXIS2_PLACEMENT_3D('',#5858,#4219,#4220);
#3834=AXIS2_PLACEMENT_3D('',#5869,#4222,#4223);
#3835=AXIS2_PLACEMENT_3D('',#5875,#4224,#4225);
#3836=AXIS2_PLACEMENT_3D('',#5900,#4227,#4228);
#3837=AXIS2_PLACEMENT_3D('',#5908,#4230,#4231);
#3838=AXIS2_PLACEMENT_3D('',#5934,#4232,#4233);
#3839=AXIS2_PLACEMENT_3D('',#5982,#4235,#4236);
#3840=AXIS2_PLACEMENT_3D('',#6033,#4238,#4239);
#3841=AXIS2_PLACEMENT_3D('',#6084,#4241,#4242);
#3842=AXIS2_PLACEMENT_3D('',#6132,#4244,#4245);
#3843=AXIS2_PLACEMENT_3D('',#6183,#4247,#4248);
#3844=AXIS2_PLACEMENT_3D('',#6234,#4250,#4251);
#3845=AXIS2_PLACEMENT_3D('',#6282,#4253,#4254);
#3846=AXIS2_PLACEMENT_3D('',#6333,#4256,#4257);
#3847=AXIS2_PLACEMENT_3D('',#6384,#4259,#4260);
#3848=AXIS2_PLACEMENT_3D('',#6432,#4262,#4263);
#3849=AXIS2_PLACEMENT_3D('',#6483,#4265,#4266);
#3850=AXIS2_PLACEMENT_3D('',#6502,#4268,#4269);
#3851=AXIS2_PLACEMENT_3D('',#6522,#4270,#4271);
#3852=AXIS2_PLACEMENT_3D('',#6534,#4273,#4274);
#3853=AXIS2_PLACEMENT_3D('',#6542,#4275,#4276);
#3854=AXIS2_PLACEMENT_3D('',#6567,#4278,#4279);
#3855=AXIS2_PLACEMENT_3D('',#6592,#4281,#4282);
#3856=AXIS2_PLACEMENT_3D('',#6616,#4284,#4285);
#3857=AXIS2_PLACEMENT_3D('',#6641,#4287,#4288);
#3858=AXIS2_PLACEMENT_3D('',#6666,#4290,#4291);
#3859=AXIS2_PLACEMENT_3D('',#6690,#4293,#4294);
#3860=AXIS2_PLACEMENT_3D('',#6715,#4296,#4297);
#3861=AXIS2_PLACEMENT_3D('',#6740,#4299,#4300);
#3862=AXIS2_PLACEMENT_3D('',#6764,#4302,#4303);
#3863=AXIS2_PLACEMENT_3D('',#6789,#4305,#4306);
#3864=AXIS2_PLACEMENT_3D('',#6814,#4308,#4309);
#3865=AXIS2_PLACEMENT_3D('',#6838,#4311,#4312);
#3866=AXIS2_PLACEMENT_3D('',#6849,#4314,#4315);
#3867=AXIS2_PLACEMENT_3D('',#6855,#4316,#4317);
#3868=AXIS2_PLACEMENT_3D('',#6857,#4318,#4319);
#3869=AXIS2_PLACEMENT_3D('',#6860,#4321,#4322);
#3870=AXIS2_PLACEMENT_3D('',#6861,#4323,#4324);
#3871=AXIS2_PLACEMENT_3D('',#6862,#4325,#4326);
#3872=AXIS2_PLACEMENT_3D('',#6864,#4327,#4328);
#3873=AXIS2_PLACEMENT_3D('',#6867,#4330,#4331);
#3874=AXIS2_PLACEMENT_3D('',#6868,#4332,#4333);
#3875=AXIS2_PLACEMENT_3D('',#6869,#4334,#4335);
#3876=AXIS2_PLACEMENT_3D('',#7049,#4336,#4337);
#3877=AXIS2_PLACEMENT_3D('',#8036,#4338,#4339);
#3878=AXIS2_PLACEMENT_3D('',#8037,#4340,#4341);
#3879=AXIS2_PLACEMENT_3D('',#8217,#4342,#4343);
#3880=AXIS2_PLACEMENT_3D('',#9204,#4344,#4345);
#3881=AXIS2_PLACEMENT_3D('',#9205,#4346,#4347);
#3882=AXIS2_PLACEMENT_3D('',#9206,#4348,#4349);
#3883=AXIS2_PLACEMENT_3D('',#9207,#4350,#4351);
#3884=AXIS2_PLACEMENT_3D('',#9216,#4356,#4357);
#3885=AXIS2_PLACEMENT_3D('',#9218,#4358,#4359);
#3886=AXIS2_PLACEMENT_3D('',#9220,#4360,#4361);
#3887=AXIS2_PLACEMENT_3D('',#9222,#4363,#4364);
#3888=AXIS2_PLACEMENT_3D('',#9228,#4368,#4369);
#3889=AXIS2_PLACEMENT_3D('',#9230,#4370,#4371);
#3890=AXIS2_PLACEMENT_3D('',#9232,#4372,#4373);
#3891=AXIS2_PLACEMENT_3D('',#9234,#4375,#4376);
#3892=AXIS2_PLACEMENT_3D('',#9240,#4380,#4381);
#3893=AXIS2_PLACEMENT_3D('',#9242,#4382,#4383);
#3894=AXIS2_PLACEMENT_3D('',#9244,#4384,#4385);
#3895=AXIS2_PLACEMENT_3D('',#9246,#4387,#4388);
#3896=AXIS2_PLACEMENT_3D('',#9252,#4392,#4393);
#3897=AXIS2_PLACEMENT_3D('',#9253,#4394,#4395);
#3898=AXIS2_PLACEMENT_3D('',#9254,#4396,#4397);
#3899=AXIS2_PLACEMENT_3D('',#9255,#4398,#4399);
#3900=AXIS2_PLACEMENT_3D('',#9258,#4400,#4401);
#3901=AXIS2_PLACEMENT_3D('',#9262,#4403,#4404);
#3902=AXIS2_PLACEMENT_3D('',#9264,#4406,#4407);
#3903=AXIS2_PLACEMENT_3D('',#9270,#4411,#4412);
#3904=AXIS2_PLACEMENT_3D('',#9272,#4413,#4414);
#3905=AXIS2_PLACEMENT_3D('',#9274,#4415,#4416);
#3906=AXIS2_PLACEMENT_3D('',#9276,#4418,#4419);
#3907=AXIS2_PLACEMENT_3D('',#9282,#4423,#4424);
#3908=AXIS2_PLACEMENT_3D('',#9288,#4428,#4429);
#3909=AXIS2_PLACEMENT_3D('',#9294,#4433,#4434);
#3910=AXIS2_PLACEMENT_3D('',#9300,#4438,#4439);
#3911=AXIS2_PLACEMENT_3D('',#9306,#4443,#4444);
#3912=AXIS2_PLACEMENT_3D('',#9308,#4445,#4446);
#3913=AXIS2_PLACEMENT_3D('',#9310,#4447,#4448);
#3914=AXIS2_PLACEMENT_3D('',#9312,#4450,#4451);
#3915=AXIS2_PLACEMENT_3D('',#9318,#4455,#4456);
#3916=AXIS2_PLACEMENT_3D('',#9320,#4457,#4458);
#3917=AXIS2_PLACEMENT_3D('',#9322,#4459,#4460);
#3918=AXIS2_PLACEMENT_3D('',#9324,#4462,#4463);
#3919=AXIS2_PLACEMENT_3D('',#9330,#4467,#4468);
#3920=AXIS2_PLACEMENT_3D('',#9336,#4472,#4473);
#3921=AXIS2_PLACEMENT_3D('',#9342,#4477,#4478);
#3922=AXIS2_PLACEMENT_3D('',#9348,#4482,#4483);
#3923=AXIS2_PLACEMENT_3D('',#9351,#4486,#4487);
#3924=AXIS2_PLACEMENT_3D('',#9352,#4488,#4489);
#4130=DIRECTION('axis',(0.,0.,1.));
#4131=DIRECTION('refdir',(1.,0.,0.));
#4132=DIRECTION('center_axis',(1.,0.,0.));
#4133=DIRECTION('ref_axis',(0.,-1.,0.));
#4134=DIRECTION('',(1.,0.,0.));
#4135=DIRECTION('center_axis',(-1.,0.,0.));
#4136=DIRECTION('ref_axis',(0.,-1.,0.));
#4137=DIRECTION('',(1.,0.,0.));
#4138=DIRECTION('center_axis',(-1.,0.,0.));
#4139=DIRECTION('ref_axis',(0.,-1.,0.));
#4140=DIRECTION('center_axis',(1.,0.,0.));
#4141=DIRECTION('ref_axis',(0.,-1.,0.));
#4142=DIRECTION('',(1.,0.,0.));
#4143=DIRECTION('center_axis',(1.,0.,0.));
#4144=DIRECTION('ref_axis',(0.,-1.,0.));
#4145=DIRECTION('',(1.,0.,0.));
#4146=DIRECTION('center_axis',(1.,0.,0.));
#4147=DIRECTION('ref_axis',(0.,-1.,0.));
#4148=DIRECTION('',(1.,0.,0.));
#4149=DIRECTION('center_axis',(1.,0.,0.));
#4150=DIRECTION('ref_axis',(0.,-1.,0.));
#4151=DIRECTION('',(1.,0.,0.));
#4152=DIRECTION('center_axis',(1.,0.,0.));
#4153=DIRECTION('ref_axis',(0.,-1.,0.));
#4154=DIRECTION('',(1.,0.,0.));
#4155=DIRECTION('center_axis',(1.,0.,0.));
#4156=DIRECTION('ref_axis',(0.,-1.,0.));
#4157=DIRECTION('',(1.,0.,0.));
#4158=DIRECTION('center_axis',(1.,0.,0.));
#4159=DIRECTION('ref_axis',(0.,-1.,0.));
#4160=DIRECTION('',(1.,0.,0.));
#4161=DIRECTION('center_axis',(1.,0.,0.));
#4162=DIRECTION('ref_axis',(0.,-1.,0.));
#4163=DIRECTION('',(1.,0.,0.));
#4164=DIRECTION('center_axis',(1.,0.,0.));
#4165=DIRECTION('ref_axis',(0.,-1.,0.));
#4166=DIRECTION('',(1.,0.,0.));
#4167=DIRECTION('center_axis',(1.,0.,0.));
#4168=DIRECTION('ref_axis',(0.,-1.,0.));
#4169=DIRECTION('',(1.,0.,0.));
#4170=DIRECTION('center_axis',(1.,0.,0.));
#4171=DIRECTION('ref_axis',(0.,-1.,0.));
#4172=DIRECTION('',(1.,0.,0.));
#4173=DIRECTION('center_axis',(1.,0.,0.));
#4174=DIRECTION('ref_axis',(0.,-0.939363391024623,-0.342923343624668));
#4175=DIRECTION('',(1.,0.,0.));
#4176=DIRECTION('center_axis',(1.,0.,0.));
#4177=DIRECTION('ref_axis',(0.,-1.,0.));
#4178=DIRECTION('center_axis',(1.,0.,0.));
#4179=DIRECTION('ref_axis',(0.,-0.130100013837605,0.991500875642304));
#4180=DIRECTION('',(1.,-1.22464679914735E-16,-9.41444059745064E-30));
#4181=DIRECTION('center_axis',(-1.,0.,0.));
#4182=DIRECTION('ref_axis',(0.,-1.,-7.67522767067882E-14));
#4183=DIRECTION('center_axis',(1.,0.,0.));
#4184=DIRECTION('ref_axis',(0.,-1.,-7.67522767067882E-14));
#4185=DIRECTION('',(1.,-1.22464679914735E-16,-9.41444059745064E-30));
#4186=DIRECTION('center_axis',(1.,0.,0.));
#4187=DIRECTION('ref_axis',(0.,-1.,-7.67522767067882E-14));
#4188=DIRECTION('',(1.,-1.22464679914735E-16,-9.41444059745064E-30));
#4189=DIRECTION('center_axis',(1.,0.,0.));
#4190=DIRECTION('ref_axis',(0.,-1.,-7.67522767067882E-14));
#4191=DIRECTION('',(1.,-1.22464679914735E-16,-9.41444059745064E-30));
#4192=DIRECTION('center_axis',(1.,0.,0.));
#4193=DIRECTION('ref_axis',(0.,-1.,-7.67522767067882E-14));
#4194=DIRECTION('',(1.,-1.22464679914735E-16,-9.41444059745064E-30));
#4195=DIRECTION('center_axis',(1.,0.,0.));
#4196=DIRECTION('ref_axis',(0.,-1.,-7.67522767067882E-14));
#4197=DIRECTION('',(1.,-1.22464679914735E-16,-9.41444059745064E-30));
#4198=DIRECTION('center_axis',(1.,0.,0.));
#4199=DIRECTION('ref_axis',(0.,-1.,-7.67522767067882E-14));
#4200=DIRECTION('',(1.,-1.22464679914735E-16,-9.41444059745064E-30));
#4201=DIRECTION('center_axis',(1.,0.,0.));
#4202=DIRECTION('ref_axis',(0.,-1.,-7.67522767067882E-14));
#4203=DIRECTION('',(1.,-1.22464679914735E-16,-9.41444059745064E-30));
#4204=DIRECTION('center_axis',(1.,0.,0.));
#4205=DIRECTION('ref_axis',(0.,-1.,-7.67522767067882E-14));
#4206=DIRECTION('',(1.,-1.22464679914735E-16,-9.41444059745064E-30));
#4207=DIRECTION('center_axis',(1.,0.,0.));
#4208=DIRECTION('ref_axis',(0.,-1.,-7.67522767067882E-14));
#4209=DIRECTION('',(1.,-1.22464679914735E-16,-9.41444059745064E-30));
#4210=DIRECTION('center_axis',(1.,0.,0.));
#4211=DIRECTION('ref_axis',(0.,-1.,-7.67522767067882E-14));
#4212=DIRECTION('',(1.,-1.22464679914735E-16,-9.41444059745064E-30));
#4213=DIRECTION('center_axis',(1.,0.,0.));
#4214=DIRECTION('ref_axis',(0.,-1.,-7.67522767067882E-14));
#4215=DIRECTION('',(1.,-1.22464679914735E-16,-9.41444059745064E-30));
#4216=DIRECTION('center_axis',(1.,0.,0.));
#4217=DIRECTION('ref_axis',(0.,-1.,-7.67522767067882E-14));
#4218=DIRECTION('',(1.,-1.22464679914735E-16,-9.41444059745064E-30));
#4219=DIRECTION('center_axis',(1.,0.,0.));
#4220=DIRECTION('ref_axis',(0.,0.609130550517291,-0.793069966917486));
#4221=DIRECTION('',(1.,-1.22464679914735E-16,-9.41444059745064E-30));
#4222=DIRECTION('center_axis',(1.,0.,0.));
#4223=DIRECTION('ref_axis',(0.,-1.,-7.67522767067882E-14));
#4224=DIRECTION('center_axis',(1.,0.,0.));
#4225=DIRECTION('ref_axis',(0.,-1.,0.));
#4226=DIRECTION('',(1.,0.,0.));
#4227=DIRECTION('center_axis',(-1.,0.,0.));
#4228=DIRECTION('ref_axis',(0.,-1.,0.));
#4229=DIRECTION('',(1.,0.,0.));
#4230=DIRECTION('center_axis',(-1.,0.,0.));
#4231=DIRECTION('ref_axis',(0.,-1.,0.));
#4232=DIRECTION('center_axis',(1.,0.,0.));
#4233=DIRECTION('ref_axis',(0.,-1.,0.));
#4234=DIRECTION('',(1.,0.,0.));
#4235=DIRECTION('center_axis',(1.,0.,0.));
#4236=DIRECTION('ref_axis',(0.,-1.,0.));
#4237=DIRECTION('',(1.,0.,0.));
#4238=DIRECTION('center_axis',(1.,0.,0.));
#4239=DIRECTION('ref_axis',(0.,-1.,0.));
#4240=DIRECTION('',(1.,0.,0.));
#4241=DIRECTION('center_axis',(1.,0.,0.));
#4242=DIRECTION('ref_axis',(0.,-1.,0.));
#4243=DIRECTION('',(1.,0.,0.));
#4244=DIRECTION('center_axis',(1.,0.,0.));
#4245=DIRECTION('ref_axis',(0.,-1.,0.));
#4246=DIRECTION('',(1.,0.,0.));
#4247=DIRECTION('center_axis',(1.,0.,0.));
#4248=DIRECTION('ref_axis',(0.,-1.,0.));
#4249=DIRECTION('',(1.,0.,0.));
#4250=DIRECTION('center_axis',(1.,0.,0.));
#4251=DIRECTION('ref_axis',(0.,-1.,0.));
#4252=DIRECTION('',(1.,0.,0.));
#4253=DIRECTION('center_axis',(1.,0.,0.));
#4254=DIRECTION('ref_axis',(0.,-1.,0.));
#4255=DIRECTION('',(1.,0.,0.));
#4256=DIRECTION('center_axis',(1.,0.,0.));
#4257=DIRECTION('ref_axis',(0.,-1.,0.));
#4258=DIRECTION('',(1.,0.,0.));
#4259=DIRECTION('center_axis',(1.,0.,0.));
#4260=DIRECTION('ref_axis',(0.,-1.,0.));
#4261=DIRECTION('',(1.,0.,0.));
#4262=DIRECTION('center_axis',(1.,0.,0.));
#4263=DIRECTION('ref_axis',(0.,-1.,0.));
#4264=DIRECTION('',(1.,0.,0.));
#4265=DIRECTION('center_axis',(1.,0.,0.));
#4266=DIRECTION('ref_axis',(0.,-0.939363407112957,-0.342923299554197));
#4267=DIRECTION('',(1.,0.,0.));
#4268=DIRECTION('center_axis',(1.,0.,0.));
#4269=DIRECTION('ref_axis',(0.,-1.,0.));
#4270=DIRECTION('center_axis',(1.,0.,0.));
#4271=DIRECTION('ref_axis',(0.,-0.130100058958222,0.991500869721791));
#4272=DIRECTION('',(1.,-1.22464679914735E-16,-9.41427121902906E-30));
#4273=DIRECTION('center_axis',(-1.,0.,0.));
#4274=DIRECTION('ref_axis',(0.,-1.,-7.67508936270162E-14));
#4275=DIRECTION('center_axis',(1.,0.,0.));
#4276=DIRECTION('ref_axis',(0.,-1.,-7.67508936270162E-14));
#4277=DIRECTION('',(1.,-1.22464679914735E-16,-9.41427121902906E-30));
#4278=DIRECTION('center_axis',(1.,0.,0.));
#4279=DIRECTION('ref_axis',(0.,-1.,-7.67508936270162E-14));
#4280=DIRECTION('',(1.,-1.22464679914735E-16,-9.41427121902906E-30));
#4281=DIRECTION('center_axis',(1.,0.,0.));
#4282=DIRECTION('ref_axis',(0.,-1.,-7.67508936270162E-14));
#4283=DIRECTION('',(1.,-1.22464679914735E-16,-9.41427121902906E-30));
#4284=DIRECTION('center_axis',(1.,0.,0.));
#4285=DIRECTION('ref_axis',(0.,-1.,-7.67508936270162E-14));
#4286=DIRECTION('',(1.,-1.22464679914735E-16,-9.41427121902906E-30));
#4287=DIRECTION('center_axis',(1.,0.,0.));
#4288=DIRECTION('ref_axis',(0.,-1.,-7.67508936270162E-14));
#4289=DIRECTION('',(1.,-1.22464679914735E-16,-9.41427121902906E-30));
#4290=DIRECTION('center_axis',(1.,0.,0.));
#4291=DIRECTION('ref_axis',(0.,-1.,-7.67508936270162E-14));
#4292=DIRECTION('',(1.,-1.22464679914735E-16,-9.41427121902906E-30));
#4293=DIRECTION('center_axis',(1.,0.,0.));
#4294=DIRECTION('ref_axis',(0.,-1.,-7.67508936270162E-14));
#4295=DIRECTION('',(1.,-1.22464679914735E-16,-9.41427121902906E-30));
#4296=DIRECTION('center_axis',(1.,0.,0.));
#4297=DIRECTION('ref_axis',(0.,-1.,-7.67508936270162E-14));
#4298=DIRECTION('',(1.,-1.22464679914735E-16,-9.41427121902906E-30));
#4299=DIRECTION('center_axis',(1.,0.,0.));
#4300=DIRECTION('ref_axis',(0.,-1.,-7.67508936270162E-14));
#4301=DIRECTION('',(1.,-1.22464679914735E-16,-9.41427121902906E-30));
#4302=DIRECTION('center_axis',(1.,0.,0.));
#4303=DIRECTION('ref_axis',(0.,-1.,-7.67508936270162E-14));
#4304=DIRECTION('',(1.,-1.22464679914735E-16,-9.41427121902906E-30));
#4305=DIRECTION('center_axis',(1.,0.,0.));
#4306=DIRECTION('ref_axis',(0.,-1.,-7.67508936270162E-14));
#4307=DIRECTION('',(1.,-1.22464679914735E-16,-9.41427121902906E-30));
#4308=DIRECTION('center_axis',(1.,0.,0.));
#4309=DIRECTION('ref_axis',(0.,-1.,-7.67508936270162E-14));
#4310=DIRECTION('',(1.,-1.22464679914735E-16,-9.41427121902906E-30));
#4311=DIRECTION('center_axis',(1.,0.,0.));
#4312=DIRECTION('ref_axis',(0.,0.609130584443187,-0.793069940860137));
#4313=DIRECTION('',(1.,-1.22464679914735E-16,-9.41427121902906E-30));
#4314=DIRECTION('center_axis',(1.,0.,0.));
#4315=DIRECTION('ref_axis',(0.,-1.,-7.67508936270162E-14));
#4316=DIRECTION('center_axis',(1.,0.,0.));
#4317=DIRECTION('ref_axis',(0.,-1.,0.));
#4318=DIRECTION('center_axis',(1.,0.,0.));
#4319=DIRECTION('ref_axis',(0.,-1.,0.));
#4320=DIRECTION('',(1.,0.,0.));
#4321=DIRECTION('center_axis',(1.,0.,0.));
#4322=DIRECTION('ref_axis',(0.,-1.,0.));
#4323=DIRECTION('center_axis',(1.,0.,0.));
#4324=DIRECTION('ref_axis',(0.,-1.,0.));
#4325=DIRECTION('center_axis',(1.,0.,0.));
#4326=DIRECTION('ref_axis',(0.,-1.,0.));
#4327=DIRECTION('center_axis',(1.,0.,0.));
#4328=DIRECTION('ref_axis',(0.,-1.,0.));
#4329=DIRECTION('',(1.,0.,0.));
#4330=DIRECTION('center_axis',(1.,0.,0.));
#4331=DIRECTION('ref_axis',(0.,-1.,0.));
#4332=DIRECTION('center_axis',(1.,0.,0.));
#4333=DIRECTION('ref_axis',(0.,-1.,0.));
#4334=DIRECTION('center_axis',(1.,0.,0.));
#4335=DIRECTION('ref_axis',(0.,0.,-1.));
#4336=DIRECTION('center_axis',(1.,0.,0.));
#4337=DIRECTION('ref_axis',(0.,-1.,-7.67508936270162E-14));
#4338=DIRECTION('center_axis',(1.,0.,0.));
#4339=DIRECTION('ref_axis',(0.,-1.,0.));
#4340=DIRECTION('center_axis',(1.,0.,0.));
#4341=DIRECTION('ref_axis',(0.,0.,-1.));
#4342=DIRECTION('center_axis',(1.,0.,0.));
#4343=DIRECTION('ref_axis',(0.,-1.,-7.67522767067882E-14));
#4344=DIRECTION('center_axis',(1.,0.,0.));
#4345=DIRECTION('ref_axis',(0.,-1.,0.));
#4346=DIRECTION('center_axis',(1.,0.,0.));
#4347=DIRECTION('ref_axis',(0.,-1.,0.));
#4348=DIRECTION('center_axis',(1.,0.,0.));
#4349=DIRECTION('ref_axis',(0.,-1.,0.));
#4350=DIRECTION('center_axis',(0.,1.,0.));
#4351=DIRECTION('ref_axis',(-1.,0.,0.));
#4352=DIRECTION('',(-1.,0.,0.));
#4353=DIRECTION('',(0.,0.,1.));
#4354=DIRECTION('',(-1.,0.,0.));
#4355=DIRECTION('',(0.,0.,1.));
#4356=DIRECTION('center_axis',(0.,0.,1.));
#4357=DIRECTION('ref_axis',(0.,-1.,0.));
#4358=DIRECTION('center_axis',(0.,0.,-1.));
#4359=DIRECTION('ref_axis',(0.,-1.,0.));
#4360=DIRECTION('center_axis',(0.,0.,-1.));
#4361=DIRECTION('ref_axis',(0.,-1.,0.));
#4362=DIRECTION('',(0.,0.,1.));
#4363=DIRECTION('center_axis',(-1.,0.,0.));
#4364=DIRECTION('ref_axis',(0.,-1.,0.));
#4365=DIRECTION('',(0.,-1.,0.));
#4366=DIRECTION('',(0.,-1.,0.));
#4367=DIRECTION('',(0.,0.,1.));
#4368=DIRECTION('center_axis',(0.,0.,1.));
#4369=DIRECTION('ref_axis',(1.,-3.33066907387548E-15,0.));
#4370=DIRECTION('center_axis',(0.,0.,-1.));
#4371=DIRECTION('ref_axis',(1.,-3.33066907387548E-15,0.));
#4372=DIRECTION('center_axis',(0.,0.,-1.));
#4373=DIRECTION('ref_axis',(1.,-3.33066907387548E-15,0.));
#4374=DIRECTION('',(0.,0.,1.));
#4375=DIRECTION('center_axis',(0.,-1.,0.));
#4376=DIRECTION('ref_axis',(1.,0.,0.));
#4377=DIRECTION('',(1.,0.,0.));
#4378=DIRECTION('',(1.,0.,0.));
#4379=DIRECTION('',(0.,0.,1.));
#4380=DIRECTION('center_axis',(0.,0.,1.));
#4381=DIRECTION('ref_axis',(2.22044604925032E-15,1.,0.));
#4382=DIRECTION('center_axis',(0.,0.,-1.));
#4383=DIRECTION('ref_axis',(2.22044604925032E-15,1.,0.));
#4384=DIRECTION('center_axis',(0.,0.,-1.));
#4385=DIRECTION('ref_axis',(2.22044604925032E-15,1.,0.));
#4386=DIRECTION('',(0.,0.,1.));
#4387=DIRECTION('center_axis',(1.,0.,0.));
#4388=DIRECTION('ref_axis',(0.,1.,0.));
#4389=DIRECTION('',(0.,1.,0.));
#4390=DIRECTION('',(0.,1.,0.));
#4391=DIRECTION('',(0.,0.,1.));
#4392=DIRECTION('center_axis',(0.,0.,1.));
#4393=DIRECTION('ref_axis',(-1.,1.66533453693774E-15,0.));
#4394=DIRECTION('center_axis',(0.,0.,-1.));
#4395=DIRECTION('ref_axis',(-1.,1.66533453693774E-15,0.));
#4396=DIRECTION('center_axis',(0.,0.,-1.));
#4397=DIRECTION('ref_axis',(-1.,1.66533453693774E-15,0.));
#4398=DIRECTION('center_axis',(0.,0.,1.));
#4399=DIRECTION('ref_axis',(-1.,0.,0.));
#4400=DIRECTION('center_axis',(0.,0.,1.));
#4401=DIRECTION('ref_axis',(-1.,0.,0.));
#4402=DIRECTION('',(0.,0.,1.));
#4403=DIRECTION('center_axis',(0.,0.,-1.));
#4404=DIRECTION('ref_axis',(-1.,0.,0.));
#4405=DIRECTION('',(0.,0.,1.));
#4406=DIRECTION('center_axis',(0.,1.,0.));
#4407=DIRECTION('ref_axis',(-1.,0.,0.));
#4408=DIRECTION('',(-1.,0.,0.));
#4409=DIRECTION('',(-1.,0.,0.));
#4410=DIRECTION('',(0.,0.,1.));
#4411=DIRECTION('center_axis',(0.,0.,1.));
#4412=DIRECTION('ref_axis',(4.44089209850061E-15,-1.,0.));
#4413=DIRECTION('center_axis',(0.,0.,1.));
#4414=DIRECTION('ref_axis',(4.44089209850061E-15,-1.,0.));
#4415=DIRECTION('center_axis',(0.,0.,-1.));
#4416=DIRECTION('ref_axis',(4.44089209850061E-15,-1.,0.));
#4417=DIRECTION('',(0.,0.,1.));
#4418=DIRECTION('center_axis',(-1.,0.,0.));
#4419=DIRECTION('ref_axis',(0.,-1.,0.));
#4420=DIRECTION('',(0.,-1.,0.));
#4421=DIRECTION('',(0.,-1.,0.));
#4422=DIRECTION('',(0.,0.,1.));
#4423=DIRECTION('center_axis',(0.,1.,0.));
#4424=DIRECTION('ref_axis',(-1.,0.,0.));
#4425=DIRECTION('',(-1.,0.,0.));
#4426=DIRECTION('',(-1.,0.,0.));
#4427=DIRECTION('',(0.,0.,1.));
#4428=DIRECTION('center_axis',(1.,0.,0.));
#4429=DIRECTION('ref_axis',(0.,1.,0.));
#4430=DIRECTION('',(0.,1.,0.));
#4431=DIRECTION('',(0.,1.,0.));
#4432=DIRECTION('',(0.,0.,1.));
#4433=DIRECTION('center_axis',(0.,-1.,0.));
#4434=DIRECTION('ref_axis',(1.,0.,0.));
#4435=DIRECTION('',(1.,0.,0.));
#4436=DIRECTION('',(1.,0.,0.));
#4437=DIRECTION('',(0.,0.,1.));
#4438=DIRECTION('center_axis',(-1.,0.,0.));
#4439=DIRECTION('ref_axis',(0.,-1.,0.));
#4440=DIRECTION('',(0.,-1.,0.));
#4441=DIRECTION('',(0.,-1.,0.));
#4442=DIRECTION('',(0.,0.,1.));
#4443=DIRECTION('center_axis',(0.,0.,1.));
#4444=DIRECTION('ref_axis',(1.,4.4408920985006E-15,0.));
#4445=DIRECTION('center_axis',(0.,0.,1.));
#4446=DIRECTION('ref_axis',(1.,4.4408920985006E-15,0.));
#4447=DIRECTION('center_axis',(0.,0.,-1.));
#4448=DIRECTION('ref_axis',(1.,4.4408920985006E-15,0.));
#4449=DIRECTION('',(0.,0.,1.));
#4450=DIRECTION('center_axis',(0.,-1.,0.));
#4451=DIRECTION('ref_axis',(1.,0.,0.));
#4452=DIRECTION('',(1.,0.,0.));
#4453=DIRECTION('',(1.,0.,0.));
#4454=DIRECTION('',(0.,0.,1.));
#4455=DIRECTION('center_axis',(0.,0.,1.));
#4456=DIRECTION('ref_axis',(0.,1.,0.));
#4457=DIRECTION('center_axis',(0.,0.,1.));
#4458=DIRECTION('ref_axis',(0.,1.,0.));
#4459=DIRECTION('center_axis',(0.,0.,-1.));
#4460=DIRECTION('ref_axis',(0.,1.,0.));
#4461=DIRECTION('',(0.,0.,1.));
#4462=DIRECTION('center_axis',(1.,0.,0.));
#4463=DIRECTION('ref_axis',(0.,1.,0.));
#4464=DIRECTION('',(0.,1.,0.));
#4465=DIRECTION('',(0.,1.,0.));
#4466=DIRECTION('',(0.,0.,1.));
#4467=DIRECTION('center_axis',(0.,-1.,0.));
#4468=DIRECTION('ref_axis',(1.,0.,0.));
#4469=DIRECTION('',(1.,0.,0.));
#4470=DIRECTION('',(1.,0.,0.));
#4471=DIRECTION('',(0.,0.,1.));
#4472=DIRECTION('center_axis',(-1.,0.,0.));
#4473=DIRECTION('ref_axis',(0.,-1.,0.));
#4474=DIRECTION('',(0.,-1.,0.));
#4475=DIRECTION('',(0.,-1.,0.));
#4476=DIRECTION('',(0.,0.,1.));
#4477=DIRECTION('center_axis',(0.,1.,0.));
#4478=DIRECTION('ref_axis',(-1.,0.,0.));
#4479=DIRECTION('',(-1.,0.,0.));
#4480=DIRECTION('',(-1.,0.,0.));
#4481=DIRECTION('',(0.,0.,1.));
#4482=DIRECTION('center_axis',(1.,0.,0.));
#4483=DIRECTION('ref_axis',(0.,1.,0.));
#4484=DIRECTION('',(0.,1.,0.));
#4485=DIRECTION('',(0.,1.,0.));
#4486=DIRECTION('center_axis',(0.,0.,1.));
#4487=DIRECTION('ref_axis',(1.,0.,0.));
#4488=DIRECTION('center_axis',(0.,0.,1.));
#4489=DIRECTION('ref_axis',(1.,0.,0.));
#4894=CARTESIAN_POINT('',(0.,0.,0.));
#4895=CARTESIAN_POINT('Origin',(6.,-6.,0.));
#4896=CARTESIAN_POINT('',(10.0890562790225,-3.88284304114924,0.00188038386388506));
#4897=CARTESIAN_POINT('',(10.3109437209775,-3.88619988433292,0.000572542807928916));
#4898=CARTESIAN_POINT('',(6.,-3.883,2.59257727379495E-16));
#4899=CARTESIAN_POINT('',(11.,-4.63708777074269,-1.61992569438875));
#4900=CARTESIAN_POINT('Ctrl Pts',(10.3109437209775,-3.88619988433292,0.000572542807928916));
#4901=CARTESIAN_POINT('Ctrl Pts',(10.3298470093174,-3.88540275069646,0.316007702174939));
#4902=CARTESIAN_POINT('Ctrl Pts',(10.3487502976573,-3.9515726183054,0.63113445646657));
#4903=CARTESIAN_POINT('Ctrl Pts',(10.3676535859971,-4.08639801625498,0.913504806799793));
#4904=CARTESIAN_POINT('Ctrl Pts',(10.4098100135973,-4.38707359317765,1.54322197643904));
#4905=CARTESIAN_POINT('Ctrl Pts',(10.4519664411975,-5.02920018705039,2.01002863635345));
#4906=CARTESIAN_POINT('Ctrl Pts',(10.4941228687977,-5.72080396656752,2.10193929805125));
#4907=CARTESIAN_POINT('Ctrl Pts',(10.5362792963979,-6.41240774608467,2.19384995974906));
#4908=CARTESIAN_POINT('Ctrl Pts',(10.5784357239981,-7.15348871124624,1.91086462323026));
#4909=CARTESIAN_POINT('Ctrl Pts',(10.6205921515983,-7.60833861494688,1.38152842182621));
#4910=CARTESIAN_POINT('Ctrl Pts',(10.6627485791985,-8.0631885186475,0.852192220422172));
#4911=CARTESIAN_POINT('Ctrl Pts',(10.7049050067987,-8.23180736088723,0.0765051541329273));
#4912=CARTESIAN_POINT('Ctrl Pts',(10.7470614343989,-8.03607510729347,-0.593437148822794));
#4913=CARTESIAN_POINT('Ctrl Pts',(10.789217861999,-7.8403428536997,-1.26337945177852));
#4914=CARTESIAN_POINT('Ctrl Pts',(10.8313742895992,-7.28025950427242,-1.82757699140071));
#4915=CARTESIAN_POINT('Ctrl Pts',(10.8735307171994,-6.61353338525505,-2.02952718354092));
#4916=CARTESIAN_POINT('Ctrl Pts',(10.9156871447996,-5.94680726623768,-2.23147737568112));
#4917=CARTESIAN_POINT('Ctrl Pts',(10.9578435723998,-5.1734383776302,-2.07118022033934));
#4918=CARTESIAN_POINT('Ctrl Pts',(11.,-4.63708777074269,-1.61992569438875));
#4919=CARTESIAN_POINT('',(11.,-4.63477372010686,1.62290954611129));
#4920=CARTESIAN_POINT('Origin',(11.,-6.,0.));
#4921=CARTESIAN_POINT('',(10.8890562790225,-3.88056244769026,-0.00125294615386077));
#4922=CARTESIAN_POINT('Ctrl Pts',(11.,-4.63477280471474,1.62291072646332));
#4923=CARTESIAN_POINT('Ctrl Pts',(10.9630187596742,-4.1668044376417,1.22807503995787));
#4924=CARTESIAN_POINT('Ctrl Pts',(10.9260375193483,-3.88442940297563,0.611672206073652));
#4925=CARTESIAN_POINT('Ctrl Pts',(10.8890562790225,-3.88056244769026,-0.00125294615386077));
#4926=CARTESIAN_POINT('',(12.,-3.883,-2.59257727379495E-16));
#4927=CARTESIAN_POINT('',(6.,-3.883,2.59257727379495E-16));
#4928=CARTESIAN_POINT('Origin',(12.,-6.,0.));
#4929=CARTESIAN_POINT('Ctrl Pts',(10.8890562790225,-3.88056244769026,-0.00125294615386077));
#4930=CARTESIAN_POINT('Ctrl Pts',(10.8848236262981,-3.8801198589972,-0.0714047120918237));
#4931=CARTESIAN_POINT('Ctrl Pts',(10.8805909735737,-3.88332565081622,-0.141510921340689));
#4932=CARTESIAN_POINT('Ctrl Pts',(10.8763583208493,-3.89031913181604,-0.211234160340694));
#4933=CARTESIAN_POINT('Ctrl Pts',(10.8342018932491,-3.95997289144109,-0.905664549114537));
#4934=CARTESIAN_POINT('Ctrl Pts',(10.7920454656489,-4.40535733277697,-1.56210510667178));
#4935=CARTESIAN_POINT('Ctrl Pts',(10.7498890380487,-5.02491685437878,-1.88289988652445));
#4936=CARTESIAN_POINT('Ctrl Pts',(10.7077326104485,-5.6444763759806,-2.20369466637711));
#4937=CARTESIAN_POINT('Ctrl Pts',(10.6655761828483,-6.43821097784834,-2.1888436685252));
#4938=CARTESIAN_POINT('Ctrl Pts',(10.6234197552481,-7.04536578251427,-1.84487773284302));
#4939=CARTESIAN_POINT('Ctrl Pts',(10.5812633276479,-7.65252058718018,-1.50091179716084));
#4940=CARTESIAN_POINT('Ctrl Pts',(10.5391069000478,-8.07309559464429,-0.827830923648425));
#4941=CARTESIAN_POINT('Ctrl Pts',(10.4969504724476,-8.11630674809371,-0.131366079627778));
#4942=CARTESIAN_POINT('Ctrl Pts',(10.4547940448474,-8.15951790154314,0.565098764392898));
#4943=CARTESIAN_POINT('Ctrl Pts',(10.4126376172472,-7.82536520097785,1.2849475789218));
#4944=CARTESIAN_POINT('Ctrl Pts',(10.370481189647,-7.26547901823063,1.70138266663689));
#4945=CARTESIAN_POINT('Ctrl Pts',(10.3283247620468,-6.70559283548343,2.11781775435196));
#4946=CARTESIAN_POINT('Ctrl Pts',(10.2861683344466,-5.91997317055431,2.23083911525323));
#4947=CARTESIAN_POINT('Ctrl Pts',(10.2440119068464,-5.26538953182608,1.98909784789284));
#4948=CARTESIAN_POINT('Ctrl Pts',(10.2018554792462,-4.61080589309784,1.74735658053246));
#4949=CARTESIAN_POINT('Ctrl Pts',(10.159699051646,-4.08725828057048,1.15085268491044));
#4950=CARTESIAN_POINT('Ctrl Pts',(10.1175426240458,-3.93244343062105,0.470451404639381));
#4951=CARTESIAN_POINT('Ctrl Pts',(10.1080471757047,-3.89757243955716,0.317195648024649));
#4952=CARTESIAN_POINT('Ctrl Pts',(10.0985517273636,-3.88140891929161,0.159683399899897));
#4953=CARTESIAN_POINT('Ctrl Pts',(10.0890562790225,-3.88284304114924,0.00188038386388506));
#4954=CARTESIAN_POINT('Origin',(6.,-6.,0.));
#4955=CARTESIAN_POINT('',(9.28905627902251,-3.88625832207874,-0.000568483867972452));
#4956=CARTESIAN_POINT('',(9.5109437209775,-3.88285291798587,-0.00188412158878793));
#4957=CARTESIAN_POINT('',(6.,-3.883,2.59257727379495E-16));
#4958=CARTESIAN_POINT('Ctrl Pts',(9.5109437209775,-3.88285291798587,-0.00188412158878793));
#4959=CARTESIAN_POINT('Ctrl Pts',(9.5435751103829,-3.88777973151044,0.540420553202403));
#4960=CARTESIAN_POINT('Ctrl Pts',(9.5762064997883,-4.10049090304194,1.08616069834087));
#4961=CARTESIAN_POINT('Ctrl Pts',(9.6088378891937,-4.47605139447185,1.4743533520236));
#4962=CARTESIAN_POINT('Ctrl Pts',(9.65099431679389,-4.9612372524739,1.97585867552033));
#4963=CARTESIAN_POINT('Ctrl Pts',(9.69315074439408,-5.71821870890957,2.21441715497353));
#4964=CARTESIAN_POINT('Ctrl Pts',(9.73530717199427,-6.40327135435487,2.08170804052273));
#4965=CARTESIAN_POINT('Ctrl Pts',(9.77746359959446,-7.08832399980019,1.94899892607192));
#4966=CARTESIAN_POINT('Ctrl Pts',(9.81962002719465,-7.70144783425515,1.44502221771709));
#4967=CARTESIAN_POINT('Ctrl Pts',(9.86177645479484,-7.96426282646742,0.798615346598204));
#4968=CARTESIAN_POINT('Ctrl Pts',(9.90393288239503,-8.22707781867969,0.152208475479324));
#4969=CARTESIAN_POINT('Ctrl Pts',(9.94608930999523,-8.1395839686493,-0.636628558403595));
#4970=CARTESIAN_POINT('Ctrl Pts',(9.98824573759542,-7.74147846610521,-1.20971721337014));
#4971=CARTESIAN_POINT('Ctrl Pts',(10.0304021651956,-7.34337296356112,-1.78280586833669));
#4972=CARTESIAN_POINT('Ctrl Pts',(10.0725585927958,-6.63465580850333,-2.14014614438684));
#4973=CARTESIAN_POINT('Ctrl Pts',(10.114715020396,-5.9371863419647,-2.11947983260037));
#4974=CARTESIAN_POINT('Ctrl Pts',(10.1568714479962,-5.23971687542607,-2.0988135208139));
#4975=CARTESIAN_POINT('Ctrl Pts',(10.1990278755964,-4.5534950974066,-1.70014062119081));
#4976=CARTESIAN_POINT('Ctrl Pts',(10.2411843031966,-4.18999648838316,-1.1044903316972));
#4977=CARTESIAN_POINT('Ctrl Pts',(10.2644374424569,-3.98949364082893,-0.775934523709865));
#4978=CARTESIAN_POINT('Ctrl Pts',(10.2876905817172,-3.88718044703313,-0.387447655396757));
#4979=CARTESIAN_POINT('Ctrl Pts',(10.3109437209775,-3.88619988433292,0.000572542807928916));
#4980=CARTESIAN_POINT('Ctrl Pts',(10.0890562790225,-3.88284304114924,0.00188038386388506));
#4981=CARTESIAN_POINT('Ctrl Pts',(10.0563952997634,-3.88777591241182,-0.540906101683727));
#4982=CARTESIAN_POINT('Ctrl Pts',(10.0237343205043,-4.10090936331863,-1.08713270990473));
#4983=CARTESIAN_POINT('Ctrl Pts',(9.99107334124527,-4.4770789027728,-1.47541427191919));
#4984=CARTESIAN_POINT('Ctrl Pts',(9.94891691364508,-4.96261131224547,-1.97658000328661));
#4985=CARTESIAN_POINT('Ctrl Pts',(9.90676048604489,-5.71975821856232,-2.21461280110137));
#4986=CARTESIAN_POINT('Ctrl Pts',(9.8646040584447,-6.40472126940695,-2.08142682840507));
#4987=CARTESIAN_POINT('Ctrl Pts',(9.82244763084451,-7.0896843202516,-1.94824085570876));
#4988=CARTESIAN_POINT('Ctrl Pts',(9.78029120324431,-7.70246351562404,-1.44383611250138));
#4989=CARTESIAN_POINT('Ctrl Pts',(9.73813477564412,-7.9648231489573,-0.797245612832521));
#4990=CARTESIAN_POINT('Ctrl Pts',(9.69597834804393,-8.22718278229054,-0.150655113163675));
#4991=CARTESIAN_POINT('Ctrl Pts',(9.65382192044375,-8.13912285358463,0.638121142966619));
#4992=CARTESIAN_POINT('Ctrl Pts',(9.61166549284356,-7.74062604192175,1.21093142563168));
#4993=CARTESIAN_POINT('Ctrl Pts',(9.56950906524337,-7.34212923025887,1.78374170829674));
#4994=CARTESIAN_POINT('Ctrl Pts',(9.52735263764317,-6.63319553563902,2.14058601749655));
#4995=CARTESIAN_POINT('Ctrl Pts',(9.48519621004298,-5.93572544911276,2.11943448582987));
#4996=CARTESIAN_POINT('Ctrl Pts',(9.44303978244279,-5.23825536258647,2.09828295416318));
#4997=CARTESIAN_POINT('Ctrl Pts',(9.4008833548426,-4.55224888415376,1.69913558162997));
#4998=CARTESIAN_POINT('Ctrl Pts',(9.35872692724241,-4.18919459490055,1.1032301330012));
#4999=CARTESIAN_POINT('Ctrl Pts',(9.33550337783578,-3.98919166050286,0.774951850999683));
#5000=CARTESIAN_POINT('Ctrl Pts',(9.31227982842914,-3.88719814718334,0.386961494651881));
#5001=CARTESIAN_POINT('Ctrl Pts',(9.28905627902251,-3.88625832207874,-0.000568483867972452));
#5002=CARTESIAN_POINT('Origin',(6.,-6.,0.));
#5003=CARTESIAN_POINT('',(8.4890562790225,-3.88081569696024,-0.00138638344793468));
#5004=CARTESIAN_POINT('',(8.7109437209775,-3.88042895428249,0.00117038079968268));
#5005=CARTESIAN_POINT('',(6.,-3.883,2.59257727379495E-16));
#5006=CARTESIAN_POINT('Ctrl Pts',(8.7109437209775,-3.88042895428249,0.00117038079968268));
#5007=CARTESIAN_POINT('Ctrl Pts',(8.71514678384823,-3.87996428152845,0.0708143797887767));
#5008=CARTESIAN_POINT('Ctrl Pts',(8.71934984671896,-3.88310204798081,0.140416007857776));
#5009=CARTESIAN_POINT('Ctrl Pts',(8.72355290958969,-3.88998055273578,0.209645965979184));
#5010=CARTESIAN_POINT('Ctrl Pts',(8.76570933718988,-3.95897147593134,0.904017619954446));
#5011=CARTESIAN_POINT('Ctrl Pts',(8.80786576479007,-4.40427880810987,1.56099946242998));
#5012=CARTESIAN_POINT('Ctrl Pts',(8.85002219239026,-5.02370573481769,1.88228135692562));
#5013=CARTESIAN_POINT('Ctrl Pts',(8.89217861999045,-5.64313266152551,2.20356325142126));
#5014=CARTESIAN_POINT('Ctrl Pts',(8.93433504759064,-6.43667918276262,2.189145197937));
#5015=CARTESIAN_POINT('Ctrl Pts',(8.97649147519083,-7.04402622875504,1.84557386816763));
#5016=CARTESIAN_POINT('Ctrl Pts',(9.01864790279102,-7.65137327474745,1.50200253839825));
#5017=CARTESIAN_POINT('Ctrl Pts',(9.06080433039121,-8.07252084549518,0.829277932343754));
#5018=CARTESIAN_POINT('Ctrl Pts',(9.1029607579914,-8.11624237804386,0.132858395408587));
#5019=CARTESIAN_POINT('Ctrl Pts',(9.14511718559159,-8.15996391059253,-0.563561141526579));
#5020=CARTESIAN_POINT('Ctrl Pts',(9.18727361319179,-7.82625940494216,-1.28367560934241));
#5021=CARTESIAN_POINT('Ctrl Pts',(9.22943004079198,-7.26665060216368,-1.70050881300008));
#5022=CARTESIAN_POINT('Ctrl Pts',(9.27158646839217,-6.7070417993852,-2.11734201665774));
#5023=CARTESIAN_POINT('Ctrl Pts',(9.31374289599236,-5.9215286994786,-2.23089395615724));
#5024=CARTESIAN_POINT('Ctrl Pts',(9.35589932359255,-5.26678371915212,-1.9896049943898));
#5025=CARTESIAN_POINT('Ctrl Pts',(9.39805575119274,-4.61203873882566,-1.74831603262238));
#5026=CARTESIAN_POINT('Ctrl Pts',(9.44021217879293,-4.0880618780793,-1.15218616958803));
#5027=CARTESIAN_POINT('Ctrl Pts',(9.48236860639312,-3.93276857749032,-0.471895154300735));
#5028=CARTESIAN_POINT('Ctrl Pts',(9.49189364458792,-3.89768081736193,-0.318186733709686));
#5029=CARTESIAN_POINT('Ctrl Pts',(9.50141868278271,-3.88141479083728,-0.16018178634426));
#5030=CARTESIAN_POINT('Ctrl Pts',(9.5109437209775,-3.88285291798587,-0.00188412158878793));
#5031=CARTESIAN_POINT('Ctrl Pts',(9.28905627902251,-3.88625832207874,-0.000568483867972452));
#5032=CARTESIAN_POINT('Ctrl Pts',(9.27012340082895,-3.88549213453708,-0.316500288744127));
#5033=CARTESIAN_POINT('Ctrl Pts',(9.25119052263539,-3.95188866409716,-0.632126115418351));
#5034=CARTESIAN_POINT('Ctrl Pts',(9.23225764444183,-4.08709739014463,-0.91484264263593));
#5035=CARTESIAN_POINT('Ctrl Pts',(9.19010121684164,-4.38815657471562,-1.54434644491999));
#5036=CARTESIAN_POINT('Ctrl Pts',(9.14794478924145,-5.03037704393129,-2.01069052476379));
#5037=CARTESIAN_POINT('Ctrl Pts',(9.10578836164126,-5.72215108182613,-2.10212591529422));
#5038=CARTESIAN_POINT('Ctrl Pts',(9.06363193404107,-6.41392511972096,-2.19356130582466));
#5039=CARTESIAN_POINT('Ctrl Pts',(9.02147550644088,-7.15525272629495,-1.91008800704174));
#5040=CARTESIAN_POINT('Ctrl Pts',(8.97931907884069,-7.6095256731943,-1.38042036796998));
#5041=CARTESIAN_POINT('Ctrl Pts',(8.9371626512405,-8.06379862009367,-0.850752728898211));
#5042=CARTESIAN_POINT('Ctrl Pts',(8.89500622364031,-8.23101690731839,-0.0748907495375924));
#5043=CARTESIAN_POINT('Ctrl Pts',(8.85284979604012,-8.03525311381774,0.594876562001453));
#5044=CARTESIAN_POINT('Ctrl Pts',(8.81069336843993,-7.8394893203171,1.26464387354049));
#5045=CARTESIAN_POINT('Ctrl Pts',(8.76853694083974,-7.28074344609107,1.82831651725797));
#5046=CARTESIAN_POINT('Ctrl Pts',(8.72638051323955,-6.6127204856351,2.02995245057092));
#5047=CARTESIAN_POINT('Ctrl Pts',(8.68422408563935,-5.94469752517913,2.23158838388388));
#5048=CARTESIAN_POINT('Ctrl Pts',(8.64206765803916,-5.1673974784932,2.07118760679231));
#5049=CARTESIAN_POINT('Ctrl Pts',(8.59991123043897,-4.63376233782377,1.62158193871465));
#5050=CARTESIAN_POINT('Ctrl Pts',(8.56295957996681,-4.16601162173637,1.22748612835167));
#5051=CARTESIAN_POINT('Ctrl Pts',(8.52600792949465,-3.88547263914832,0.611189469031259));
#5052=CARTESIAN_POINT('Ctrl Pts',(8.4890562790225,-3.88081569696024,-0.00138638344793468));
#5053=CARTESIAN_POINT('Origin',(6.,-6.,0.));
#5054=CARTESIAN_POINT('',(7.68905627902251,-3.88235469492868,0.00183633483374523));
#5055=CARTESIAN_POINT('',(7.9109437209775,-3.88609278259416,0.000819409314603885));
#5056=CARTESIAN_POINT('',(6.,-3.883,2.59257727379495E-16));
#5057=CARTESIAN_POINT('Ctrl Pts',(7.9109437209775,-3.88609278259416,0.000819409314603885));
#5058=CARTESIAN_POINT('Ctrl Pts',(7.92887488491375,-3.88504204554916,0.299977116189444));
#5059=CARTESIAN_POINT('Ctrl Pts',(7.94680604885,-3.94433953053336,0.598737191648719));
#5060=CARTESIAN_POINT('Ctrl Pts',(7.96473721278625,-4.06603975290357,0.869443107203424));
#5061=CARTESIAN_POINT('Ctrl Pts',(8.00689364038644,-4.35215874838639,1.505876657786));
#5062=CARTESIAN_POINT('Ctrl Pts',(8.04905006798663,-4.98319449029903,1.98724730626784));
#5063=CARTESIAN_POINT('Ctrl Pts',(8.09120649558682,-5.67261796286648,2.09498318776012));
#5064=CARTESIAN_POINT('Ctrl Pts',(8.13336292318701,-6.36204143543391,2.2027190692524));
#5065=CARTESIAN_POINT('Ctrl Pts',(8.1755193507872,-7.10985263865614,1.93682018375513));
#5066=CARTESIAN_POINT('Ctrl Pts',(8.21767577838739,-7.57649931373914,1.41802097027599));
#5067=CARTESIAN_POINT('Ctrl Pts',(8.25983220598758,-8.04314598882215,0.899221756796831));
#5068=CARTESIAN_POINT('Ctrl Pts',(8.30198863358777,-8.22862813576591,0.127522215335779));
#5069=CARTESIAN_POINT('Ctrl Pts',(8.34414506118797,-8.04872546454541,-0.546678624303283));
#5070=CARTESIAN_POINT('Ctrl Pts',(8.38630148878816,-7.86882279332492,-1.22087946394234));
#5071=CARTESIAN_POINT('Ctrl Pts',(8.42845791638835,-7.32353530394018,-1.7975816017594));
#5072=CARTESIAN_POINT('Ctrl Pts',(8.47061434398854,-6.66045702367441,-2.01492681722953));
#5073=CARTESIAN_POINT('Ctrl Pts',(8.51277077158873,-5.99737874340865,-2.23227203269965));
#5074=CARTESIAN_POINT('Ctrl Pts',(8.55492719918892,-5.21650967226187,-2.09026032582285));
#5075=CARTESIAN_POINT('Ctrl Pts',(8.59708362678911,-4.67241239379476,-1.65337373964697));
#5076=CARTESIAN_POINT('Ctrl Pts',(8.63503699151858,-4.18256247923803,-1.2600454408689));
#5077=CARTESIAN_POINT('Ctrl Pts',(8.67299035624804,-3.88462491685935,-0.627710075226815));
#5078=CARTESIAN_POINT('Ctrl Pts',(8.7109437209775,-3.88042895428249,0.00117038079968268));
#5079=CARTESIAN_POINT('Ctrl Pts',(8.4890562790225,-3.88081569696024,-0.00138638344793468));
#5080=CARTESIAN_POINT('Ctrl Pts',(8.48385150189447,-3.88015974936717,-0.0876699660601046));
#5081=CARTESIAN_POINT('Ctrl Pts',(8.47864672476643,-3.88497723749026,-0.173879728727243));
#5082=CARTESIAN_POINT('Ctrl Pts',(8.4734419476384,-3.89551595094417,-0.259384332255975));
#5083=CARTESIAN_POINT('Ctrl Pts',(8.4312855200382,-3.98087493938691,-0.951934376085218));
#5084=CARTESIAN_POINT('Ctrl Pts',(8.38912909243802,-4.44156315092533,-1.59822390467993));
#5085=CARTESIAN_POINT('Ctrl Pts',(8.34697266483782,-5.06839981536676,-1.90479774186325));
#5086=CARTESIAN_POINT('Ctrl Pts',(8.30481623723763,-5.69523647980819,-2.21137157904657));
#5087=CARTESIAN_POINT('Ctrl Pts',(8.26265980963744,-6.48822159715263,-2.17822972481849));
#5088=CARTESIAN_POINT('Ctrl Pts',(8.22050338203725,-7.08729117964857,-1.82042061921142));
#5089=CARTESIAN_POINT('Ctrl Pts',(8.17834695443706,-7.68636076214451,-1.46261151360435));
#5090=CARTESIAN_POINT('Ctrl Pts',(8.13619052683687,-8.09151480979196,-0.780135156618282));
#5091=CARTESIAN_POINT('Ctrl Pts',(8.09403409923668,-8.11878847871396,-0.0828777667085811));
#5092=CARTESIAN_POINT('Ctrl Pts',(8.05187767163649,-8.14606214763596,0.61437962320112));
#5093=CARTESIAN_POINT('Ctrl Pts',(8.00972124403629,-7.79545543783251,1.32641804603445));
#5094=CARTESIAN_POINT('Ctrl Pts',(7.9675648164361,-7.22616534830724,1.72992828747435));
#5095=CARTESIAN_POINT('Ctrl Pts',(7.92540838883591,-6.65687525878197,2.13343852891425));
#5096=CARTESIAN_POINT('Ctrl Pts',(7.88325196123572,-5.86890178953488,2.22842058896072));
#5097=CARTESIAN_POINT('Ctrl Pts',(7.84109553363553,-5.2200333333253,1.97174677379236));
#5098=CARTESIAN_POINT('Ctrl Pts',(7.79893910603534,-4.57116487711572,1.71507295862401));
#5099=CARTESIAN_POINT('Ctrl Pts',(7.75678267843515,-4.06140143394366,1.10674326824082));
#5100=CARTESIAN_POINT('Ctrl Pts',(7.71462625083496,-3.92220694306612,0.422976776968435));
#5101=CARTESIAN_POINT('Ctrl Pts',(7.70610292689748,-3.89406414720794,0.284730639084455));
#5102=CARTESIAN_POINT('Ctrl Pts',(7.69757960295999,-3.88106949506508,0.143400790343917));
#5103=CARTESIAN_POINT('Ctrl Pts',(7.68905627902251,-3.88235469492868,0.00183633483374523));
#5104=CARTESIAN_POINT('Origin',(6.,-6.,0.));
#5105=CARTESIAN_POINT('',(6.8890562790225,-3.88636003231944,-0.00031417126607286));
#5106=CARTESIAN_POINT('',(7.1109437209775,-3.88333340233497,-0.00189050360831077));
#5107=CARTESIAN_POINT('',(6.,-3.883,2.59257727379495E-16));
#5108=CARTESIAN_POINT('Ctrl Pts',(7.1109437209775,-3.88333340233497,-0.00189050360831077));
#5109=CARTESIAN_POINT('Ctrl Pts',(7.14260298597927,-3.88803082624995,0.524564043326856));
#5110=CARTESIAN_POINT('Ctrl Pts',(7.17426225098104,-4.087035328391,1.05418914371193));
#5111=CARTESIAN_POINT('Ctrl Pts',(7.20592151598281,-4.4426850828802,1.43906351629628));
#5112=CARTESIAN_POINT('Ctrl Pts',(7.248077943583,-4.91625650424173,1.95154947015887));
#5113=CARTESIAN_POINT('Ctrl Pts',(7.29023437118319,-5.66757096416104,2.20738221321448));
#5114=CARTESIAN_POINT('Ctrl Pts',(7.33239079878338,-6.35548551341645,2.09039795368626));
#5115=CARTESIAN_POINT('Ctrl Pts',(7.37454722638357,-7.04340006267187,1.97341369415804));
#5116=CARTESIAN_POINT('Ctrl Pts',(7.41670365398376,-7.66791470126341,1.483612432046));
#5117=CARTESIAN_POINT('Ctrl Pts',(7.45886008158396,-7.9454613933261,0.843394049180934));
#5118=CARTESIAN_POINT('Ctrl Pts',(7.50101650918415,-8.22300808538879,0.203175666315868));
#5119=CARTESIAN_POINT('Ctrl Pts',(7.54317293678433,-8.15358683092263,-0.587459837302209));
#5120=CARTESIAN_POINT('Ctrl Pts',(7.58532936438453,-7.76871914701981,-1.16951534144242));
#5121=CARTESIAN_POINT('Ctrl Pts',(7.62748579198471,-7.38385146311698,-1.75157084558263));
#5122=CARTESIAN_POINT('Ctrl Pts',(7.66964221958491,-6.6835373497775,-2.12504635024497));
#5123=CARTESIAN_POINT('Ctrl Pts',(7.7117986471851,-5.98576246358723,-2.12036101821588));
#5124=CARTESIAN_POINT('Ctrl Pts',(7.75395507478529,-5.28798757739695,-2.1156756861868));
#5125=CARTESIAN_POINT('Ctrl Pts',(7.79611150238548,-4.59275191835588,-1.7328295174663));
#5126=CARTESIAN_POINT('Ctrl Pts',(7.83826792998567,-4.21573521336184,-1.14565820676439));
#5127=CARTESIAN_POINT('Ctrl Pts',(7.86249319364961,-3.9990819150603,-0.80823920265523));
#5128=CARTESIAN_POINT('Ctrl Pts',(7.88671845731356,-3.88751234364703,-0.403347010216734));
#5129=CARTESIAN_POINT('Ctrl Pts',(7.9109437209775,-3.88609278259416,0.000819409314603885));
#5130=CARTESIAN_POINT('Ctrl Pts',(7.68905627902251,-3.88235469492868,0.00183633483374523));
#5131=CARTESIAN_POINT('Ctrl Pts',(7.6554231753598,-3.88742610375424,-0.556778126150017));
#5132=CARTESIAN_POINT('Ctrl Pts',(7.62179007169709,-4.11484877990915,-1.11904564407922));
#5133=CARTESIAN_POINT('Ctrl Pts',(7.58815696803438,-4.51127209883019,-1.50990813544534));
#5134=CARTESIAN_POINT('Ctrl Pts',(7.54600054043419,-5.00815728405479,-1.99982326442516));
#5135=CARTESIAN_POINT('Ctrl Pts',(7.503844112834,-5.770553193087,-2.22045023022322));
#5136=CARTESIAN_POINT('Ctrl Pts',(7.46168768523381,-6.45228521760907,-2.07161082810745));
#5137=CARTESIAN_POINT('Ctrl Pts',(7.41953125763362,-7.13401724213114,-1.92277142599167));
#5138=CARTESIAN_POINT('Ctrl Pts',(7.37737483003343,-7.73508538214306,-1.40446565596207));
#5139=CARTESIAN_POINT('Ctrl Pts',(7.33521840243324,-7.98256775348064,-0.752036198654528));
#5140=CARTESIAN_POINT('Ctrl Pts',(7.29306197483304,-8.23005012481823,-0.0996067413469874));
#5141=CARTESIAN_POINT('Ctrl Pts',(7.25090554723286,-8.12394672748148,0.686946403238489));
#5142=CARTESIAN_POINT('Ctrl Pts',(7.20874911963266,-7.71243502620873,1.25047975682414));
#5143=CARTESIAN_POINT('Ctrl Pts',(7.16659269203247,-7.30092332493598,1.81401311040979));
#5144=CARTESIAN_POINT('Ctrl Pts',(7.12443626443228,-6.58400331972723,2.15452667299561));
#5145=CARTESIAN_POINT('Ctrl Pts',(7.08227983683209,-5.88720076311748,2.11740635527826));
#5146=CARTESIAN_POINT('Ctrl Pts',(7.0401234092319,-5.19039820650772,2.08028603756091));
#5147=CARTESIAN_POINT('Ctrl Pts',(6.99796698163171,-4.51371309849697,1.66553183954039));
#5148=CARTESIAN_POINT('Ctrl Pts',(6.95581055403152,-4.16440207499811,1.06146766269465));
#5149=CARTESIAN_POINT('Ctrl Pts',(6.93355912902851,-3.98002525550516,0.742624499427559));
#5150=CARTESIAN_POINT('Ctrl Pts',(6.91130770402551,-3.88685631420567,0.37103873280126));
#5151=CARTESIAN_POINT('Ctrl Pts',(6.8890562790225,-3.88636003231944,-0.00031417126607286));
#5152=CARTESIAN_POINT('Origin',(6.,-6.,0.));
#5153=CARTESIAN_POINT('',(6.0890562790225,-3.88123446329707,-0.00156260716336218));
#5154=CARTESIAN_POINT('',(6.3109437209775,-3.88010896117177,0.000931372864572485));
#5155=CARTESIAN_POINT('',(6.,-3.883,2.59257727379495E-16));
#5156=CARTESIAN_POINT('Ctrl Pts',(6.3109437209775,-3.88010896117177,0.000931372864572485));
#5157=CARTESIAN_POINT('Ctrl Pts',(6.3141746594446,-3.87981270635624,0.0544460888779948));
#5158=CARTESIAN_POINT('Ctrl Pts',(6.3174055979117,-3.88166513255228,0.107939967166579));
#5159=CARTESIAN_POINT('Ctrl Pts',(6.3206365363788,-3.88573247061989,0.161264903944568));
#5160=CARTESIAN_POINT('Ctrl Pts',(6.36279296397899,-3.93880201821999,0.857034526132367));
#5161=CARTESIAN_POINT('Ctrl Pts',(6.40494939157918,-4.36894564474271,1.52404297487717));
#5162=CARTESIAN_POINT('Ctrl Pts',(6.44710581917937,-4.98085170215647,1.85942741241423));
#5163=CARTESIAN_POINT('Ctrl Pts',(6.48926224677956,-5.59275775957023,2.19481184995129));
#5164=CARTESIAN_POINT('Ctrl Pts',(6.53141867437975,-6.38642624787501,2.19857227628061));
#5165=CARTESIAN_POINT('Ctrl Pts',(6.57357510197994,-7.00148288535931,1.86900122668953));
#5166=CARTESIAN_POINT('Ctrl Pts',(6.61573152958014,-7.6165395228436,1.53943017709846));
#5167=CARTESIAN_POINT('Ctrl Pts',(6.65788795718033,-8.05298430950739,0.876527651586999));
#5168=CARTESIAN_POINT('Ctrl Pts',(6.70004438478052,-8.11264448327204,0.181292146374433));
#5169=CARTESIAN_POINT('Ctrl Pts',(6.74220081238071,-8.17230465703668,-0.513943358838142));
#5170=CARTESIAN_POINT('Ctrl Pts',(6.7843572399809,-7.85518021790216,-1.24151184375183));
#5171=CARTESIAN_POINT('Ctrl Pts',(6.82651366758109,-7.30526515536498,-1.67105249146255));
#5172=CARTESIAN_POINT('Ctrl Pts',(6.86867009518128,-6.7553500928278,-2.10059313917327));
#5173=CARTESIAN_POINT('Ctrl Pts',(6.91082652278147,-5.97264440688797,-2.23210594968102));
#5174=CARTESIAN_POINT('Ctrl Pts',(6.95298295038166,-5.31254459307855,-2.00587602272101));
#5175=CARTESIAN_POINT('Ctrl Pts',(6.99513937798185,-4.65244477926912,-1.779646095761));
#5176=CARTESIAN_POINT('Ctrl Pts',(7.03729580558204,-4.11495083759011,-1.19567343133322));
#5177=CARTESIAN_POINT('Ctrl Pts',(7.07945223318223,-3.94411805815251,-0.519117516784533));
#5178=CARTESIAN_POINT('Ctrl Pts',(7.08994939578066,-3.90157983646295,-0.350651689715541));
#5179=CARTESIAN_POINT('Ctrl Pts',(7.10044655837907,-3.88177589230982,-0.176445376551414));
#5180=CARTESIAN_POINT('Ctrl Pts',(7.1109437209775,-3.88333340233497,-0.00189050360831077));
#5181=CARTESIAN_POINT('Ctrl Pts',(6.8890562790225,-3.88636003231944,-0.00031417126607286));
#5182=CARTESIAN_POINT('Ctrl Pts',(6.86915127642532,-3.8859160835731,-0.33250775073049));
#5183=CARTESIAN_POINT('Ctrl Pts',(6.84924627382813,-3.95963055094797,-0.664514989167724));
#5184=CARTESIAN_POINT('Ctrl Pts',(6.82934127123095,-4.10855197683347,-0.958414167713982));
#5185=CARTESIAN_POINT('Ctrl Pts',(6.78718484363076,-4.42394984115464,-1.58085766560597));
#5186=CARTESIAN_POINT('Ctrl Pts',(6.74502841603057,-5.07668250878394,-2.03237050571901));
#5187=CARTESIAN_POINT('Ctrl Pts',(6.70287198843038,-5.77036922413792,-2.10793810345388));
#5188=CARTESIAN_POINT('Ctrl Pts',(6.66071556083019,-6.46405593949191,-2.18350570118874));
#5189=CARTESIAN_POINT('Ctrl Pts',(6.61855913322999,-7.19869670257056,-1.88312805654543));
#5190=CARTESIAN_POINT('Ctrl Pts',(6.5764027056298,-7.64071944743897,-1.34319508486732));
#5191=CARTESIAN_POINT('Ctrl Pts',(6.53424627802961,-8.08274219230738,-0.803262113189214));
#5192=CARTESIAN_POINT('Ctrl Pts',(6.49208985042942,-8.23214691896553,-0.0237738144762983));
#5193=CARTESIAN_POINT('Ctrl Pts',(6.44993342282923,-8.0210946973726,0.641334207311783));
#5194=CARTESIAN_POINT('Ctrl Pts',(6.40777699522904,-7.81004247577966,1.30644222909986));
#5195=CARTESIAN_POINT('Ctrl Pts',(6.36562056762885,-7.23853330593564,1.85716997396313));
#5196=CARTESIAN_POINT('Ctrl Pts',(6.32346414002865,-6.56606748249676,2.04345319165272));
#5197=CARTESIAN_POINT('Ctrl Pts',(6.28130771242846,-5.89360165905787,2.22973640934232));
#5198=CARTESIAN_POINT('Ctrl Pts',(6.23915128482827,-5.12017918202413,2.05157509985824));
#5199=CARTESIAN_POINT('Ctrl Pts',(6.19699485722808,-4.59698139943735,1.58986544955578));
#5200=CARTESIAN_POINT('Ctrl Pts',(6.16101533115955,-4.15044431531567,1.19580704980958));
#5201=CARTESIAN_POINT('Ctrl Pts',(6.12503580509103,-3.8861764962572,0.595205695519721));
#5202=CARTESIAN_POINT('Ctrl Pts',(6.0890562790225,-3.88123446329707,-0.00156260716336218));
#5203=CARTESIAN_POINT('Origin',(6.,-6.,0.));
#5204=CARTESIAN_POINT('',(5.2890562790225,-3.88187782281943,0.00175000188907953));
#5205=CARTESIAN_POINT('',(5.51094372097749,-3.88587578853395,0.0010475127251217));
#5206=CARTESIAN_POINT('',(6.,-3.883,2.59257727379495E-16));
#5207=CARTESIAN_POINT('Ctrl Pts',(5.51094372097749,-3.88587578853395,0.0010475127251217));
#5208=CARTESIAN_POINT('Ctrl Pts',(5.52790276051011,-3.88459758142574,0.283913878504502));
#5209=CARTESIAN_POINT('Ctrl Pts',(5.54486180004273,-3.93742581719468,0.566322436662692));
#5210=CARTESIAN_POINT('Ctrl Pts',(5.56182083957536,-4.0466340760357,0.824921282384071));
#5211=CARTESIAN_POINT('Ctrl Pts',(5.60397726717555,-4.31810169354546,1.46774091236234));
#5212=CARTESIAN_POINT('Ctrl Pts',(5.64613369477574,-4.93794700987619,1.96343799118942));
#5213=CARTESIAN_POINT('Ctrl Pts',(5.68829012237593,-5.62472214856941,2.08693557381648));
#5214=CARTESIAN_POINT('Ctrl Pts',(5.73044654997612,-6.31149728726264,2.21043315644353));
#5215=CARTESIAN_POINT('Ctrl Pts',(5.77260297757631,-7.06520224831835,1.96173124287054));
#5216=CARTESIAN_POINT('Ctrl Pts',(5.8147594051765,-7.54360864801481,1.45375578994855));
#5217=CARTESIAN_POINT('Ctrl Pts',(5.85691583277669,-8.02201504771127,0.94578033702656));
#5218=CARTESIAN_POINT('Ctrl Pts',(5.89907226037688,-8.22512288604848,0.178531344755563));
#5219=CARTESIAN_POINT('Ctrl Pts',(5.94122868797708,-8.06070871907031,-0.499612980398527));
#5220=CARTESIAN_POINT('Ctrl Pts',(5.98338511557727,-7.89629455209214,-1.17775730555262));
#5221=CARTESIAN_POINT('Ctrl Pts',(6.02554154317746,-7.36435837979858,-1.76679696358982));
#5222=CARTESIAN_POINT('Ctrl Pts',(6.06769797077765,-6.70643192334511,-1.99927174058805));
#5223=CARTESIAN_POINT('Ctrl Pts',(6.10985439837784,-6.04850546689163,-2.23174651758629));
#5224=CARTESIAN_POINT('Ctrl Pts',(6.15201082597803,-5.26458872627824,-2.10765641354556));
#5225=CARTESIAN_POINT('Ctrl Pts',(6.19416725357822,-4.71062809031028,-1.68334596370979));
#5226=CARTESIAN_POINT('Ctrl Pts',(6.23309274271131,-4.19912391543011,-1.29155536985824));
#5227=CARTESIAN_POINT('Ctrl Pts',(6.2720182318444,-3.88367816056074,-0.643799722404717));
#5228=CARTESIAN_POINT('Ctrl Pts',(6.3109437209775,-3.88010896117177,0.000931372864572485));
#5229=CARTESIAN_POINT('Ctrl Pts',(6.0890562790225,-3.88123446329707,-0.00156260716336218));
#5230=CARTESIAN_POINT('Ctrl Pts',(6.08287937749084,-3.88038602380115,-0.104014736073326));
#5231=CARTESIAN_POINT('Ctrl Pts',(6.07670247595917,-3.8871808011753,-0.206353891857302));
#5232=CARTESIAN_POINT('Ctrl Pts',(6.07052557442751,-3.90200869710868,-0.307515583683664));
#5233=CARTESIAN_POINT('Ctrl Pts',(6.02836914682732,-4.00320686550659,-0.997928975499783));
#5234=CARTESIAN_POINT('Ctrl Pts',(5.98621271922713,-4.47857629044222,-1.63349776801118));
#5235=CARTESIAN_POINT('Ctrl Pts',(5.94405629162693,-5.11227003130558,-1.92563466002711));
#5236=CARTESIAN_POINT('Ctrl Pts',(5.90189986402674,-5.74596377216895,-2.21777155204305));
#5237=CARTESIAN_POINT('Ctrl Pts',(5.85974343642655,-6.53798182896006,-2.16647654356351));
#5238=CARTESIAN_POINT('Ctrl Pts',(5.81758700882636,-7.12869931732839,-1.7950407216212));
#5239=CARTESIAN_POINT('Ctrl Pts',(5.77543058122617,-7.71941680569672,-1.4236048996789));
#5240=CARTESIAN_POINT('Ctrl Pts',(5.73327415362598,-8.10883372564228,-0.732028264273839));
#5241=CARTESIAN_POINT('Ctrl Pts',(5.69111772602579,-8.12013085745316,-0.0343291201587056));
#5242=CARTESIAN_POINT('Ctrl Pts',(5.6489612984256,-8.13142798926403,0.663370023956428));
#5243=CARTESIAN_POINT('Ctrl Pts',(5.60680487082541,-7.76460533294022,1.36719167678164));
#5244=CARTESIAN_POINT('Ctrl Pts',(5.56464844322521,-7.18622292360526,1.75755754293546));
#5245=CARTESIAN_POINT('Ctrl Pts',(5.52249201562502,-6.60784051427029,2.14792340908928));
#5246=CARTESIAN_POINT('Ctrl Pts',(5.48033558802483,-5.81789835192417,2.22483348857171));
#5247=CARTESIAN_POINT('Ctrl Pts',(5.43817916042464,-5.17507873723095,1.95336587751692));
#5248=CARTESIAN_POINT('Ctrl Pts',(5.39602273282445,-4.53225912253772,1.68189826646213));
#5249=CARTESIAN_POINT('Ctrl Pts',(5.35386630522426,-4.03656205549739,1.06205296487013));
#5250=CARTESIAN_POINT('Ctrl Pts',(5.31170987762407,-3.91306447580689,0.375277842507117));
#5251=CARTESIAN_POINT('Ctrl Pts',(5.30415867809022,-3.89094317855098,0.252260398215228));
#5252=CARTESIAN_POINT('Ctrl Pts',(5.29660747855636,-3.88076396363212,0.127095499513492));
#5253=CARTESIAN_POINT('Ctrl Pts',(5.2890562790225,-3.88187782281943,0.00175000188907953));
#5254=CARTESIAN_POINT('Origin',(6.,-6.,0.));
#5255=CARTESIAN_POINT('',(4.4890562790225,-3.88640241446317,-5.40837461397714E-5));
#5256=CARTESIAN_POINT('',(4.71094372097749,-3.88380208938619,-0.00185818885717421));
#5257=CARTESIAN_POINT('',(6.,-3.883,2.59257727379495E-16));
#5258=CARTESIAN_POINT('Ctrl Pts',(4.71094372097749,-3.88380208938619,-0.00185818885717421));
#5259=CARTESIAN_POINT('Ctrl Pts',(4.74163086157564,-3.8881945038456,0.508719203379237));
#5260=CARTESIAN_POINT('Ctrl Pts',(4.77231800217378,-4.07403987422288,1.02216462871928));
#5261=CARTESIAN_POINT('Ctrl Pts',(4.80300514277192,-4.41013451264019,1.40301863392375));
#5262=CARTESIAN_POINT('Ctrl Pts',(4.84516157037211,-4.87184417392123,1.92621642895119));
#5263=CARTESIAN_POINT('Ctrl Pts',(4.8873179979723,-5.61710218276291,2.1991895235818));
#5264=CARTESIAN_POINT('Ctrl Pts',(4.92947442557249,-6.30751559099577,2.0979913527776));
#5265=CARTESIAN_POINT('Ctrl Pts',(4.97163085317269,-6.99792899922862,1.9967931819734));
#5266=CARTESIAN_POINT('Ctrl Pts',(5.01378728077288,-7.63349780685265,1.52142374573439));
#5267=CARTESIAN_POINT('Ctrl Pts',(5.05594370837307,-7.92563470581505,0.887729989802999));
#5268=CARTESIAN_POINT('Ctrl Pts',(5.09810013597325,-8.21777160477746,0.254036233871597));
#5269=CARTESIAN_POINT('Ctrl Pts',(5.14025656357344,-8.16647659507823,-0.537981841752198));
#5270=CARTESIAN_POINT('Ctrl Pts',(5.18241299117363,-7.7950407643039,-1.12869934416668));
#5271=CARTESIAN_POINT('Ctrl Pts',(5.22456941877382,-7.42360493352957,-1.71941684658117));
#5272=CARTESIAN_POINT('Ctrl Pts',(5.26672584637402,-6.73202828168015,-2.10883377578635));
#5273=CARTESIAN_POINT('Ctrl Pts',(5.30888227397421,-6.03432912097505,-2.12013090786587));
#5274=CARTESIAN_POINT('Ctrl Pts',(5.3510387015744,-5.33662996026994,-2.13142803994539));
#5275=CARTESIAN_POINT('Ctrl Pts',(5.3931951291746,-4.63280829070917,-1.76460537489925));
#5276=CARTESIAN_POINT('Ctrl Pts',(5.43535155677479,-4.24244241527317,-1.18622295181145));
#5277=CARTESIAN_POINT('Ctrl Pts',(5.46054894484236,-4.00911618220183,-0.840517037064096));
#5278=CARTESIAN_POINT('Ctrl Pts',(5.48574633290992,-3.88777492205943,-0.419229447894989));
#5279=CARTESIAN_POINT('Ctrl Pts',(5.51094372097749,-3.88587578853395,0.0010475127251217));
#5280=CARTESIAN_POINT('Ctrl Pts',(5.2890562790225,-3.88187782281943,0.00175000188907953));
#5281=CARTESIAN_POINT('Ctrl Pts',(5.25445105095617,-3.88698235634922,-0.572676552850085));
#5282=CARTESIAN_POINT('Ctrl Pts',(5.21984582288983,-4.12925905438439,-1.15089596655715));
#5283=CARTESIAN_POINT('Ctrl Pts',(5.18524059482349,-4.54624424461905,-1.54360861131074));
#5284=CARTESIAN_POINT('Ctrl Pts',(5.1430841672233,-5.05421968546235,-2.02201499963159));
#5285=CARTESIAN_POINT('Ctrl Pts',(5.10092773962312,-5.82146865948962,-2.22512283313927));
#5286=CARTESIAN_POINT('Ctrl Pts',(5.05877131202292,-6.49961296851871,-2.06070867007054));
#5287=CARTESIAN_POINT('Ctrl Pts',(5.01661488442273,-7.17775727754781,-1.89629450700181));
#5288=CARTESIAN_POINT('Ctrl Pts',(4.97445845682254,-7.76679692157875,-1.36435834735668));
#5289=CARTESIAN_POINT('Ctrl Pts',(4.93230202922235,-7.99927169304916,-0.706431906547451));
#5290=CARTESIAN_POINT('Ctrl Pts',(4.89014560162216,-8.23174646451957,-0.0485054657382238));
#5291=CARTESIAN_POINT('Ctrl Pts',(4.84798917402197,-8.10765636342946,0.735411256235103));
#5292=CARTESIAN_POINT('Ctrl Pts',(4.80583274642178,-7.68334592368299,1.28937187903092));
#5293=CARTESIAN_POINT('Ctrl Pts',(4.76367631882159,-7.25903548393652,1.84333250182674));
#5294=CARTESIAN_POINT('Ctrl Pts',(4.72151989122139,-6.53450470553368,2.16733702544503));
#5295=CARTESIAN_POINT('Ctrl Pts',(4.6793634636212,-5.83873509988996,2.11426747910681));
#5296=CARTESIAN_POINT('Ctrl Pts',(4.63720703602101,-5.14296549424625,2.0611979327686));
#5297=CARTESIAN_POINT('Ctrl Pts',(4.59505060842082,-4.47595706136166,1.63105431647387));
#5298=CARTESIAN_POINT('Ctrl Pts',(4.55289418082063,-4.14057263179942,1.01914827361007));
#5299=CARTESIAN_POINT('Ctrl Pts',(4.53161488022125,-3.97128062820059,0.71027645106943));
#5300=CARTESIAN_POINT('Ctrl Pts',(4.51033557962188,-3.88648402241563,0.355092876705326));
#5301=CARTESIAN_POINT('Ctrl Pts',(4.4890562790225,-3.88640241446317,-5.40837461397714E-5));
#5302=CARTESIAN_POINT('Origin',(6.,-6.,0.));
#5303=CARTESIAN_POINT('',(3.6890562790225,-3.88168480846505,-0.00170294642171713));
#5304=CARTESIAN_POINT('',(3.91094372097749,-3.87985545958303,0.000668395347130348));
#5305=CARTESIAN_POINT('',(6.,-3.883,2.59257727379495E-16));
#5306=CARTESIAN_POINT('Ctrl Pts',(3.91094372097749,-3.87985545958303,0.000668395347130348));
#5307=CARTESIAN_POINT('Ctrl Pts',(3.91320253504096,-3.87969984037501,0.0380697161946482));
#5308=CARTESIAN_POINT('Ctrl Pts',(3.91546134910444,-3.88060462371222,0.0754633564891892));
#5309=CARTESIAN_POINT('Ctrl Pts',(3.91772016316791,-3.88259359437381,0.112799239564616));
#5310=CARTESIAN_POINT('Ctrl Pts',(3.9598765907681,-3.91971391297379,0.809601812743023));
#5311=CARTESIAN_POINT('Ctrl Pts',(4.00203301836829,-4.33446812085637,1.48628693684409));
#5312=CARTESIAN_POINT('Ctrl Pts',(4.04418944596848,-4.9385323120656,1.83559796864891));
#5313=CARTESIAN_POINT('Ctrl Pts',(4.08634587356867,-5.54259650327483,2.18490900045374));
#5314=CARTESIAN_POINT('Ctrl Pts',(4.12850230116886,-6.33597067781071,2.20684593996233));
#5315=CARTESIAN_POINT('Ctrl Pts',(4.17065872876905,-6.95841419050323,1.8914480681416));
#5316=CARTESIAN_POINT('Ctrl Pts',(4.21281515636925,-7.58085770319576,1.57605019632088));
#5317=CARTESIAN_POINT('Ctrl Pts',(4.25497158396944,-8.03237055404493,0.923317513170838));
#5318=CARTESIAN_POINT('Ctrl Pts',(4.29712801156963,-8.10793815357666,0.229630781322297));
#5319=CARTESIAN_POINT('Ctrl Pts',(4.33928443916982,-8.18350575310838,-0.464055950526245));
#5320=CARTESIAN_POINT('Ctrl Pts',(4.38144086677001,-7.88312810132267,-1.19869673107329));
#5321=CARTESIAN_POINT('Ctrl Pts',(4.4235972943702,-7.34319511680599,-1.64071948645217));
#5322=CARTESIAN_POINT('Ctrl Pts',(4.46575372197039,-6.8032621322893,-2.08274224183105));
#5323=CARTESIAN_POINT('Ctrl Pts',(4.50791014957058,-6.02377381504164,-2.23214697204177));
#5324=CARTESIAN_POINT('Ctrl Pts',(4.55006657717077,-5.35866577743854,-2.02109474543042));
#5325=CARTESIAN_POINT('Ctrl Pts',(4.59222300477096,-4.69355773983544,-1.81004251881908));
#5326=CARTESIAN_POINT('Ctrl Pts',(4.63437943237116,-4.14282998187691,-1.23853333538567));
#5327=CARTESIAN_POINT('Ctrl Pts',(4.67653585997135,-3.95654675975784,-0.566067495956831));
#5328=CARTESIAN_POINT('Ctrl Pts',(4.6880051469734,-3.90586562144097,-0.383113100849401));
#5329=CARTESIAN_POINT('Ctrl Pts',(4.69947443397545,-3.8821604290332,-0.192685960170335));
#5330=CARTESIAN_POINT('Ctrl Pts',(4.71094372097749,-3.88380208938619,-0.00185818885717421));
#5331=CARTESIAN_POINT('Ctrl Pts',(4.4890562790225,-3.88640241446317,-5.40837461397714E-5));
#5332=CARTESIAN_POINT('Ctrl Pts',(4.46817915202169,-3.88632234888114,-0.348488853144316));
#5333=CARTESIAN_POINT('Ctrl Pts',(4.44730202502087,-3.96778535574421,-0.696888379539397));
#5334=CARTESIAN_POINT('Ctrl Pts',(4.42642489802006,-4.1309988177518,-1.00148286154596));
#5335=CARTESIAN_POINT('Ctrl Pts',(4.38426847041987,-4.46056985950631,-1.61653948440537));
#5336=CARTESIAN_POINT('Ctrl Pts',(4.34211204281968,-5.12347236925522,-2.05298426069133));
#5337=CARTESIAN_POINT('Ctrl Pts',(4.29995561521949,-5.81870785793641,-2.11264443303735));
#5338=CARTESIAN_POINT('Ctrl Pts',(4.2577991876193,-6.5139433466176,-2.17230460538337));
#5339=CARTESIAN_POINT('Ctrl Pts',(4.2156427600191,-7.24151181423107,-1.85518017378945));
#5340=CARTESIAN_POINT('Ctrl Pts',(4.17348633241891,-7.67105245172811,-1.3052651243282));
#5341=CARTESIAN_POINT('Ctrl Pts',(4.13132990481872,-8.10059308922514,-0.755350074866954));
#5342=CARTESIAN_POINT('Ctrl Pts',(4.08917347721853,-8.23210589660575,0.0273555924616259));
#5343=CARTESIAN_POINT('Ctrl Pts',(4.04701704961834,-8.00587597502505,0.687455390575113));
#5344=CARTESIAN_POINT('Ctrl Pts',(4.00486062201815,-7.77964605344434,1.3475551886886));
#5345=CARTESIAN_POINT('Ctrl Pts',(3.96270419441796,-7.19567340290233,1.885049117587));
#5346=CARTESIAN_POINT('Ctrl Pts',(3.92054776681776,-6.51911750444087,2.05588189296251));
#5347=CARTESIAN_POINT('Ctrl Pts',(3.87839133921757,-5.84256160597942,2.22671466833802));
#5348=CARTESIAN_POINT('Ctrl Pts',(3.83623491161738,-5.07342245959854,2.03088629019065));
#5349=CARTESIAN_POINT('Ctrl Pts',(3.79407848401719,-4.56093651792191,1.55731488008976));
#5350=CARTESIAN_POINT('Ctrl Pts',(3.75907108235229,-4.13535963133093,1.16405327055198));
#5351=CARTESIAN_POINT('Ctrl Pts',(3.7240636806874,-3.88676871644664,0.579262315211952));
#5352=CARTESIAN_POINT('Ctrl Pts',(3.6890562790225,-3.88168480846505,-0.00170294642171713));
#5353=CARTESIAN_POINT('Origin',(6.,-6.,0.));
#5354=CARTESIAN_POINT('',(2.8890562790225,-3.88141756531907,0.00162515511074018));
#5355=CARTESIAN_POINT('',(3.11094372097749,-3.88560636234646,0.00125599444870333));
#5356=CARTESIAN_POINT('',(6.,-3.883,2.59257727379495E-16));
#5357=CARTESIAN_POINT('Ctrl Pts',(3.11094372097749,-3.88560636234646,0.00125599444870333));
#5358=CARTESIAN_POINT('Ctrl Pts',(3.12693063610648,-3.8841502733519,0.267822688839656));
#5359=CARTESIAN_POINT('Ctrl Pts',(3.14291755123548,-3.93091517346986,0.533897324592317));
#5360=CARTESIAN_POINT('Ctrl Pts',(3.15890446636447,-4.02825317932317,0.779966685220892));
#5361=CARTESIAN_POINT('Ctrl Pts',(3.20106089396466,-4.28492700059471,1.4288351568594));
#5362=CARTESIAN_POINT('Ctrl Pts',(3.24321732156485,-4.89325670544289,1.93859861215253));
#5363=CARTESIAN_POINT('Ctrl Pts',(3.28537374916504,-5.57702321297396,2.07779310633982));
#5364=CARTESIAN_POINT('Ctrl Pts',(3.32753017676523,-6.26078972050503,2.21698760052711));
#5365=CARTESIAN_POINT('Ctrl Pts',(3.36968660436542,-7.01999303071899,1.98561313360857));
#5366=CARTESIAN_POINT('Ctrl Pts',(3.41184303196561,-7.50990817134806,1.48872793656901));
#5367=CARTESIAN_POINT('Ctrl Pts',(3.45399945956581,-7.99982331197713,0.991842739529444));
#5368=CARTESIAN_POINT('Ctrl Pts',(3.496155887166,-8.22045028302133,0.229446812368861));
#5369=CARTESIAN_POINT('Ctrl Pts',(3.53831231476619,-8.07161087736646,-0.452285228363516));
#5370=CARTESIAN_POINT('Ctrl Pts',(3.58046874236638,-7.9227714717116,-1.13401726909589));
#5371=CARTESIAN_POINT('Ctrl Pts',(3.62262516996657,-7.40446568935766,-1.73508542340006));
#5372=CARTESIAN_POINT('Ctrl Pts',(3.66478159756676,-6.75203621653659,-1.98256780062233));
#5373=CARTESIAN_POINT('Ctrl Pts',(3.70693802516695,-6.09960674371551,-2.2300501778446));
#5374=CARTESIAN_POINT('Ctrl Pts',(3.74909445276714,-5.31305358042728,-2.12394677798495));
#5375=CARTESIAN_POINT('Ctrl Pts',(3.79125088036734,-4.74952021344186,-1.71243506692724));
#5376=CARTESIAN_POINT('Ctrl Pts',(3.83114849390406,-4.21618193572383,-1.32297286274512));
#5377=CARTESIAN_POINT('Ctrl Pts',(3.87104610744078,-3.88260417410584,-0.659954127360146));
#5378=CARTESIAN_POINT('Ctrl Pts',(3.91094372097749,-3.87985545958303,0.000668395347130348));
#5379=CARTESIAN_POINT('Ctrl Pts',(3.6890562790225,-3.88168480846505,-0.00170294642171713));
#5380=CARTESIAN_POINT('Ctrl Pts',(3.68190725308721,-3.88064659973533,-0.120344591485258));
#5381=CARTESIAN_POINT('Ctrl Pts',(3.67475822715191,-3.8897635201934,-0.238826691185751));
#5382=CARTESIAN_POINT('Ctrl Pts',(3.66760920121662,-3.90960209601946,-0.355485504963693));
#5383=CARTESIAN_POINT('Ctrl Pts',(3.62545277361643,-4.02658635276603,-1.04340003786182));
#5384=CARTESIAN_POINT('Ctrl Pts',(3.58329634601624,-4.51638760323151,-1.66791466160366));
#5385=CARTESIAN_POINT('Ctrl Pts',(3.54113991841605,-5.1566059708734,-1.94546134706676));
#5386=CARTESIAN_POINT('Ctrl Pts',(3.49898349081586,-5.79682433851529,-2.22300803252987));
#5387=CARTESIAN_POINT('Ctrl Pts',(3.45682706321567,-6.58745982333359,-2.15358677971423));
#5388=CARTESIAN_POINT('Ctrl Pts',(3.41467063561547,-7.16951531363361,-1.76871910496289));
#5389=CARTESIAN_POINT('Ctrl Pts',(3.37251420801528,-7.75157080393361,-1.38385143021156));
#5390=CARTESIAN_POINT('Ctrl Pts',(3.33035778041509,-8.12504629971534,-0.683537333524543));
#5391=CARTESIAN_POINT('Ctrl Pts',(3.2882013528149,-8.12036096779767,0.0142375360740912));
#5392=CARTESIAN_POINT('Ctrl Pts',(3.24604492521471,-8.11567563588001,0.712012405672736));
#5393=CARTESIAN_POINT('Ctrl Pts',(3.20388849761452,-7.73282947626296,1.40724804818299));
#5394=CARTESIAN_POINT('Ctrl Pts',(3.16173207001432,-7.14565817952281,1.78426474421204));
#5395=CARTESIAN_POINT('Ctrl Pts',(3.11957564241413,-6.55848688278268,2.16128144024109));
#5396=CARTESIAN_POINT('Ctrl Pts',(3.07741921481394,-5.76699044891946,2.22007918978893));
#5397=CARTESIAN_POINT('Ctrl Pts',(3.03526278721375,-5.13055691347015,1.93396020110993));
#5398=CARTESIAN_POINT('Ctrl Pts',(2.99310635961356,-4.49412337802086,1.64784121243092));
#5399=CARTESIAN_POINT('Ctrl Pts',(2.95094993201337,-4.01275274098548,1.01680548552507));
#5400=CARTESIAN_POINT('Ctrl Pts',(2.90879350441318,-3.9050168620548,0.327382029349999));
#5401=CARTESIAN_POINT('Ctrl Pts',(2.90221442928295,-3.88820323523547,0.219788265529837));
#5402=CARTESIAN_POINT('Ctrl Pts',(2.89563535415273,-3.88048977537532,0.110772422866118));
#5403=CARTESIAN_POINT('Ctrl Pts',(2.8890562790225,-3.88141756531907,0.00162515511074018));
#5404=CARTESIAN_POINT('Origin',(6.,-6.,0.));
#5405=CARTESIAN_POINT('',(2.0890562790225,-3.88638481832281,0.000206967542925318));
#5406=CARTESIAN_POINT('',(2.31094372097749,-3.88425079107578,-0.00178855544584995));
#5407=CARTESIAN_POINT('',(6.,-3.883,2.59257727379495E-16));
#5408=CARTESIAN_POINT('Ctrl Pts',(2.31094372097749,-3.88425079107578,-0.00178855544584995));
#5409=CARTESIAN_POINT('Ctrl Pts',(2.34065873717201,-3.88827746358585,0.49288078299178));
#5410=CARTESIAN_POINT('Ctrl Pts',(2.37037375336652,-4.06150217415285,0.990091561638185));
#5411=CARTESIAN_POINT('Ctrl Pts',(2.40008876956103,-4.37841802272573,1.36623769466599));
#5412=CARTESIAN_POINT('Ctrl Pts',(2.44224519716122,-4.82802370149306,1.89987284802682));
#5413=CARTESIAN_POINT('Ctrl Pts',(2.48440162476141,-5.56683427812707,2.18984308956855));
#5414=CARTESIAN_POINT('Ctrl Pts',(2.5265580523616,-6.25938433842444,2.10448409909473));
#5415=CARTESIAN_POINT('Ctrl Pts',(2.56871447996179,-6.95193439872182,2.01912510862091));
#5416=CARTESIAN_POINT('Ctrl Pts',(2.61087090756198,-7.59822394268257,1.55843688613156));
#5417=CARTESIAN_POINT('Ctrl Pts',(2.65302733516218,-7.9047977871553,0.931600206785907));
#5418=CARTESIAN_POINT('Ctrl Pts',(2.69518376276237,-8.21137163162803,0.304763527440254));
#5419=CARTESIAN_POINT('Ctrl Pts',(2.73734019036256,-8.17822977661274,-0.488221608761689));
#5420=CARTESIAN_POINT('Ctrl Pts',(2.77949661796275,-7.82042066249784,-1.0872912055028));
#5421=CARTESIAN_POINT('Ctrl Pts',(2.82165304556294,-7.46261154838294,-1.6863608022439));
#5422=CARTESIAN_POINT('Ctrl Pts',(2.86380947316313,-6.78013517516843,-2.09151485952416));
#5423=CARTESIAN_POINT('Ctrl Pts',(2.90596590076332,-6.08287776867917,-2.11878852909447));
#5424=CARTESIAN_POINT('Ctrl Pts',(2.94812232836351,-5.3856203621899,-2.14606219866477));
#5425=CARTESIAN_POINT('Ctrl Pts',(2.9902787559637,-4.67358192242587,-1.7954554805251));
#5426=CARTESIAN_POINT('Ctrl Pts',(3.0324351835639,-4.2700716713913,-1.22616537746331));
#5427=CARTESIAN_POINT('Ctrl Pts',(3.0586046960351,-4.01958397241328,-0.872766256619923));
#5428=CARTESIAN_POINT('Ctrl Pts',(3.08477420850629,-3.88798988279394,-0.435095883132698));
#5429=CARTESIAN_POINT('Ctrl Pts',(3.11094372097749,-3.88560636234646,0.00125599444870333));
#5430=CARTESIAN_POINT('Ctrl Pts',(2.8890562790225,-3.88141756531907,0.00162515511074018));
#5431=CARTESIAN_POINT('Ctrl Pts',(2.85347892655253,-3.88643473098346,-0.588605346776316));
#5432=CARTESIAN_POINT('Ctrl Pts',(2.81790157408257,-4.14414542594115,-1.18267907400726));
#5433=CARTESIAN_POINT('Ctrl Pts',(2.78232422161261,-4.58197906344156,-1.5764992762549));
#5434=CARTESIAN_POINT('Ctrl Pts',(2.74016779401242,-5.10077826458496,-2.04314594024041));
#5435=CARTESIAN_POINT('Ctrl Pts',(2.69801136641223,-5.87247778769773,-2.22862808276713));
#5436=CARTESIAN_POINT('Ctrl Pts',(2.65585493881203,-6.54667861130499,-2.04872541582711));
#5437=CARTESIAN_POINT('Ctrl Pts',(2.61369851121184,-7.22087943491225,-1.86882274888709));
#5438=CARTESIAN_POINT('Ctrl Pts',(2.57154208361165,-7.797581559014,-1.32353527248033));
#5439=CARTESIAN_POINT('Ctrl Pts',(2.52938565601146,-8.01492676931713,-0.660457007976325));
#5440=CARTESIAN_POINT('Ctrl Pts',(2.48722922841127,-8.23227197962026,0.00262125652767495));
#5441=CARTESIAN_POINT('Ctrl Pts',(2.44507280081108,-8.09026027612478,0.783490309128911));
#5442=CARTESIAN_POINT('Ctrl Pts',(2.40291637321089,-7.65337370033519,1.32758757464938));
#5443=CARTESIAN_POINT('Ctrl Pts',(2.3607599456107,-7.2164871245456,1.87168484016984));
#5444=CARTESIAN_POINT('Ctrl Pts',(2.3186035180105,-6.48472567646189,2.17901031860954));
#5445=CARTESIAN_POINT('Ctrl Pts',(2.27644709041031,-5.79035403900129,2.11001939707077));
#5446=CARTESIAN_POINT('Ctrl Pts',(2.23429066281012,-5.09598240154068,2.04102847553199));
#5447=CARTESIAN_POINT('Ctrl Pts',(2.19213423520993,-4.43900057470318,1.59572115401476));
#5448=CARTESIAN_POINT('Ctrl Pts',(2.14997780760974,-4.11771868783986,0.976294242006309));
#5449=CARTESIAN_POINT('Ctrl Pts',(2.129670631414,-3.96295396377662,0.67791005343511));
#5450=CARTESIAN_POINT('Ctrl Pts',(2.10936345521825,-3.88608659904271,0.339122353597826));
#5451=CARTESIAN_POINT('Ctrl Pts',(2.0890562790225,-3.88638481832281,0.000206967542925318));
#5452=CARTESIAN_POINT('Origin',(6.,-6.,0.));
#5453=CARTESIAN_POINT('',(1.2890562790225,-3.88215585431528,-0.00180833227560233));
#5454=CARTESIAN_POINT('',(1.51094372097749,-3.87968050865492,0.000387557652718817));
#5455=CARTESIAN_POINT('',(6.,-3.883,2.59257727379495E-16));
#5456=CARTESIAN_POINT('Ctrl Pts',(1.51094372097749,-3.87968050865492,0.000387557652718817));
#5457=CARTESIAN_POINT('Ctrl Pts',(1.51223041063733,-3.87962643184165,0.0216877999309881));
#5458=CARTESIAN_POINT('Ctrl Pts',(1.51351710029718,-3.8799198812182,0.0429865156964861));
#5459=CARTESIAN_POINT('Ctrl Pts',(1.51480378995702,-3.88056546385779,0.0642745521975925));
#5460=CARTESIAN_POINT('Ctrl Pts',(1.55696021755721,-3.90171699608445,0.761744655143333));
#5461=CARTESIAN_POINT('Ctrl Pts',(1.5991166451574,-4.30086437795335,1.44775115029935));
#5462=CARTESIAN_POINT('Ctrl Pts',(1.64127307275759,-4.89676984071834,1.81080544827727));
#5463=CARTESIAN_POINT('Ctrl Pts',(1.68342950035778,-5.49267530348333,2.17385974625519));
#5464=CARTESIAN_POINT('Ctrl Pts',(1.72558592795797,-6.2853388471444,2.21396184705501));
#5465=CARTESIAN_POINT('Ctrl Pts',(1.76774235555817,-6.91484266441608,1.91290265527438));
#5466=CARTESIAN_POINT('Ctrl Pts',(1.80989878315836,-7.54434648168775,1.61184346349375));
#5467=CARTESIAN_POINT('Ctrl Pts',(1.85205521075855,-8.01069057257003,0.969622979132674));
#5468=CARTESIAN_POINT('Ctrl Pts',(1.89421163835874,-8.10212596526366,0.277848924816985));
#5469=CARTESIAN_POINT('Ctrl Pts',(1.93636806595893,-8.19356135795729,-0.413925129498698));
#5470=CARTESIAN_POINT('Ctrl Pts',(1.97852449355912,-7.91008805246229,-1.15525275376899));
#5471=CARTESIAN_POINT('Ctrl Pts',(2.02068092115931,-7.38042040080226,-1.60952571148568));
#5472=CARTESIAN_POINT('Ctrl Pts',(2.0628373487595,-6.85075274914223,-2.06379866920236));
#5473=CARTESIAN_POINT('Ctrl Pts',(2.10499377635969,-6.07489075131718,-2.23101696036544));
#5474=CARTESIAN_POINT('Ctrl Pts',(2.14715020395988,-5.40512342384882,-2.03525316220135));
#5475=CARTESIAN_POINT('Ctrl Pts',(2.18930663156007,-4.73535609638045,-1.83948936403726));
#5476=CARTESIAN_POINT('Ctrl Pts',(2.23146305916027,-4.17168343926878,-1.280743476546));
#5477=CARTESIAN_POINT('Ctrl Pts',(2.27361948676046,-3.97004750116327,-0.6127205002104));
#5478=CARTESIAN_POINT('Ctrl Pts',(2.28606089816614,-3.9105397154483,-0.415570287297211));
#5479=CARTESIAN_POINT('Ctrl Pts',(2.29850230957181,-3.88256485932444,-0.20890218139817));
#5480=CARTESIAN_POINT('Ctrl Pts',(2.31094372097749,-3.88425079107578,-0.00178855544584995));
#5481=CARTESIAN_POINT('Ctrl Pts',(2.0890562790225,-3.88638481832281,0.000206967542925318));
#5482=CARTESIAN_POINT('Ctrl Pts',(2.06720702761806,-3.88670568361505,-0.364444789223636));
#5483=CARTESIAN_POINT('Ctrl Pts',(2.04535777621361,-3.97635662359167,-0.729244360841879));
#5484=CARTESIAN_POINT('Ctrl Pts',(2.02350852480917,-4.15442617570082,-1.04402620399982));
#5485=CARTESIAN_POINT('Ctrl Pts',(1.98135209720898,-4.49799749731423,-1.65137323549784));
#5486=CARTESIAN_POINT('Ctrl Pts',(1.93919566960879,-5.17072208743017,-2.0725207959942));
#5487=CARTESIAN_POINT('Ctrl Pts',(1.8970392420086,-5.8671416077804,-2.11624232759768));
#5488=CARTESIAN_POINT('Ctrl Pts',(1.8548828144084,-6.56356112813062,-2.15996385920116));
#5489=CARTESIAN_POINT('Ctrl Pts',(1.81272638680821,-7.28367557871513,-1.82625936191177));
#5490=CARTESIAN_POINT('Ctrl Pts',(1.77056995920802,-7.70050877250907,-1.26665057227176));
#5491=CARTESIAN_POINT('Ctrl Pts',(1.72841353160783,-8.11734196630301,-0.707041782631743));
#5492=CARTESIAN_POINT('Ctrl Pts',(1.68625710400764,-8.23089390330638,0.0784712993588993));
#5493=CARTESIAN_POINT('Ctrl Pts',(1.64410067640745,-7.98960494718644,0.733216263819768));
#5494=CARTESIAN_POINT('Ctrl Pts',(1.60194424880726,-7.74831599106649,1.38796122828064));
#5495=CARTESIAN_POINT('Ctrl Pts',(1.55978782120707,-7.15218614182322,1.91193807521173));
#5496=CARTESIAN_POINT('Ctrl Pts',(1.51763139360688,-6.47189514288099,2.06723137262971));
#5497=CARTESIAN_POINT('Ctrl Pts',(1.47547496600669,-5.79160414393876,2.22252467004768));
#5498=CARTESIAN_POINT('Ctrl Pts',(1.4333185384065,-5.02715199529757,2.00913441795253));
#5499=CARTESIAN_POINT('Ctrl Pts',(1.3911621108063,-4.52564668340792,1.52394857057864));
#5500=CARTESIAN_POINT('Ctrl Pts',(1.35712683354504,-4.12075297419606,1.13223049154154));
#5501=CARTESIAN_POINT('Ctrl Pts',(1.32309155628377,-3.88725457516647,0.563349260688335));
#5502=CARTESIAN_POINT('Ctrl Pts',(1.2890562790225,-3.88215585431528,-0.00180833227560233));
#5503=CARTESIAN_POINT('Origin',(6.,-6.,0.));
#5504=CARTESIAN_POINT('',(0.4890562790225,-3.88098062526521,0.00140302826277638));
#5505=CARTESIAN_POINT('',(0.710943720977493,-3.88529148023119,0.00143577679747337));
#5506=CARTESIAN_POINT('',(6.,-3.883,2.59257727379495E-16));
#5507=CARTESIAN_POINT('',(0.,-7.61992569438872,1.36291222925734));
#5508=CARTESIAN_POINT('Ctrl Pts',(0.4890562790225,-3.88098062526521,0.00140302826277638));
#5509=CARTESIAN_POINT('Ctrl Pts',(0.452506802148906,-3.88578409771184,-0.604476981624192));
#5510=CARTESIAN_POINT('Ctrl Pts',(0.415957325275312,-4.15953906766724,-1.21398517371684));
#5511=CARTESIAN_POINT('Ctrl Pts',(0.379407848401718,-4.61847166921745,-1.60833849276868));
#5512=CARTESIAN_POINT('Ctrl Pts',(0.337251420801527,-5.14780780876139,-2.06318842676363));
#5513=CARTESIAN_POINT('Ctrl Pts',(0.295094993201337,-5.92349464593687,-2.23180749898577));
#5514=CARTESIAN_POINT('Ctrl Pts',(0.252938565601146,-6.59343701884389,-2.03607518357452));
#5515=CARTESIAN_POINT('Ctrl Pts',(0.210782138000955,-7.26337939175092,-1.84034286816327));
#5516=CARTESIAN_POINT('Ctrl Pts',(0.168625710400764,-7.82757730038949,-1.28025916511862));
#5517=CARTESIAN_POINT('Ctrl Pts',(0.126469282800573,-8.02952750753659,-0.613533042485344));
#5518=CARTESIAN_POINT('Ctrl Pts',(0.0843128552003817,-8.23147771468369,
0.0531930801479328));
#5519=CARTESIAN_POINT('Ctrl Pts',(0.0421564276001906,-8.07118022033932,
0.826561622369841));
#5520=CARTESIAN_POINT('Ctrl Pts',(-4.10547488943358E-16,-7.61992569438872,
1.36291222925734));
#5521=CARTESIAN_POINT('',(2.70473896144179E-15,-4.37709039209165,1.36522613564372));
#5522=CARTESIAN_POINT('Origin',(0.,-6.,0.));
#5523=CARTESIAN_POINT('Ctrl Pts',(1.80411241501588E-15,-4.37708920932832,
1.36522705282968));
#5524=CARTESIAN_POINT('Ctrl Pts',(0.0412138930502395,-4.8171154211057,1.88675622363143));
#5525=CARTESIAN_POINT('Ctrl Pts',(0.0824277861004773,-5.53232983704421,
2.17777740054626));
#5526=CARTESIAN_POINT('Ctrl Pts',(0.123641679150715,-6.21123416498923,2.10968102048252));
#5527=CARTESIAN_POINT('Ctrl Pts',(0.165798106750906,-6.90566458711858,2.04002732112213));
#5528=CARTESIAN_POINT('Ctrl Pts',(0.207954534351097,-7.56210515530846,1.59464268056525));
#5529=CARTESIAN_POINT('Ctrl Pts',(0.250110961951288,-7.88289993702619,0.975083106675219));
#5530=CARTESIAN_POINT('Ctrl Pts',(0.292267389551479,-8.20369471874392,0.355523532785185));
#5531=CARTESIAN_POINT('Ctrl Pts',(0.33442381715167,-8.18884371398951,-0.438210974438008));
#5532=CARTESIAN_POINT('Ctrl Pts',(0.376580244751861,-7.84487777104374,-1.04536577050709));
#5533=CARTESIAN_POINT('Ctrl Pts',(0.418736672352052,-7.50091182809796,-1.65252056657617));
#5534=CARTESIAN_POINT('Ctrl Pts',(0.460893099952243,-6.82783094696082,-2.07309565149114));
#5535=CARTESIAN_POINT('Ctrl Pts',(0.503049527552434,-6.13136608707291,-2.11630681992121));
#5536=CARTESIAN_POINT('Ctrl Pts',(0.545205955152625,-5.43490122718498,-2.15951798835128));
#5537=CARTESIAN_POINT('Ctrl Pts',(0.587362382752816,-4.71505238854628,-1.82536524029645));
#5538=CARTESIAN_POINT('Ctrl Pts',(0.629518810353007,-4.2986172899441,-1.26547903592209));
#5539=CARTESIAN_POINT('Ctrl Pts',(0.656660447227835,-4.03050324727928,-0.905006649730477));
#5540=CARTESIAN_POINT('Ctrl Pts',(0.683802084102664,-3.8881599727947,-0.450963450951839));
#5541=CARTESIAN_POINT('Ctrl Pts',(0.710943720977493,-3.88529148023119,0.00143577679747337));
#5542=CARTESIAN_POINT('Origin',(-1.7667098902285,-6.,0.));
#5543=CARTESIAN_POINT('',(10.5667098902285,-3.44386948695903,0.000692352191159762));
#5544=CARTESIAN_POINT('',(10.6332901097715,-3.43705236943178,-0.00151513564181791));
#5545=CARTESIAN_POINT('',(-1.7667098902285,-3.44,1.9679933794996E-13));
#5546=CARTESIAN_POINT('',(11.,-8.47299490241841,0.661737268568548));
#5547=CARTESIAN_POINT('Ctrl Pts',(10.6332901097715,-3.43705236943178,-0.00151513564181784));
#5548=CARTESIAN_POINT('Ctrl Pts',(10.6712138846473,-3.44184769772038,0.758560196074207));
#5549=CARTESIAN_POINT('Ctrl Pts',(10.7512940871233,-4.19985142761009,2.37288109075158));
#5550=CARTESIAN_POINT('Ctrl Pts',(10.8735307171994,-6.94276063434935,2.8696483143193));
#5551=CARTESIAN_POINT('Ctrl Pts',(10.9578435723998,-8.2538964667147,1.48053551427594));
#5552=CARTESIAN_POINT('Ctrl Pts',(11.,-8.47299490241841,0.661737268568548));
#5553=CARTESIAN_POINT('',(11.,-8.47735530983487,-0.663092355832106));
#5554=CARTESIAN_POINT('Origin',(11.,-6.,0.));
#5555=CARTESIAN_POINT('Ctrl Pts',(10.5667098902285,-3.44386948695903,0.000692352191160109));
#5556=CARTESIAN_POINT('Ctrl Pts',(10.5856131785684,-3.4429055464256,0.382134963423751));
#5557=CARTESIAN_POINT('Ctrl Pts',(10.6466728945085,-3.70136760183046,1.61303222180456));
#5558=CARTESIAN_POINT('Ctrl Pts',(10.7498890380487,-5.60254915406858,2.99513384905324));
#5559=CARTESIAN_POINT('Ctrl Pts',(10.8754157862993,-8.27098793310559,1.97617764674277));
#5560=CARTESIAN_POINT('Ctrl Pts',(10.9587861069498,-8.68954097008596,0.134309514573586));
#5561=CARTESIAN_POINT('Ctrl Pts',(11.,-8.4773570382127,-0.663092892961434));
#5562=CARTESIAN_POINT('Origin',(-1.7667098902285,-6.,0.));
#5563=CARTESIAN_POINT('',(9.76670989022852,-3.43982213984121,-0.00227838982848949));
#5564=CARTESIAN_POINT('',(9.8332901097715,-3.43981019619369,0.0022738699535656));
#5565=CARTESIAN_POINT('',(-1.7667098902285,-3.44,1.9679933794996E-13));
#5566=CARTESIAN_POINT('Ctrl Pts',(9.8332901097715,-3.43981019619369,0.00227386995356616));
#5567=CARTESIAN_POINT('Ctrl Pts',(9.84278555811261,-3.43807597231295,0.193098490195483));
#5568=CARTESIAN_POINT('Ctrl Pts',(9.89443743405392,-3.54439859556582,1.22920418622825));
#5569=CARTESIAN_POINT('Ctrl Pts',(9.98824573759542,-4.95320971865872,2.83433293290292));
#5570=CARTESIAN_POINT('Ctrl Pts',(10.114715020396,-7.80326121920459,2.4243168480084));
#5571=CARTESIAN_POINT('Ctrl Pts',(10.2411843031966,-9.01549208379667,-0.187132795629694));
#5572=CARTESIAN_POINT('Ctrl Pts',(10.3676535859971,-7.48974052152724,-2.62891886486708));
#5573=CARTESIAN_POINT('Ctrl Pts',(10.4941228687977,-4.61024985438304,-2.68279494587922));
#5574=CARTESIAN_POINT('Ctrl Pts',(10.5826683767225,-3.47900431032775,-1.0154815268328));
#5575=CARTESIAN_POINT('Ctrl Pts',(10.6290574570471,-3.4365171653438,-0.0863467467902525));
#5576=CARTESIAN_POINT('Ctrl Pts',(10.6332901097715,-3.43705236943178,-0.00151513564181784));
#5577=CARTESIAN_POINT('Ctrl Pts',(9.76670989022852,-3.43982213984121,-0.00227838982848942));
#5578=CARTESIAN_POINT('Ctrl Pts',(9.79934127963391,-3.44577993040473,0.653508085119705));
#5579=CARTESIAN_POINT('Ctrl Pts',(9.8741290966395,-4.03530828415894,2.16602520880728));
#5580=CARTESIAN_POINT('Ctrl Pts',(9.99107334124527,-6.57463978426254,2.96628135292037));
#5581=CARTESIAN_POINT('Ctrl Pts',(10.1175426240459,-8.79891519692859,1.13796717239844));
#5582=CARTESIAN_POINT('Ctrl Pts',(10.2440119068464,-8.4815071817026,-1.72375621929785));
#5583=CARTESIAN_POINT('Ctrl Pts',(10.370481189647,-5.91044069571119,-3.02010639410425));
#5584=CARTESIAN_POINT('Ctrl Pts',(10.4780471841077,-3.79308023070163,-1.7899877019098));
#5585=CARTESIAN_POINT('Ctrl Pts',(10.5434567509682,-3.44505524062577,-0.468524325845745));
#5586=CARTESIAN_POINT('Ctrl Pts',(10.5667098902285,-3.44386948695903,0.000692352191160109));
#5587=CARTESIAN_POINT('Origin',(-1.7667098902285,-6.,0.));
#5588=CARTESIAN_POINT('',(8.96670989022851,-3.43689094140915,0.00141529279526265));
#5589=CARTESIAN_POINT('',(9.0332901097715,-3.44394015329315,-0.000687443883765837));
#5590=CARTESIAN_POINT('',(-1.7667098902285,-3.44,1.9679933794996E-13));
#5591=CARTESIAN_POINT('Ctrl Pts',(9.0332901097715,-3.44394015329315,-0.0006874438837658));
#5592=CARTESIAN_POINT('Ctrl Pts',(9.05651365917813,-3.44507664468085,0.467936431888932));
#5593=CARTESIAN_POINT('Ctrl Pts',(9.12189363618495,-3.79229911794252,1.7887946585363));
#5594=CARTESIAN_POINT('Ctrl Pts',(9.22943004079198,-5.90841299622533,3.0200385622781));
#5595=CARTESIAN_POINT('Ctrl Pts',(9.35589932359255,-8.48026503905977,1.72548764368831));
#5596=CARTESIAN_POINT('Ctrl Pts',(9.48236860639313,-8.79972666043973,-1.1360152599871));
#5597=CARTESIAN_POINT('Ctrl Pts',(9.60883788919369,-6.57670152087419,-2.96588225471199));
#5598=CARTESIAN_POINT('Ctrl Pts',(9.72581172365316,-4.03617235544237,-2.1671874966241));
#5599=CARTESIAN_POINT('Ctrl Pts',(9.80062913051242,-3.44577531212764,-0.654095238691659));
#5600=CARTESIAN_POINT('Ctrl Pts',(9.8332901097715,-3.43981019619369,0.00227386995356616));
#5601=CARTESIAN_POINT('Ctrl Pts',(8.96670989022851,-3.43689094140915,0.00141529279526262));
#5602=CARTESIAN_POINT('Ctrl Pts',(8.97091295309924,-3.43632903198528,0.0856328825033177));
#5603=CARTESIAN_POINT('Ctrl Pts',(9.01727244357015,-3.4781806728961,1.01398188137752));
#5604=CARTESIAN_POINT('Ctrl Pts',(9.10578836164126,-4.60885239449141,2.68211248963539));
#5605=CARTESIAN_POINT('Ctrl Pts',(9.23225764444184,-7.48766074739694,2.6298070334431));
#5606=CARTESIAN_POINT('Ctrl Pts',(9.3587269272424,-9.01548944052047,0.189313422437645));
#5607=CARTESIAN_POINT('Ctrl Pts',(9.48519621004299,-7.80488452630467,-2.42309995159429));
#5608=CARTESIAN_POINT('Ctrl Pts',(9.61166549284354,-4.95521961969974,-2.83504085634446));
#5609=CARTESIAN_POINT('Ctrl Pts',(9.70550338623873,-3.54480869101683,-1.23041260512691));
#5610=CARTESIAN_POINT('Ctrl Pts',(9.75718485203372,-3.43808307252877,-0.193701168181872));
#5611=CARTESIAN_POINT('Ctrl Pts',(9.76670989022852,-3.43982213984121,-0.00227838982848942));
#5612=CARTESIAN_POINT('Origin',(-1.7667098902285,-6.,0.));
#5613=CARTESIAN_POINT('',(8.16670989022851,-3.44373997328344,0.000990877584209626));
#5614=CARTESIAN_POINT('',(8.2332901097715,-3.43735861323487,-0.00167649580848317));
#5615=CARTESIAN_POINT('',(-1.7667098902285,-3.44,1.9679933794996E-13));
#5616=CARTESIAN_POINT('Ctrl Pts',(8.2332901097715,-3.43735861323486,-0.0016764958084832));
#5617=CARTESIAN_POINT('Ctrl Pts',(8.27024176024366,-3.44299005962199,0.739085989948098));
#5618=CARTESIAN_POINT('Ctrl Pts',(8.349349838316,-4.16926208645861,2.33458270048732));
#5619=CARTESIAN_POINT('Ctrl Pts',(8.47061434398855,-6.87308161737107,2.89253294855792));
#5620=CARTESIAN_POINT('Ctrl Pts',(8.59708362678911,-8.90008601701954,0.847655336961254));
#5621=CARTESIAN_POINT('Ctrl Pts',(8.72355290958969,-8.29345566941167,-1.96699747432336));
#5622=CARTESIAN_POINT('Ctrl Pts',(8.85002219239025,-5.60408579766473,-2.99537486433416));
#5623=CARTESIAN_POINT('Ctrl Pts',(8.9532679257842,-3.7020811956009,-1.61424699855408));
#5624=CARTESIAN_POINT('Ctrl Pts',(9.01435723157795,-3.44301363458428,-0.3827306278625));
#5625=CARTESIAN_POINT('Ctrl Pts',(9.0332901097715,-3.44394015329315,-0.0006874438837658));
#5626=CARTESIAN_POINT('Ctrl Pts',(8.16670989022851,-3.44373997328344,0.000990877584210043));
#5627=CARTESIAN_POINT('Ctrl Pts',(8.18464105416476,-3.44246936070189,0.36274984291225));
#5628=CARTESIAN_POINT('Ctrl Pts',(8.2447286457012,-3.68275714716096,1.57339810621675));
#5629=CARTESIAN_POINT('Ctrl Pts',(8.34697266483782,-5.5335046738129,2.98519695992403));
#5630=CARTESIAN_POINT('Ctrl Pts',(8.47344194763839,-8.24639557638579,2.02057558976858));
#5631=CARTESIAN_POINT('Ctrl Pts',(8.59991123043898,-8.91928310048972,-0.77897683272588));
#5632=CARTESIAN_POINT('Ctrl Pts',(8.72638051323954,-6.94110269497493,-2.87112251928));
#5633=CARTESIAN_POINT('Ctrl Pts',(8.8486467331694,-4.20243074754735,-2.37305761672387));
#5634=CARTESIAN_POINT('Ctrl Pts',(8.92875652549905,-3.44196494433624,-0.759063671507021));
#5635=CARTESIAN_POINT('Ctrl Pts',(8.96670989022851,-3.43689094140915,0.00141529279526262));
#5636=CARTESIAN_POINT('Origin',(-1.7667098902285,-6.,0.));
#5637=CARTESIAN_POINT('',(7.36670989022851,-3.44040316956898,-0.00228610733910742));
#5638=CARTESIAN_POINT('',(7.4332901097715,-3.43921965943194,0.00222060329450378));
#5639=CARTESIAN_POINT('',(-1.7667098902285,-3.44,1.9679933794996E-13));
#5640=CARTESIAN_POINT('Ctrl Pts',(7.4332901097715,-3.43921965943194,0.00222060329450373));
#5641=CARTESIAN_POINT('Ctrl Pts',(7.44181343370898,-3.43766552072112,0.173408608068247));
#5642=CARTESIAN_POINT('Ctrl Pts',(7.49249318524665,-3.53110044716585,1.1896069546148));
#5643=CARTESIAN_POINT('Ctrl Pts',(7.58532936438453,-4.88860486534565,2.80959413389628));
#5644=CARTESIAN_POINT('Ctrl Pts',(7.7117986471851,-7.74719543871252,2.46502057642963));
#5645=CARTESIAN_POINT('Ctrl Pts',(7.83826792998567,-9.01911774919456,-0.118094722276079));
#5646=CARTESIAN_POINT('Ctrl Pts',(7.96473721278625,-7.54930996179144,-2.5939654930144));
#5647=CARTESIAN_POINT('Ctrl Pts',(8.09120649558682,-4.67253825597884,-2.71419668832455));
#5648=CARTESIAN_POINT('Ctrl Pts',(8.18072412791524,-3.48957571549017,-1.05464412437998));
#5649=CARTESIAN_POINT('Ctrl Pts',(8.22808533264346,-3.43656540310815,-0.106015641527535));
#5650=CARTESIAN_POINT('Ctrl Pts',(8.2332901097715,-3.43735861323486,-0.0016764958084832));
#5651=CARTESIAN_POINT('Ctrl Pts',(7.36670989022851,-3.44040316956898,-0.00228610733910735));
#5652=CARTESIAN_POINT('Ctrl Pts',(7.39836915523028,-3.44608356882379,0.634333467603688));
#5653=CARTESIAN_POINT('Ctrl Pts',(7.47218484783223,-4.00717014687453,2.12759383120187));
#5654=CARTESIAN_POINT('Ctrl Pts',(7.58815696803439,-6.50654071121665,2.97866333871112));
#5655=CARTESIAN_POINT('Ctrl Pts',(7.71462625083495,-8.77213940010801,1.20177448985872));
#5656=CARTESIAN_POINT('Ctrl Pts',(7.84109553363553,-8.52029469802955,-1.66647334565703));
#5657=CARTESIAN_POINT('Ctrl Pts',(7.96756481643611,-5.9797125579978,-3.02135850191909));
#5658=CARTESIAN_POINT('Ctrl Pts',(8.07610293530042,-3.81515252211499,-1.82939789701246));
#5659=CARTESIAN_POINT('Ctrl Pts',(8.14248462656456,-3.4454565893889,-0.487750753970042));
#5660=CARTESIAN_POINT('Ctrl Pts',(8.16670989022851,-3.44373997328344,0.000990877584210043));
#5661=CARTESIAN_POINT('Origin',(-1.7667098902285,-6.,0.));
#5662=CARTESIAN_POINT('',(6.56670989022851,-3.43650398705703,0.0011262704457668));
#5663=CARTESIAN_POINT('',(6.6332901097715,-3.44406314725449,-0.000379914237597221));
#5664=CARTESIAN_POINT('',(-1.7667098902285,-3.44,1.9679933794996E-13));
#5665=CARTESIAN_POINT('Ctrl Pts',(6.6332901097715,-3.44406314725449,-0.000379914237597229));
#5666=CARTESIAN_POINT('Ctrl Pts',(6.6555415347745,-3.44466328028651,0.448681698616593));
#5667=CARTESIAN_POINT('Ctrl Pts',(6.7199493873777,-3.77077864344925,1.749327874684));
#5668=CARTESIAN_POINT('Ctrl Pts',(6.8265136675811,-5.83926938364069,3.01714832455762));
#5669=CARTESIAN_POINT('Ctrl Pts',(6.95298295038165,-8.44009396559778,1.78184168277249));
#5670=CARTESIAN_POINT('Ctrl Pts',(7.07945223318224,-8.82501323416001,-1.07159627207705));
#5671=CARTESIAN_POINT('Ctrl Pts',(7.2059215159828,-6.6444731702528,-2.95189306651605));
#5672=CARTESIAN_POINT('Ctrl Pts',(7.3238674748459,-4.06507178369403,-2.20544952615896));
#5673=CARTESIAN_POINT('Ctrl Pts',(7.39965700610879,-3.4453523030755,-0.673288617356633));
#5674=CARTESIAN_POINT('Ctrl Pts',(7.4332901097715,-3.43921965943194,0.00222060329450373));
#5675=CARTESIAN_POINT('Ctrl Pts',(6.56670989022851,-3.43650398705703,0.00112627044576692));
#5676=CARTESIAN_POINT('Ctrl Pts',(6.56994082869561,-3.43614573843741,0.0658393894794153));
#5677=CARTESIAN_POINT('Ctrl Pts',(6.61532819476289,-3.46761353360699,0.974558132719011));
#5678=CARTESIAN_POINT('Ctrl Pts',(6.70287198843037,-4.54778863223406,2.64954730489951));
#5679=CARTESIAN_POINT('Ctrl Pts',(6.82934127123096,-7.42703945423727,2.66318928610364));
#5680=CARTESIAN_POINT('Ctrl Pts',(6.95581055403151,-9.01036300717914,0.25832797484807));
#5681=CARTESIAN_POINT('Ctrl Pts',(7.0822798368321,-7.85990684631327,-2.38112689720535));
#5682=CARTESIAN_POINT('Ctrl Pts',(7.20874911963266,-5.02042660634255,-2.85822580353484));
#5683=CARTESIAN_POINT('Ctrl Pts',(7.30355913743147,-3.55864292974095,-1.27003728223635));
#5684=CARTESIAN_POINT('Ctrl Pts',(7.35621272763009,-3.4385197375121,-0.213368051002073));
#5685=CARTESIAN_POINT('Ctrl Pts',(7.36670989022851,-3.44040316956898,-0.00228610733910735));
#5686=CARTESIAN_POINT('Origin',(-1.7667098902285,-6.,0.));
#5687=CARTESIAN_POINT('',(5.76670989022851,-3.44347757139674,0.00126671354594904));
#5688=CARTESIAN_POINT('',(5.8332901097715,-3.43786500993883,-0.00188959581389439));
#5689=CARTESIAN_POINT('',(-1.7667098902285,-3.44,1.9679933794996E-13));
#5690=CARTESIAN_POINT('Ctrl Pts',(5.8332901097715,-3.43786500993883,-0.00188959581389444));
#5691=CARTESIAN_POINT('Ctrl Pts',(5.86926963584003,-3.4438412047324,0.719757477813235));
#5692=CARTESIAN_POINT('Ctrl Pts',(5.94740558950874,-4.1378402398782,2.29700877488544));
#5693=CARTESIAN_POINT('Ctrl Pts',(6.06769797077765,-6.80660452923693,2.9117705055246));
#5694=CARTESIAN_POINT('Ctrl Pts',(6.19416725357822,-8.87991129560537,0.913854076356023));
#5695=CARTESIAN_POINT('Ctrl Pts',(6.32063653637879,-8.33790454041667,-1.91395420617355));
#5696=CARTESIAN_POINT('Ctrl Pts',(6.44710581917937,-5.67279303335752,-3.00365676208316));
#5697=CARTESIAN_POINT('Ctrl Pts',(6.55132367697694,-3.72145370847857,-1.65386257482374));
#5698=CARTESIAN_POINT('Ctrl Pts',(6.61338510717431,-3.44352629851068,-0.402087785484153));
#5699=CARTESIAN_POINT('Ctrl Pts',(6.6332901097715,-3.44406314725449,-0.000379914237597229));
#5700=CARTESIAN_POINT('Ctrl Pts',(5.76670989022851,-3.44347757139674,0.00126671354594932));
#5701=CARTESIAN_POINT('Ctrl Pts',(5.78366892976113,-3.44193188873403,0.343325238059439));
#5702=CARTESIAN_POINT('Ctrl Pts',(5.84278439689394,-3.66461387574044,1.53373597131417));
#5703=CARTESIAN_POINT('Ctrl Pts',(5.94405629162693,-5.4652566627727,2.97372970205115));
#5704=CARTESIAN_POINT('Ctrl Pts',(6.07052557442751,-8.19952879357467,2.0714950793584));
#5705=CARTESIAN_POINT('Ctrl Pts',(6.19699485722808,-8.9363583629794,-0.711911751364896));
#5706=CARTESIAN_POINT('Ctrl Pts',(6.32346414002865,-7.00661353387476,-2.84881518722965));
#5707=CARTESIAN_POINT('Ctrl Pts',(6.44670248436214,-4.2353929234673,-2.41014480803071));
#5708=CARTESIAN_POINT('Ctrl Pts',(6.52778440109542,-3.44082007134406,-0.778520212260661));
#5709=CARTESIAN_POINT('Ctrl Pts',(6.56670989022851,-3.43650398705703,0.00112627044576692));
#5710=CARTESIAN_POINT('Origin',(-1.7667098902285,-6.,0.));
#5711=CARTESIAN_POINT('',(4.96670989022851,-3.44096993331538,-0.00224703045531571));
#5712=CARTESIAN_POINT('',(5.0332901097715,-3.4386429978355,0.0021162044573253));
#5713=CARTESIAN_POINT('',(-1.7667098902285,-3.44,1.9679933794996E-13));
#5714=CARTESIAN_POINT('Ctrl Pts',(5.0332901097715,-3.4386429978355,0.00211620445732504));
#5715=CARTESIAN_POINT('Ctrl Pts',(5.04084130930535,-3.43729605427409,0.153691298419752));
#5716=CARTESIAN_POINT('Ctrl Pts',(5.0905489364394,-3.51832505384762,1.15003400307478));
#5717=CARTESIAN_POINT('Ctrl Pts',(5.18241299117364,-4.82454787213973,2.7834027086531));
#5718=CARTESIAN_POINT('Ctrl Pts',(5.3088822739742,-7.69028042141618,2.50439023325154));
#5719=CARTESIAN_POINT('Ctrl Pts',(5.43535155677479,-9.02103053977556,-0.0489164713765121));
#5720=CARTESIAN_POINT('Ctrl Pts',(5.56182083957535,-7.60831351323712,-2.55780100605334));
#5721=CARTESIAN_POINT('Ctrl Pts',(5.68829012237593,-4.73505008567186,-2.743887763315));
#5722=CARTESIAN_POINT('Ctrl Pts',(5.77877987910798,-3.50113301626044,-1.09414097539061));
#5723=CARTESIAN_POINT('Ctrl Pts',(5.82711320823984,-3.43683902736464,-0.125780691708827));
#5724=CARTESIAN_POINT('Ctrl Pts',(5.8332901097715,-3.43786500993883,-0.00188959581389444));
#5725=CARTESIAN_POINT('Ctrl Pts',(4.96670989022851,-3.44096993331538,-0.00224703045531561));
#5726=CARTESIAN_POINT('Ctrl Pts',(4.99739703082665,-3.44628149732869,0.615172962045894));
#5727=CARTESIAN_POINT('Ctrl Pts',(5.07024059902497,-3.97974614246111,2.08900564922984));
#5728=CARTESIAN_POINT('Ctrl Pts',(5.1852405948235,-6.43818709990916,2.98948337393659));
#5729=CARTESIAN_POINT('Ctrl Pts',(5.31170987762407,-8.74388782855944,1.26494994440632));
#5730=CARTESIAN_POINT('Ctrl Pts',(5.43817916042464,-8.55780106687306,-1.60831355147971));
#5731=CARTESIAN_POINT('Ctrl Pts',(5.56464844322523,-6.04891647253973,-3.02103061160996));
#5732=CARTESIAN_POINT('Ctrl Pts',(5.67415868649316,-3.83799822568673,-1.86872888720316));
#5733=CARTESIAN_POINT('Ctrl Pts',(5.74151250216093,-3.44577411453568,-0.50695672489885));
#5734=CARTESIAN_POINT('Ctrl Pts',(5.76670989022851,-3.44347757139674,0.00126671354594932));
#5735=CARTESIAN_POINT('Origin',(-1.7667098902285,-6.,0.));
#5736=CARTESIAN_POINT('',(4.16670989022851,-3.43619743813536,0.000808262677862992));
#5737=CARTESIAN_POINT('',(4.2332901097715,-3.44411439821716,-6.54012234668632E-5));
#5738=CARTESIAN_POINT('',(-1.7667098902285,-3.44,1.9679933794996E-13));
#5739=CARTESIAN_POINT('Ctrl Pts',(4.2332901097715,-3.44411439821716,-6.54012234668419E-5));
#5740=CARTESIAN_POINT('Ctrl Pts',(4.25456941037087,-3.4442130833179,0.429399038434416));
#5741=CARTESIAN_POINT('Ctrl Pts',(4.31800513857044,-3.74989810283886,1.70980757434144));
#5742=CARTESIAN_POINT('Ctrl Pts',(4.4235972943702,-5.77020937810816,3.01267565687393));
#5743=CARTESIAN_POINT('Ctrl Pts',(4.55006657717077,-8.39864413395782,1.83726009646369));
#5744=CARTESIAN_POINT('Ctrl Pts',(4.67653585997135,-8.84881511949022,-1.00661350993934));
#5745=CARTESIAN_POINT('Ctrl Pts',(4.80300514277192,-6.71191173443704,-2.93635829315832));
#5746=CARTESIAN_POINT('Ctrl Pts',(4.92192322603864,-4.09469599587263,-2.24352319467422));
#5747=CARTESIAN_POINT('Ctrl Pts',(4.99868488170516,-3.44481569780537,-0.692513923144139));
#5748=CARTESIAN_POINT('Ctrl Pts',(5.0332901097715,-3.4386429978355,0.00211620445732504));
#5749=CARTESIAN_POINT('Ctrl Pts',(4.16670989022851,-3.43619743813536,0.000808262677863087));
#5750=CARTESIAN_POINT('Ctrl Pts',(4.16896870429198,-3.43600925430327,0.0460361235042767));
#5751=CARTESIAN_POINT('Ctrl Pts',(4.21338394595564,-3.45752296120616,0.935172543509394));
#5752=CARTESIAN_POINT('Ctrl Pts',(4.29995561521949,-4.48748661387422,2.61559210015096));
#5753=CARTESIAN_POINT('Ctrl Pts',(4.42642489802005,-7.36566973169923,2.69517438424447));
#5754=CARTESIAN_POINT('Ctrl Pts',(4.55289418082063,-9.00365683350444,0.327206974422883));
#5755=CARTESIAN_POINT('Ctrl Pts',(4.67936346362121,-7.9139542516838,-2.33790459600758));
#5756=CARTESIAN_POINT('Ctrl Pts',(4.80583274642177,-5.08614590191431,-2.87991136408426));
#5757=CARTESIAN_POINT('Ctrl Pts',(4.90161488862421,-3.57301389199172,-1.30968210485211));
#5758=CARTESIAN_POINT('Ctrl Pts',(4.95524060322646,-3.43898474176898,-0.233007112912495));
#5759=CARTESIAN_POINT('Ctrl Pts',(4.96670989022851,-3.44096993331538,-0.00224703045531561));
#5760=CARTESIAN_POINT('Origin',(-1.7667098902285,-6.,0.));
#5761=CARTESIAN_POINT('',(3.36670989022851,-3.44315176552051,0.0015188218181697));
#5762=CARTESIAN_POINT('',(3.4332901097715,-3.43840959360912,-0.00205930223877143));
#5763=CARTESIAN_POINT('',(-1.7667098902285,-3.44,1.9679933794996E-13));
#5764=CARTESIAN_POINT('Ctrl Pts',(3.4332901097715,-3.43840959360912,-0.00205930223877139));
#5765=CARTESIAN_POINT('Ctrl Pts',(3.46829751143639,-3.44455735196194,0.700477811498659));
#5766=CARTESIAN_POINT('Ctrl Pts',(3.54546134070148,-4.10716776075693,2.25921769609112));
#5767=CARTESIAN_POINT('Ctrl Pts',(3.66478159756677,-6.73970426360059,2.92948049079009));
#5768=CARTESIAN_POINT('Ctrl Pts',(3.79125088036733,-8.85822573557158,0.979573370365098));
#5769=CARTESIAN_POINT('Ctrl Pts',(3.91772016316791,-8.3811268405867,-1.85990680208812));
#5770=CARTESIAN_POINT('Ctrl Pts',(4.04418944596848,-5.74167203129455,-3.01036293559842));
#5771=CARTESIAN_POINT('Ctrl Pts',(4.14937942816968,-3.74144472779083,-1.69344416525101));
#5772=CARTESIAN_POINT('Ctrl Pts',(4.21241298277068,-3.44401757824078,-0.421413067571763));
#5773=CARTESIAN_POINT('Ctrl Pts',(4.2332901097715,-3.44411439821716,-6.54012234668419E-5));
#5774=CARTESIAN_POINT('Ctrl Pts',(3.36670989022851,-3.44315176552051,0.00151882181816984));
#5775=CARTESIAN_POINT('Ctrl Pts',(3.3826968053575,-3.44139097769529,0.323866832040517));
#5776=CARTESIAN_POINT('Ctrl Pts',(3.44084014808668,-3.64706263387512,1.49406094909534));
#5777=CARTESIAN_POINT('Ctrl Pts',(3.54113991841605,-5.39728918769256,2.96070235836602));
#5778=CARTESIAN_POINT('Ctrl Pts',(3.66760920121662,-8.15150809295624,2.12132781612021));
#5779=CARTESIAN_POINT('Ctrl Pts',(3.79407848401719,-8.95189313670652,-0.644473185577155));
#5780=CARTESIAN_POINT('Ctrl Pts',(3.92054776681777,-7.07159629755764,-2.82501330133343));
#5781=CARTESIAN_POINT('Ctrl Pts',(4.04475823555487,-4.26912231760636,-2.44696890310363));
#5782=CARTESIAN_POINT('Ctrl Pts',(4.12681227669178,-3.43952134421862,-0.798055061899725));
#5783=CARTESIAN_POINT('Ctrl Pts',(4.16670989022851,-3.43619743813536,0.000808262677863087));
#5784=CARTESIAN_POINT('Origin',(-1.7667098902285,-6.,0.));
#5785=CARTESIAN_POINT('',(2.5667098902285,-3.44151252959564,-0.00216282566888451));
#5786=CARTESIAN_POINT('',(2.6332901097715,-3.43808642759416,0.00196523244380428));
#5787=CARTESIAN_POINT('',(-1.7667098902285,-3.44,1.9679933794996E-13));
#5788=CARTESIAN_POINT('Ctrl Pts',(2.6332901097715,-3.43808642759416,0.00196523244380487));
#5789=CARTESIAN_POINT('Ctrl Pts',(2.63986918490172,-3.43696448982562,0.133952481122952));
#5790=CARTESIAN_POINT('Ctrl Pts',(2.68860468763214,-3.50605985805332,1.11049088646622));
#5791=CARTESIAN_POINT('Ctrl Pts',(2.77949661796275,-4.7611075477298,2.75575104615122));
#5792=CARTESIAN_POINT('Ctrl Pts',(2.90596590076332,-7.63247864459777,2.54244603125873));
#5793=CARTESIAN_POINT('Ctrl Pts',(3.03243518356389,-9.02135843007676,0.0202874415191203));
#5794=CARTESIAN_POINT('Ctrl Pts',(3.15890446636447,-7.66647330603156,-2.52029463810126));
#5795=CARTESIAN_POINT('Ctrl Pts',(3.28537374916504,-4.79822553871722,-2.77213933419203));
#5796=CARTESIAN_POINT('Ctrl Pts',(3.37683563030072,-3.5131894475665,-1.13367101628351));
#5797=CARTESIAN_POINT('Ctrl Pts',(3.4261410838362,-3.43715413099785,-0.145527706283506));
#5798=CARTESIAN_POINT('Ctrl Pts',(3.4332901097715,-3.43840959360912,-0.00205930223877139));
#5799=CARTESIAN_POINT('Ctrl Pts',(2.5667098902285,-3.44151252959564,-0.0021628256688843));
#5800=CARTESIAN_POINT('Ctrl Pts',(2.59642490642301,-3.44638181709016,0.596020219394989));
#5801=CARTESIAN_POINT('Ctrl Pts',(2.66829635021772,-3.95303333681341,2.05027345959037));
#5802=CARTESIAN_POINT('Ctrl Pts',(2.7823242216126,-6.36960360330106,2.99873506265578));
#5803=CARTESIAN_POINT('Ctrl Pts',(2.90879350441318,-8.71419675286107,1.32746177559001));
#5804=CARTESIAN_POINT('Ctrl Pts',(3.03526278721375,-8.59396555469508,-1.5493099986334));
#5805=CARTESIAN_POINT('Ctrl Pts',(3.16173207001433,-6.1180947250836,-3.01911782098221));
#5806=CARTESIAN_POINT('Ctrl Pts',(3.27221443768591,-3.8615096110079,-1.907978510426));
#5807=CARTESIAN_POINT('Ctrl Pts',(3.34054037775731,-3.44603405760624,-0.526143344742301));
#5808=CARTESIAN_POINT('Ctrl Pts',(3.36670989022851,-3.44315176552051,0.00151882181816984));
#5809=CARTESIAN_POINT('Origin',(-1.7667098902285,-6.,0.));
#5810=CARTESIAN_POINT('',(1.76670989022851,-3.43598587725866,0.000468657341183842));
#5811=CARTESIAN_POINT('',(1.8332901097715,-3.44409311993689,0.000250277236630306));
#5812=CARTESIAN_POINT('',(-1.7667098902285,-3.44,1.9679933794996E-13));
#5813=CARTESIAN_POINT('Ctrl Pts',(1.8332901097715,-3.44409311993689,0.000250277236630361));
#5814=CARTESIAN_POINT('Ctrl Pts',(1.85359728596724,-3.44373249577201,0.410086549461726));
#5815=CARTESIAN_POINT('Ctrl Pts',(1.91606088976318,-3.72964858803878,1.67024234614915));
#5816=CARTESIAN_POINT('Ctrl Pts',(2.02068092115931,-5.70126992189332,3.00662240928013));
#5817=CARTESIAN_POINT('Ctrl Pts',(2.14715020395988,-8.35593592155457,1.89171467455323));
#5818=CARTESIAN_POINT('Ctrl Pts',(2.27361948676046,-8.87112245100439,-0.941102672625564));
#5819=CARTESIAN_POINT('Ctrl Pts',(2.40008876956103,-6.77897681420636,-2.91928303105917));
#5820=CARTESIAN_POINT('Ctrl Pts',(2.51997897723137,-4.12506033817286,-2.28139989219694));
#5821=CARTESIAN_POINT('Ctrl Pts',(2.59771275730153,-3.44415347724027,-0.711775950754531));
#5822=CARTESIAN_POINT('Ctrl Pts',(2.6332901097715,-3.43808642759416,0.00196523244380487));
#5823=CARTESIAN_POINT('Ctrl Pts',(1.76670989022851,-3.43598587725866,0.000468657341183452));
#5824=CARTESIAN_POINT('Ctrl Pts',(1.76799657988834,-3.43592048441881,0.0262261539081465));
#5825=CARTESIAN_POINT('Ctrl Pts',(1.81143969714838,-3.44790166097614,0.895826481676196));
#5826=CARTESIAN_POINT('Ctrl Pts',(1.8970392420086,-4.42797832080538,2.58026432327149));
#5827=CARTESIAN_POINT('Ctrl Pts',(2.02350852480917,-7.30358342959944,2.725745728157));
#5828=CARTESIAN_POINT('Ctrl Pts',(2.14997780760974,-8.99537493549262,0.395914211910863));
#5829=CARTESIAN_POINT('Ctrl Pts',(2.27644709041031,-7.9669975211319,-2.29345572403429));
#5830=CARTESIAN_POINT('Ctrl Pts',(2.40291637321089,-5.15234464286247,-2.90008608592962));
#5831=CARTESIAN_POINT('Ctrl Pts',(2.49967063981695,-3.58792809894497,-1.34934329362133));
#5832=CARTESIAN_POINT('Ctrl Pts',(2.55426847882282,-3.43947380248962,-0.2526167143973));
#5833=CARTESIAN_POINT('Ctrl Pts',(2.5667098902285,-3.44151252959564,-0.0021628256688843));
#5834=CARTESIAN_POINT('Origin',(-1.7667098902285,-6.,0.));
#5835=CARTESIAN_POINT('',(0.966709890228505,-3.4427709916825,0.00173622513077953));
#5836=CARTESIAN_POINT('',(1.0332901097715,-3.438979209753,-0.0021867409662462));
#5837=CARTESIAN_POINT('',(-1.7667098902285,-3.44,1.9679933794996E-13));
#5838=CARTESIAN_POINT('Ctrl Pts',(1.0332901097715,-3.438979209753,-0.00218674096624601));
#5839=CARTESIAN_POINT('Ctrl Pts',(1.06732538703276,-3.44514488069256,0.681234816892835));
#5840=CARTESIAN_POINT('Ctrl Pts',(1.14351709189422,-4.07723850978797,2.22122910905365));
#5841=CARTESIAN_POINT('Ctrl Pts',(1.26186522435587,-6.67241573405984,2.94565054354541));
#5842=CARTESIAN_POINT('Ctrl Pts',(1.38833450715645,-8.83504078941567,1.04478035722949));
#5843=CARTESIAN_POINT('Ctrl Pts',(1.51480378995702,-8.42309989372086,-1.8048844843804));
#5844=CARTESIAN_POINT('Ctrl Pts',(1.64127307275759,-5.81068658220031,-3.01548936826444));
#5845=CARTESIAN_POINT('Ctrl Pts',(1.74743517936242,-3.76206314555082,-1.73298420137006));
#5846=CARTESIAN_POINT('Ctrl Pts',(1.81144085836705,-3.44448112898182,-0.440707917058323));
#5847=CARTESIAN_POINT('Ctrl Pts',(1.8332901097715,-3.44409311993689,0.000250277236630361));
#5848=CARTESIAN_POINT('Ctrl Pts',(0.966709890228505,-3.4427709916825,0.00173622513077922));
#5849=CARTESIAN_POINT('Ctrl Pts',(0.981724680953865,-3.44085207515589,0.304374748864834));
#5850=CARTESIAN_POINT('Ctrl Pts',(1.03889589927942,-3.63008029168738,1.45440282564708));
#5851=CARTESIAN_POINT('Ctrl Pts',(1.13822354520516,-5.32964905792872,2.94610338914275));
#5852=CARTESIAN_POINT('Ctrl Pts',(1.26469282800573,-8.10235283801081,2.17005725520049));
#5853=CARTESIAN_POINT('Ctrl Pts',(1.3911621108063,-8.96588232345381,-0.576701529052951));
#5854=CARTESIAN_POINT('Ctrl Pts',(1.51763139360688,-7.13601528805713,-2.7997267301126));
#5855=CARTESIAN_POINT('Ctrl Pts',(1.64281398674761,-4.30362504627695,-2.48351527668098));
#5856=CARTESIAN_POINT('Ctrl Pts',(1.72584015228815,-3.43806298124983,-0.817679002928948));
#5857=CARTESIAN_POINT('Ctrl Pts',(1.76670989022851,-3.43598587725866,0.000468657341183452));
#5858=CARTESIAN_POINT('Origin',(-1.7667098902285,-6.,0.));
#5859=CARTESIAN_POINT('',(0.166709890228505,-3.44261795854501,-0.003041210415346));
#5860=CARTESIAN_POINT('',(0.233290109771496,-3.4375580541705,0.00169662369046232));
#5861=CARTESIAN_POINT('',(-1.7667098902285,-3.44,1.9679933794996E-13));
#5862=CARTESIAN_POINT('',(0.,-5.33826273143149,-2.47299490241842));
#5863=CARTESIAN_POINT('Ctrl Pts',(0.,-5.33826273143149,-2.47299490241842));
#5864=CARTESIAN_POINT('Ctrl Pts',(0.042156427600191,-4.51946448572409,-2.25389646671472));
#5865=CARTESIAN_POINT('Ctrl Pts',(0.0977263910096926,-3.60391090134556,
-1.38973602151771));
#5866=CARTESIAN_POINT('Ctrl Pts',(0.153296354419194,-3.44063791734118,-0.273280262488538));
#5867=CARTESIAN_POINT('Ctrl Pts',(0.166709890228505,-3.44261795854501,-0.00304121041534603));
#5868=CARTESIAN_POINT('',(1.04028532515104E-16,-6.66309219466394,-2.47735541001815));
#5869=CARTESIAN_POINT('Origin',(0.,-6.,0.));
#5870=CARTESIAN_POINT('Ctrl Pts',(-4.13352078260099E-17,-6.66309273064559,
-2.4773571349477));
#5871=CARTESIAN_POINT('Ctrl Pts',(0.0412138930502382,-5.86569025594692,
-2.68954112476757));
#5872=CARTESIAN_POINT('Ctrl Pts',(0.11897726297407,-4.14769481245353,-2.29913676584276));
#5873=CARTESIAN_POINT('Ctrl Pts',(0.196740632897902,-3.44336669350132,-0.730968858270161));
#5874=CARTESIAN_POINT('Ctrl Pts',(0.233290109771496,-3.4375580541705,0.00169662369046196));
#5875=CARTESIAN_POINT('Origin',(6.,6.,0.));
#5876=CARTESIAN_POINT('',(10.0890562790225,8.11715687076559,0.00188038179815303));
#5877=CARTESIAN_POINT('',(10.3109437209775,8.11380015351683,0.000572561662963434));
#5878=CARTESIAN_POINT('',(6.,8.117,2.59257727379495E-16));
#5879=CARTESIAN_POINT('',(11.,7.36291222925732,-1.61992569438875));
#5880=CARTESIAN_POINT('Ctrl Pts',(10.3109437209775,8.11380015351683,0.000572561662963434));
#5881=CARTESIAN_POINT('Ctrl Pts',(10.3298470093174,8.11459727114496,0.316007738993721));
#5882=CARTESIAN_POINT('Ctrl Pts',(10.3487502976573,8.04842739124356,0.631134507362876));
#5883=CARTESIAN_POINT('Ctrl Pts',(10.3676535859971,7.91360200006723,0.913504858331154));
#5884=CARTESIAN_POINT('Ctrl Pts',(10.4098100135973,7.61292643824968,1.54322202938665));
#5885=CARTESIAN_POINT('Ctrl Pts',(10.4519664411975,6.97079995430339,2.01002862386259));
#5886=CARTESIAN_POINT('Ctrl Pts',(10.4941228687977,6.27919611550385,2.10193932389814));
#5887=CARTESIAN_POINT('Ctrl Pts',(10.5362792963979,5.58759227670429,2.19385002393369));
#5888=CARTESIAN_POINT('Ctrl Pts',(10.5784357239981,4.84651108305146,1.91086482952882));
#5889=CARTESIAN_POINT('Ctrl Pts',(10.6205921515983,4.39166122021261,1.38152854464845));
#5890=CARTESIAN_POINT('Ctrl Pts',(10.6627485791985,3.93681135737378,0.852192259768091));
#5891=CARTESIAN_POINT('Ctrl Pts',(10.7049050067987,3.7681928253489,0.07650488441227));
#5892=CARTESIAN_POINT('Ctrl Pts',(10.7470614343988,3.96392499548221,-0.593437324111172));
#5893=CARTESIAN_POINT('Ctrl Pts',(10.789217861999,4.15965716561551,-1.26337953263462));
#5894=CARTESIAN_POINT('Ctrl Pts',(10.8313742895992,4.71974003790703,-1.82757657432568));
#5895=CARTESIAN_POINT('Ctrl Pts',(10.8735307171994,5.38646615209559,-2.02952674625186));
#5896=CARTESIAN_POINT('Ctrl Pts',(10.9156871447996,6.05319226628417,-2.23147691817804));
#5897=CARTESIAN_POINT('Ctrl Pts',(10.9578435723998,6.8265616223698,-2.07118022033934));
#5898=CARTESIAN_POINT('Ctrl Pts',(11.,7.36291222925732,-1.61992569438875));
#5899=CARTESIAN_POINT('',(11.,7.36522651177467,1.62290944688048));
#5900=CARTESIAN_POINT('Origin',(11.,6.,0.));
#5901=CARTESIAN_POINT('',(10.8890562790225,8.11943734836568,-0.00125295574427895));
#5902=CARTESIAN_POINT('Ctrl Pts',(11.,7.36522742428751,1.6229106233628));
#5903=CARTESIAN_POINT('Ctrl Pts',(10.9630187596742,7.83319589372452,1.22807491081379));
#5904=CARTESIAN_POINT('Ctrl Pts',(10.9260375193483,8.11557054190741,0.611672144507363));
#5905=CARTESIAN_POINT('Ctrl Pts',(10.8890562790225,8.11943734836568,-0.00125295574427895));
#5906=CARTESIAN_POINT('',(12.,8.117,-2.59257727379495E-16));
#5907=CARTESIAN_POINT('',(6.,8.117,2.59257727379495E-16));
#5908=CARTESIAN_POINT('Origin',(12.,6.,0.));
#5909=CARTESIAN_POINT('Ctrl Pts',(10.8890562790225,8.11943734836568,-0.00125295574427895));
#5910=CARTESIAN_POINT('Ctrl Pts',(10.8848236262981,8.11987992002488,-0.071404715733393));
#5911=CARTESIAN_POINT('Ctrl Pts',(10.8805909735737,8.11667411428522,-0.14151091923779));
#5912=CARTESIAN_POINT('Ctrl Pts',(10.8763583208493,8.10968062356725,-0.211234152861468));
#5913=CARTESIAN_POINT('Ctrl Pts',(10.8342018932491,8.04002676715129,-0.905664488088106));
#5914=CARTESIAN_POINT('Ctrl Pts',(10.7920454656489,7.59464264590244,-1.56210502861697));
#5915=CARTESIAN_POINT('Ctrl Pts',(10.7498890380487,6.97508320827158,-1.88289980549192));
#5916=CARTESIAN_POINT('Ctrl Pts',(10.7077326104485,6.35552377064071,-2.20369458236686));
#5917=CARTESIAN_POINT('Ctrl Pts',(10.6655761828483,5.56178901662783,-2.18884359558788));
#5918=CARTESIAN_POINT('Ctrl Pts',(10.6234197552481,4.95463419811742,-1.84487767155484));
#5919=CARTESIAN_POINT('Ctrl Pts',(10.5812633276479,4.34747937960703,-1.50091174752182));
#5920=CARTESIAN_POINT('Ctrl Pts',(10.5391069000478,3.9269044965991,-0.827830886234752));
#5921=CARTESIAN_POINT('Ctrl Pts',(10.4969504724476,3.88369336722059,-0.131366067674812));
#5922=CARTESIAN_POINT('Ctrl Pts',(10.4547940448474,3.84048223784208,0.565098750885158));
#5923=CARTESIAN_POINT('Ctrl Pts',(10.4126376172472,4.17463486209302,1.28494752671801));
#5924=CARTESIAN_POINT('Ctrl Pts',(10.370481189647,4.73452101011657,1.70138259696357));
#5925=CARTESIAN_POINT('Ctrl Pts',(10.3283247620468,5.2944071581401,2.11781766720914));
#5926=CARTESIAN_POINT('Ctrl Pts',(10.2861683344466,6.08002682993622,2.23083903186743));
#5927=CARTESIAN_POINT('Ctrl Pts',(10.2440119068464,6.7346104515374,1.98909777508149));
#5928=CARTESIAN_POINT('Ctrl Pts',(10.2018554792462,7.38919407313857,1.74735651829556));
#5929=CARTESIAN_POINT('Ctrl Pts',(10.159699051646,7.9127416445448,1.15085264006539));
#5930=CARTESIAN_POINT('Ctrl Pts',(10.1175426240458,8.06755648403457,0.470451384772961));
#5931=CARTESIAN_POINT('Ctrl Pts',(10.1080471757047,8.10242747274249,0.317195633784494));
#5932=CARTESIAN_POINT('Ctrl Pts',(10.0985517273636,8.11859099220767,0.159683391670918));
#5933=CARTESIAN_POINT('Ctrl Pts',(10.0890562790225,8.11715687076559,0.00188038179815303));
#5934=CARTESIAN_POINT('Origin',(6.,6.,0.));
#5935=CARTESIAN_POINT('',(9.28905627902251,8.11374159717219,-0.000568483884271914));
#5936=CARTESIAN_POINT('',(9.5109437209775,8.11714715018758,-0.00188412167347644));
#5937=CARTESIAN_POINT('',(6.,8.117,2.59257727379495E-16));
#5938=CARTESIAN_POINT('Ctrl Pts',(9.5109437209775,8.11714715018758,-0.00188412167347644));
#5939=CARTESIAN_POINT('Ctrl Pts',(9.5435751103829,8.11222033535175,0.540420570882553));
#5940=CARTESIAN_POINT('Ctrl Pts',(9.5762064997883,7.89950915526723,1.08616073405186));
#5941=CARTESIAN_POINT('Ctrl Pts',(9.6088378891937,7.5239486527264,1.47435339986777));
#5942=CARTESIAN_POINT('Ctrl Pts',(9.65099431679389,7.03876278037019,1.97585873903933));
#5943=CARTESIAN_POINT('Ctrl Pts',(9.69315074439408,6.28178130531125,2.21441722432417));
#5944=CARTESIAN_POINT('Ctrl Pts',(9.73530717199427,5.59672863575656,2.08170810641676));
#5945=CARTESIAN_POINT('Ctrl Pts',(9.77746359959447,4.91167596620186,1.94899898850936));
#5946=CARTESIAN_POINT('Ctrl Pts',(9.81962002719466,4.29855210215141,1.44502226740969));
#5947=CARTESIAN_POINT('Ctrl Pts',(9.86177645479485,4.03573710510172,0.798615374023543));
#5948=CARTESIAN_POINT('Ctrl Pts',(9.90393288239503,3.77292210805203,0.152208480637401));
#5949=CARTESIAN_POINT('Ctrl Pts',(9.94608930999522,3.86041597800307,-0.636628585035204));
#5950=CARTESIAN_POINT('Ctrl Pts',(9.98824573759542,4.25852148728445,-1.20971725556392));
#5951=CARTESIAN_POINT('Ctrl Pts',(10.0304021651956,4.65662699656582,-1.78280592609263));
#5952=CARTESIAN_POINT('Ctrl Pts',(10.0725585927958,5.36534414517754,-2.14014620147742));
#5953=CARTESIAN_POINT('Ctrl Pts',(10.114715020396,6.06281364406225,-2.11947989435853));
#5954=CARTESIAN_POINT('Ctrl Pts',(10.1568714479962,6.76028314294696,-2.09881358723964));
#5955=CARTESIAN_POINT('Ctrl Pts',(10.1990278755964,7.44650499210468,-1.70014069761706));
#5956=CARTESIAN_POINT('Ctrl Pts',(10.2411843031966,7.81000359683914,-1.10449037898824));
#5957=CARTESIAN_POINT('Ctrl Pts',(10.2644374424569,8.0105064420276,-0.775934554930158));
#5958=CARTESIAN_POINT('Ctrl Pts',(10.2876905817172,8.11281961050863,-0.387447658639123));
#5959=CARTESIAN_POINT('Ctrl Pts',(10.3109437209775,8.11380015351683,0.000572561662963434));
#5960=CARTESIAN_POINT('Ctrl Pts',(10.0890562790225,8.11715687076559,0.00188038179815303));
#5961=CARTESIAN_POINT('Ctrl Pts',(10.0563952997634,8.11222400093238,-0.540906082550074));
#5962=CARTESIAN_POINT('Ctrl Pts',(10.0237343205044,7.8990905658408,-1.08713266777252));
#5963=CARTESIAN_POINT('Ctrl Pts',(9.99107334124528,7.5229210427651,-1.4754142144647));
#5964=CARTESIAN_POINT('Ctrl Pts',(9.94891691364509,7.03738865443255,-1.97657992605523));
#5965=CARTESIAN_POINT('Ctrl Pts',(9.90676048604489,6.28024177019415,-2.21461271688159));
#5966=CARTESIAN_POINT('Ctrl Pts',(9.8646040584447,5.59527874399254,-2.08142674968445));
#5967=CARTESIAN_POINT('Ctrl Pts',(9.82244763084451,4.91031571779093,-1.9482407824873));
#5968=CARTESIAN_POINT('Ctrl Pts',(9.78029120324432,4.29753654962611,-1.44383605726662));
#5969=CARTESIAN_POINT('Ctrl Pts',(9.73813477564413,4.03517692714596,-0.797245582009668));
#5970=CARTESIAN_POINT('Ctrl Pts',(9.69597834804394,3.77281730466582,-0.150655106752722));
#5971=CARTESIAN_POINT('Ctrl Pts',(9.65382192044375,3.86087722787033,0.638121118540479));
#5972=CARTESIAN_POINT('Ctrl Pts',(9.61166549284355,4.25937402385499,1.21093137919616));
#5973=CARTESIAN_POINT('Ctrl Pts',(9.56950906524336,4.65787081983965,1.78374163985182));
#5974=CARTESIAN_POINT('Ctrl Pts',(9.52735263764317,5.36680448860446,2.14058593586996));
#5975=CARTESIAN_POINT('Ctrl Pts',(9.48519621004299,6.06427454878569,2.11943440510194));
#5976=CARTESIAN_POINT('Ctrl Pts',(9.44303978244279,6.76174460896693,2.09828287433392));
#5977=CARTESIAN_POINT('Ctrl Pts',(9.4008833548426,7.44775106056461,1.69913551677972));
#5978=CARTESIAN_POINT('Ctrl Pts',(9.35872692724241,7.81080533581827,1.10323009083302));
#5979=CARTESIAN_POINT('Ctrl Pts',(9.33550337783578,8.01080826250376,0.774951821326824));
#5980=CARTESIAN_POINT('Ctrl Pts',(9.31227982842914,8.11280177200639,0.386961479812062));
#5981=CARTESIAN_POINT('Ctrl Pts',(9.28905627902251,8.11374159717219,-0.000568483884271914));
#5982=CARTESIAN_POINT('Origin',(6.,6.,0.));
#5983=CARTESIAN_POINT('',(8.4890562790225,8.1191842221883,-0.0013863833942596));
#5984=CARTESIAN_POINT('',(8.7109437209775,8.11957111380812,0.00117038083020428));
#5985=CARTESIAN_POINT('',(6.,8.117,2.59257727379495E-16));
#5986=CARTESIAN_POINT('Ctrl Pts',(8.7109437209775,8.11957111380812,0.00117038083020428));
#5987=CARTESIAN_POINT('Ctrl Pts',(8.71514678384822,8.12003578657627,0.0708143820557132));
#5988=CARTESIAN_POINT('Ctrl Pts',(8.71934984671895,8.11689802002172,0.140416012359908));
#5989=CARTESIAN_POINT('Ctrl Pts',(8.72355290958968,8.1100195150437,0.209645972704743));
#5990=CARTESIAN_POINT('Ctrl Pts',(8.76570933718987,8.04102858961091,0.904017648980825));
#5991=CARTESIAN_POINT('Ctrl Pts',(8.80786576479007,7.59572124303596,1.56099951257333));
#5992=CARTESIAN_POINT('Ctrl Pts',(8.85002219239026,6.9762942964785,1.88228141737542));
#5993=CARTESIAN_POINT('Ctrl Pts',(8.89217861999045,6.35686734992103,2.2035633221775));
#5994=CARTESIAN_POINT('Ctrl Pts',(8.93433504759064,5.56332080338105,2.18914526818917));
#5995=CARTESIAN_POINT('Ctrl Pts',(8.97649147519083,4.95597373781604,1.84557392740617));
#5996=CARTESIAN_POINT('Ctrl Pts',(9.01864790279102,4.34862667225104,1.50200258662317));
#5997=CARTESIAN_POINT('Ctrl Pts',(9.06080433039121,3.92747908766101,0.829277959045507));
#5998=CARTESIAN_POINT('Ctrl Pts',(9.1029607579914,3.88375755383572,0.132858399714689));
#5999=CARTESIAN_POINT('Ctrl Pts',(9.14511718559159,3.84003602001042,-0.563561159616129));
#6000=CARTESIAN_POINT('Ctrl Pts',(9.18727361319178,4.17374053694986,-1.2836756507001));
#6001=CARTESIAN_POINT('Ctrl Pts',(9.22943004079197,4.73334935747058,-1.70050886767758));
#6002=CARTESIAN_POINT('Ctrl Pts',(9.27158646839217,5.2929581779913,-2.11734208465505));
#6003=CARTESIAN_POINT('Ctrl Pts',(9.31374289599236,6.07847130209331,-2.23089402752604));
#6004=CARTESIAN_POINT('Ctrl Pts',(9.35589932359255,6.73321630384336,-1.98960505813209));
#6005=CARTESIAN_POINT('Ctrl Pts',(9.39805575119274,7.3879613055934,-1.74831608873814));
#6006=CARTESIAN_POINT('Ctrl Pts',(9.44021217879293,7.9119381849915,-1.15218620707927));
#6007=CARTESIAN_POINT('Ctrl Pts',(9.48236860639312,8.06723148986381,-0.471895169720698));
#6008=CARTESIAN_POINT('Ctrl Pts',(9.49189364458791,8.10231925096,-0.318186744142753));
#6009=CARTESIAN_POINT('Ctrl Pts',(9.50141868278271,8.11858527771892,-0.160181791614469));
#6010=CARTESIAN_POINT('Ctrl Pts',(9.5109437209775,8.11714715018758,-0.00188412167347644));
#6011=CARTESIAN_POINT('Ctrl Pts',(9.28905627902251,8.11374159717219,-0.000568483884271914));
#6012=CARTESIAN_POINT('Ctrl Pts',(9.27012340082895,8.11450778476374,-0.316500276675629));
#6013=CARTESIAN_POINT('Ctrl Pts',(9.25119052263539,8.04811125783102,-0.632126091271384));
#6014=CARTESIAN_POINT('Ctrl Pts',(9.23225764444183,7.91290253697904,-0.914842607688629));
#6015=CARTESIAN_POINT('Ctrl Pts',(9.19010121684164,7.61184336397646,-1.54434638592439));
#6016=CARTESIAN_POINT('Ctrl Pts',(9.14794478924145,6.96962291906164,-2.01069044805671));
#6017=CARTESIAN_POINT('Ctrl Pts',(9.10578836164126,6.27784890751461,-2.10212583511627));
#6018=CARTESIAN_POINT('Ctrl Pts',(9.06363193404107,5.58607489596759,-2.19356122217583));
#6019=CARTESIAN_POINT('Ctrl Pts',(9.02147550644089,4.84474731778836,-1.91008793416263));
#6020=CARTESIAN_POINT('Ctrl Pts',(8.9793190788407,4.3904743882459,-1.38042031528924));
#6021=CARTESIAN_POINT('Ctrl Pts',(8.9371626512405,3.93620145870344,-0.850752696415834));
#6022=CARTESIAN_POINT('Ctrl Pts',(8.89500622364031,3.76898317779776,-0.0748907466822245));
#6023=CARTESIAN_POINT('Ctrl Pts',(8.85284979604011,3.96474696381566,0.594876539297566));
#6024=CARTESIAN_POINT('Ctrl Pts',(8.81069336843992,4.16051074983357,1.26464382527735));
#6025=CARTESIAN_POINT('Ctrl Pts',(8.76853694083973,4.71925660277507,1.82831644750333));
#6026=CARTESIAN_POINT('Ctrl Pts',(8.72638051323954,5.38727953775154,2.02995237312644));
#6027=CARTESIAN_POINT('Ctrl Pts',(8.68422408563935,6.05530247272803,2.23158829874956));
#6028=CARTESIAN_POINT('Ctrl Pts',(8.64206765803917,6.83260248973948,2.07118752776983));
#6029=CARTESIAN_POINT('Ctrl Pts',(8.59991123043898,7.36623761004502,1.62158187684418));
#6030=CARTESIAN_POINT('Ctrl Pts',(8.56295957996682,7.83398830828272,1.22748608151556));
#6031=CARTESIAN_POINT('Ctrl Pts',(8.52600792949466,8.11452728017455,0.611189445711882));
#6032=CARTESIAN_POINT('Ctrl Pts',(8.4890562790225,8.1191842221883,-0.0013863833942596));
#6033=CARTESIAN_POINT('Origin',(6.,6.,0.));
#6034=CARTESIAN_POINT('',(7.6890562790225,8.11764522427697,0.00183633476372319));
#6035=CARTESIAN_POINT('',(7.9109437209775,8.11390728528231,0.000819409340793068));
#6036=CARTESIAN_POINT('',(6.,8.117,2.59257727379495E-16));
#6037=CARTESIAN_POINT('Ctrl Pts',(7.9109437209775,8.11390728528231,0.000819409340793068));
#6038=CARTESIAN_POINT('Ctrl Pts',(7.92887488491374,8.11495802236128,0.299977125821297));
#6039=CARTESIAN_POINT('Ctrl Pts',(7.94680604884999,8.0556605354732,0.598737210873491));
#6040=CARTESIAN_POINT('Ctrl Pts',(7.96473721278624,7.93396030919504,0.869443135120387));
#6041=CARTESIAN_POINT('Ctrl Pts',(8.00689364038643,7.64784130452458,1.50587670613843));
#6042=CARTESIAN_POINT('Ctrl Pts',(8.04905006798663,7.01680554234725,1.98724737007717));
#6043=CARTESIAN_POINT('Ctrl Pts',(8.09120649558682,6.32738204764409,2.09498325502854));
#6044=CARTESIAN_POINT('Ctrl Pts',(8.13336292318701,5.63795855294095,2.20271913997992));
#6045=CARTESIAN_POINT('Ctrl Pts',(8.1755193507872,4.89014732571198,1.93682024594394));
#6046=CARTESIAN_POINT('Ctrl Pts',(8.21767577838739,4.42350063564333,1.41802101580699));
#6047=CARTESIAN_POINT('Ctrl Pts',(8.25983220598758,3.95685394557466,0.899221785670026));
#6048=CARTESIAN_POINT('Ctrl Pts',(8.30198863358777,3.77137179266632,0.127522219432072));
#6049=CARTESIAN_POINT('Ctrl Pts',(8.34414506118796,3.95127446966703,-0.546678641855785));
#6050=CARTESIAN_POINT('Ctrl Pts',(8.38630148878815,4.13117714666773,-1.22087950314363));
#6051=CARTESIAN_POINT('Ctrl Pts',(8.42845791638834,4.67646465357747,-1.79758165948139));
#6052=CARTESIAN_POINT('Ctrl Pts',(8.47061434398854,5.33954295512743,-2.01492688192885));
#6053=CARTESIAN_POINT('Ctrl Pts',(8.51277077158873,6.00262125667738,-2.2322721043763));
#6054=CARTESIAN_POINT('Ctrl Pts',(8.55492719918893,6.78349035286756,-2.09026039293348));
#6055=CARTESIAN_POINT('Ctrl Pts',(8.59708362678912,7.32758764881733,-1.65337379273224));
#6056=CARTESIAN_POINT('Ctrl Pts',(8.63503699151858,7.81743757911368,-1.26004548132718));
#6057=CARTESIAN_POINT('Ctrl Pts',(8.67299035624804,8.11537515110373,-0.627710095390964));
#6058=CARTESIAN_POINT('Ctrl Pts',(8.7109437209775,8.11957111380812,0.00117038083020428));
#6059=CARTESIAN_POINT('Ctrl Pts',(8.4890562790225,8.1191842221883,-0.0013863833942596));
#6060=CARTESIAN_POINT('Ctrl Pts',(8.48385150189447,8.11984016975681,-0.0876699627142483));
#6061=CARTESIAN_POINT('Ctrl Pts',(8.47864672476643,8.11502268181792,-0.173879722092055));
#6062=CARTESIAN_POINT('Ctrl Pts',(8.4734419476384,8.10448396876637,-0.259384322358413));
#6063=CARTESIAN_POINT('Ctrl Pts',(8.4312855200382,8.01912498358259,-0.95193433976384));
#6064=CARTESIAN_POINT('Ctrl Pts',(8.38912909243802,7.55843678961539,-1.59822384370313));
#6065=CARTESIAN_POINT('Ctrl Pts',(8.34697266483783,6.9316001490884,-1.90479766919029));
#6066=CARTESIAN_POINT('Ctrl Pts',(8.30481623723763,6.30476350856141,-2.21137149467746));
#6067=CARTESIAN_POINT('Ctrl Pts',(8.26265980963744,5.51177842147463,-2.17822964171251));
#6068=CARTESIAN_POINT('Ctrl Pts',(8.22050338203725,4.91270886183563,-1.82042054975661));
#6069=CARTESIAN_POINT('Ctrl Pts',(8.17834695443706,4.31363930219663,-1.46261145780071));
#6070=CARTESIAN_POINT('Ctrl Pts',(8.13619052683687,3.90848527000542,-0.780135126853865));
#6071=CARTESIAN_POINT('Ctrl Pts',(8.09403409923668,3.88121160212363,-0.0828777635467605));
#6072=CARTESIAN_POINT('Ctrl Pts',(8.05187767163649,3.85393793424184,0.614379599760344));
#6073=CARTESIAN_POINT('Ctrl Pts',(8.00972124403629,4.20454463066947,1.32641799542771));
#6074=CARTESIAN_POINT('Ctrl Pts',(7.9675648164361,4.77383469847484,1.72992822147259));
#6075=CARTESIAN_POINT('Ctrl Pts',(7.92540838883591,5.3431247662802,2.13343844751747));
#6076=CARTESIAN_POINT('Ctrl Pts',(7.88325196123572,6.13109820546331,2.22842050393988));
#6077=CARTESIAN_POINT('Ctrl Pts',(7.84109553363553,6.77996663691654,1.97174669856434));
#6078=CARTESIAN_POINT('Ctrl Pts',(7.79893910603534,7.42883506836976,1.71507289318879));
#6079=CARTESIAN_POINT('Ctrl Pts',(7.75678267843515,7.93859849209309,1.1067432260153));
#6080=CARTESIAN_POINT('Ctrl Pts',(7.71462625083496,8.07779297766,0.422976760830654));
#6081=CARTESIAN_POINT('Ctrl Pts',(7.70610292689747,8.10593577244447,0.284730628221179));
#6082=CARTESIAN_POINT('Ctrl Pts',(7.69757960295999,8.11893042409154,0.143400784872793));
#6083=CARTESIAN_POINT('Ctrl Pts',(7.6890562790225,8.11764522427697,0.00183633476372319));
#6084=CARTESIAN_POINT('Origin',(6.,6.,0.));
#6085=CARTESIAN_POINT('',(6.8890562790225,8.11363988703895,-0.00031417125408606));
#6086=CARTESIAN_POINT('',(7.1109437209775,8.11666666562943,-0.00189050366901346));
#6087=CARTESIAN_POINT('',(6.,8.117,2.59257727379495E-16));
#6088=CARTESIAN_POINT('Ctrl Pts',(7.1109437209775,8.11666666562943,-0.00189050366901346));
#6089=CARTESIAN_POINT('Ctrl Pts',(7.14260298597926,8.11196924156364,0.52456406017017));
#6090=CARTESIAN_POINT('Ctrl Pts',(7.17426225098103,7.91296473303274,1.05418917756107));
#6091=CARTESIAN_POINT('Ctrl Pts',(7.2059215159828,7.55731496712391,1.43906356250341));
#6092=CARTESIAN_POINT('Ctrl Pts',(7.248077943583,7.08374353055638,1.9515495328215));
#6093=CARTESIAN_POINT('Ctrl Pts',(7.29023437118319,6.33242904651292,2.2073822840917));
#6094=CARTESIAN_POINT('Ctrl Pts',(7.33239079878338,5.64451447516916,2.09039802080721));
#6095=CARTESIAN_POINT('Ctrl Pts',(7.37454722638357,4.9565999038254,1.97341375752272));
#6096=CARTESIAN_POINT('Ctrl Pts',(7.41670365398376,4.33208524518135,1.48361247968354));
#6097=CARTESIAN_POINT('Ctrl Pts',(7.45886008158395,4.05453854420681,0.843394076261605));
#6098=CARTESIAN_POINT('Ctrl Pts',(7.50101650918415,3.77699184323228,0.203175672839669));
#6099=CARTESIAN_POINT('Ctrl Pts',(7.54317293678434,3.84641309992727,-0.58745985616502));
#6100=CARTESIAN_POINT('Ctrl Pts',(7.58532936438453,4.23128079618797,-1.16951537899457));
#6101=CARTESIAN_POINT('Ctrl Pts',(7.62748579198472,4.61614849244866,-1.75157090182411));
#6102=CARTESIAN_POINT('Ctrl Pts',(7.6696422195849,5.31646262827508,-2.12504641847851));
#6103=CARTESIAN_POINT('Ctrl Pts',(7.7117986471851,6.01423753687015,-2.12036108629895));
#6104=CARTESIAN_POINT('Ctrl Pts',(7.75395507478529,6.71201244546522,-2.1156757541194));
#6105=CARTESIAN_POINT('Ctrl Pts',(7.79611150238549,7.40724812682894,-1.73282957310589));
#6106=CARTESIAN_POINT('Ctrl Pts',(7.83826792998568,7.78426484392901,-1.14565824355045));
#6107=CARTESIAN_POINT('Ctrl Pts',(7.86249319364962,8.0009181491873,-0.808239228607084));
#6108=CARTESIAN_POINT('Ctrl Pts',(7.88671845731356,8.11248772418353,-0.403347023167936));
#6109=CARTESIAN_POINT('Ctrl Pts',(7.9109437209775,8.11390728528231,0.000819409340793068));
#6110=CARTESIAN_POINT('Ctrl Pts',(7.6890562790225,8.11764522427697,0.00183633476372319));
#6111=CARTESIAN_POINT('Ctrl Pts',(7.6554231753598,8.11257381564489,-0.55677810490725));
#6112=CARTESIAN_POINT('Ctrl Pts',(7.62179007169709,7.88515114816674,-1.11904560138433));
#6113=CARTESIAN_POINT('Ctrl Pts',(7.58815696803438,7.4887278443704,-1.5099080778379));
#6114=CARTESIAN_POINT('Ctrl Pts',(7.54600054043419,6.99184267810341,-1.99982318812603));
#6115=CARTESIAN_POINT('Ctrl Pts',(7.503844112834,6.22944679815893,-2.22045014550648));
#6116=CARTESIAN_POINT('Ctrl Pts',(7.46168768523381,5.54771479964697,-2.07161074906936));
#6117=CARTESIAN_POINT('Ctrl Pts',(7.41953125763362,4.86598280113501,-1.92277135263224));
#6118=CARTESIAN_POINT('Ctrl Pts',(7.37737483003343,4.26491468405557,-1.40446560237755));
#6119=CARTESIAN_POINT('Ctrl Pts',(7.33521840243324,4.01743232216016,-0.752036169962131));
#6120=CARTESIAN_POINT('Ctrl Pts',(7.29306197483305,3.76994996026475,-0.0996067375467069));
#6121=CARTESIAN_POINT('Ctrl Pts',(7.25090554723286,3.87605335355337,0.686946377029455));
#6122=CARTESIAN_POINT('Ctrl Pts',(7.20874911963266,4.28756503912573,1.25047970911464));
#6123=CARTESIAN_POINT('Ctrl Pts',(7.16659269203248,4.6990767246981,1.81401304119983));
#6124=CARTESIAN_POINT('Ctrl Pts',(7.12443626443228,5.41599670255422,2.15452659079405));
#6125=CARTESIAN_POINT('Ctrl Pts',(7.08227983683209,6.11279923257889,2.11740627449295));
#6126=CARTESIAN_POINT('Ctrl Pts',(7.0401234092319,6.80960176260356,2.08028595819184));
#6127=CARTESIAN_POINT('Ctrl Pts',(6.99796698163171,7.4862868447968,1.66553177599542));
#6128=CARTESIAN_POINT('Ctrl Pts',(6.95581055403152,7.8355978549684,1.06146762219652));
#6129=CARTESIAN_POINT('Ctrl Pts',(6.93355912902851,8.01997466742683,0.74262447109424));
#6130=CARTESIAN_POINT('Ctrl Pts',(6.91130770402551,8.11314360517165,0.371038718645036));
#6131=CARTESIAN_POINT('Ctrl Pts',(6.8890562790225,8.11363988703895,-0.00031417125408606));
#6132=CARTESIAN_POINT('Origin',(6.,6.,0.));
#6133=CARTESIAN_POINT('',(6.0890562790225,8.11876545586576,-0.0015626071037439));
#6134=CARTESIAN_POINT('',(6.3109437209775,8.11989110689617,0.00093137289447728));
#6135=CARTESIAN_POINT('',(6.,8.117,2.59257727379495E-16));
#6136=CARTESIAN_POINT('Ctrl Pts',(6.3109437209775,8.11989110689617,0.00093137289447728));
#6137=CARTESIAN_POINT('Ctrl Pts',(6.3141746594446,8.12018736172121,0.0544460906262127));
#6138=CARTESIAN_POINT('Ctrl Pts',(6.3174055979117,8.11833493546569,0.10793997063244));
#6139=CARTESIAN_POINT('Ctrl Pts',(6.3206365363788,8.11426759726748,0.161264909122649));
#6140=CARTESIAN_POINT('Ctrl Pts',(6.36279296397899,8.06119804796336,0.857034553651034));
#6141=CARTESIAN_POINT('Ctrl Pts',(6.40494939157917,7.63105440762909,1.52404302381293));
#6142=CARTESIAN_POINT('Ctrl Pts',(6.44710581917936,7.01914833056754,1.8594274721189));
#6143=CARTESIAN_POINT('Ctrl Pts',(6.48926224677956,6.40724225350598,2.19481192042488));
#6144=CARTESIAN_POINT('Ctrl Pts',(6.53141867437976,5.61357373971716,2.19857234687494));
#6145=CARTESIAN_POINT('Ctrl Pts',(6.57357510197995,4.9985170824839,1.86900128670161));
#6146=CARTESIAN_POINT('Ctrl Pts',(6.61573152958014,4.38346042525066,1.53943022652828));
#6147=CARTESIAN_POINT('Ctrl Pts',(6.65788795718032,3.94701562457299,0.876527679731573));
#6148=CARTESIAN_POINT('Ctrl Pts',(6.70004438478051,3.8873554488927,0.181292152195573));
#6149=CARTESIAN_POINT('Ctrl Pts',(6.7422008123807,3.82769527321242,-0.513943375340437));
#6150=CARTESIAN_POINT('Ctrl Pts',(6.78435723998089,4.14481972252953,-1.24151188361575));
#6151=CARTESIAN_POINT('Ctrl Pts',(6.82651366758109,4.69473480272403,-1.67105254511866));
#6152=CARTESIAN_POINT('Ctrl Pts',(6.86867009518128,5.24464988291853,-2.10059320662157));
#6153=CARTESIAN_POINT('Ctrl Pts',(6.91082652278147,6.02735559399041,-2.23210602135209));
#6154=CARTESIAN_POINT('Ctrl Pts',(6.95298295038166,6.68745542899508,-2.00587608712802));
#6155=CARTESIAN_POINT('Ctrl Pts',(6.99513937798185,7.34755526399976,-1.77964615290396));
#6156=CARTESIAN_POINT('Ctrl Pts',(7.03729580558204,7.88504922293722,-1.19567346972529));
#6157=CARTESIAN_POINT('Ctrl Pts',(7.07945223318223,8.05588200786014,-0.519117533452964));
#6158=CARTESIAN_POINT('Ctrl Pts',(7.08994939578065,8.09842023091556,-0.350651700974674));
#6159=CARTESIAN_POINT('Ctrl Pts',(7.10044655837908,8.11822417570459,-0.176445382216928));
#6160=CARTESIAN_POINT('Ctrl Pts',(7.1109437209775,8.11666666562943,-0.00189050366901346));
#6161=CARTESIAN_POINT('Ctrl Pts',(6.8890562790225,8.11363988703895,-0.00031417125408606));
#6162=CARTESIAN_POINT('Ctrl Pts',(6.86915127642532,8.11408383576835,-0.332507738044336));
#6163=CARTESIAN_POINT('Ctrl Pts',(6.84924627382813,8.04036937120591,-0.664514963814514));
#6164=CARTESIAN_POINT('Ctrl Pts',(6.82934127123095,7.8914479510022,-0.958414131147649));
#6165=CARTESIAN_POINT('Ctrl Pts',(6.78718484363076,7.57605009871439,-1.58085760529158));
#6166=CARTESIAN_POINT('Ctrl Pts',(6.74502841603057,6.92331745598877,-2.03237042817807));
#6167=CARTESIAN_POINT('Ctrl Pts',(6.70287198843038,6.22963076710099,-2.1079380230298));
#6168=CARTESIAN_POINT('Ctrl Pts',(6.66071556083018,5.5359440782132,-2.18350561788154));
#6169=CARTESIAN_POINT('Ctrl Pts',(6.61855913322999,4.80130334316326,-1.88312798469853));
#6170=CARTESIAN_POINT('Ctrl Pts',(6.5764027056298,4.35928061515932,-1.34319503362046));
#6171=CARTESIAN_POINT('Ctrl Pts',(6.53424627802961,3.91725788715539,-0.803262082542392));
#6172=CARTESIAN_POINT('Ctrl Pts',(6.49208985042942,3.76785316619748,-0.0237738135692568));
#6173=CARTESIAN_POINT('Ctrl Pts',(6.44993342282923,3.97890537973814,0.641334182842987));
#6174=CARTESIAN_POINT('Ctrl Pts',(6.40777699522904,4.18995759327881,1.30644217925523));
#6175=CARTESIAN_POINT('Ctrl Pts',(6.36562056762885,4.76146674131807,1.85716990310661));
#6176=CARTESIAN_POINT('Ctrl Pts',(6.32346414002865,5.43393253910038,2.04345311368894));
#6177=CARTESIAN_POINT('Ctrl Pts',(6.28130771242846,6.10639833688271,2.22973632427128));
#6178=CARTESIAN_POINT('Ctrl Pts',(6.23915128482827,6.87982078440811,2.05157502158459));
#6179=CARTESIAN_POINT('Ctrl Pts',(6.19699485722808,7.40301854703335,1.58986538889771));
#6180=CARTESIAN_POINT('Ctrl Pts',(6.16101533115955,7.84955561411832,1.19580700418601));
#6181=CARTESIAN_POINT('Ctrl Pts',(6.12503580509103,8.11382342309418,0.595205672810865));
#6182=CARTESIAN_POINT('Ctrl Pts',(6.0890562790225,8.11876545586576,-0.0015626071037439));
#6183=CARTESIAN_POINT('Origin',(6.,6.,0.));
#6184=CARTESIAN_POINT('',(5.2890562790225,8.11812209636794,0.00175000182231128));
#6185=CARTESIAN_POINT('',(5.51094372097749,8.11412427934883,0.00104751275875566));
#6186=CARTESIAN_POINT('',(6.,8.117,2.59257727379495E-16));
#6187=CARTESIAN_POINT('Ctrl Pts',(5.51094372097749,8.11412427934883,0.00104751275875566));
#6188=CARTESIAN_POINT('Ctrl Pts',(5.52790276051011,8.11540248649808,0.28391388762074));
#6189=CARTESIAN_POINT('Ctrl Pts',(5.54486180004273,8.06257424903286,0.566322454846834));
#6190=CARTESIAN_POINT('Ctrl Pts',(5.56182083957536,7.95336598668525,0.824921308871607));
#6191=CARTESIAN_POINT('Ctrl Pts',(5.60397726717555,7.6818983604589,1.46774095949028));
#6192=CARTESIAN_POINT('Ctrl Pts',(5.64613369477574,7.06205302422545,1.96343805423379));
#6193=CARTESIAN_POINT('Ctrl Pts',(5.68829012237593,6.37527786348045,2.08693564082625));
#6194=CARTESIAN_POINT('Ctrl Pts',(5.73044654997612,5.68850270273544,2.21043322741871));
#6195=CARTESIAN_POINT('Ctrl Pts',(5.77260297757631,4.93479771747889,1.9617313058601));
#6196=CARTESIAN_POINT('Ctrl Pts',(5.8147594051765,4.45639130242119,1.45375583662744));
#6197=CARTESIAN_POINT('Ctrl Pts',(5.85691583277669,3.9779848873635,0.94578036739478));
#6198=CARTESIAN_POINT('Ctrl Pts',(5.89907226037688,3.77487704250467,0.178531350488057));
#6199=CARTESIAN_POINT('Ctrl Pts',(5.94122868797708,3.93929121476205,-0.499612996440685));
#6200=CARTESIAN_POINT('Ctrl Pts',(5.98338511557727,4.10370538701942,-1.17775734336943));
#6201=CARTESIAN_POINT('Ctrl Pts',(6.02554154317746,4.635641576393,-1.7667970203202));
#6202=CARTESIAN_POINT('Ctrl Pts',(6.06769797077765,5.29356805397195,-1.99927180478301));
#6203=CARTESIAN_POINT('Ctrl Pts',(6.10985439837784,5.9514945315509,-2.23174658924581));
#6204=CARTESIAN_POINT('Ctrl Pts',(6.15201082597803,6.73541129733521,-2.10765648122066));
#6205=CARTESIAN_POINT('Ctrl Pts',(6.19416725357822,7.28937195109038,-1.68334601776064));
#6206=CARTESIAN_POINT('Ctrl Pts',(6.23309274271131,7.80087614239452,-1.29155541132901));
#6207=CARTESIAN_POINT('Ctrl Pts',(6.27201823184441,8.1163219073926,-0.643799743076592));
#6208=CARTESIAN_POINT('Ctrl Pts',(6.3109437209775,8.11989110689617,0.00093137289447728));
#6209=CARTESIAN_POINT('Ctrl Pts',(6.0890562790225,8.11876545586576,-0.0015626071037439));
#6210=CARTESIAN_POINT('Ctrl Pts',(6.08287937749084,8.11961389532931,-0.104014732104856));
#6211=CARTESIAN_POINT('Ctrl Pts',(6.07670247595917,8.1128191182144,-0.206353883984291));
#6212=CARTESIAN_POINT('Ctrl Pts',(6.07052557442751,8.09799122284675,-0.307515571951035));
#6213=CARTESIAN_POINT('Ctrl Pts',(6.02836914682732,7.99679305830984,-0.997928937425843));
#6214=CARTESIAN_POINT('Ctrl Pts',(5.98621271922713,7.52142365151097,-1.63349770568842));
#6215=CARTESIAN_POINT('Ctrl Pts',(5.94405629162694,6.8877299348249,-1.92563458655846));
#6216=CARTESIAN_POINT('Ctrl Pts',(5.90189986402674,6.25403621813882,-2.21777146742851));
#6217=CARTESIAN_POINT('Ctrl Pts',(5.85974343642655,5.46201819156553,-2.16647646090602));
#6218=CARTESIAN_POINT('Ctrl Pts',(5.81758700882636,4.87130072573482,-1.79504065313509));
#6219=CARTESIAN_POINT('Ctrl Pts',(5.77543058122617,4.28058325990411,-1.42360484536416));
#6220=CARTESIAN_POINT('Ctrl Pts',(5.73327415362598,3.89116635481596,-0.732028236344795));
#6221=CARTESIAN_POINT('Ctrl Pts',(5.69111772602579,3.8798692234361,-0.0343291188489477));
#6222=CARTESIAN_POINT('Ctrl Pts',(5.6489612984256,3.86857209205625,0.6633699986469));
#6223=CARTESIAN_POINT('Ctrl Pts',(5.60680487082541,4.23539473438468,1.36719162461923));
#6224=CARTESIAN_POINT('Ctrl Pts',(5.56464844322521,4.81377712165265,1.75755747587944));
#6225=CARTESIAN_POINT('Ctrl Pts',(5.52249201562502,5.39215950892061,2.14792332713965));
#6226=CARTESIAN_POINT('Ctrl Pts',(5.48033558802483,6.18210164112811,2.22483340368774));
#6227=CARTESIAN_POINT('Ctrl Pts',(5.43817916042464,6.82492123129587,1.95336580299024));
#6228=CARTESIAN_POINT('Ctrl Pts',(5.39602273282445,7.46774082146363,1.68189820229274));
#6229=CARTESIAN_POINT('Ctrl Pts',(5.35386630522426,7.96343786959165,1.06205292434967));
#6230=CARTESIAN_POINT('Ctrl Pts',(5.31170987762407,8.08693544457034,0.375277828189158));
#6231=CARTESIAN_POINT('Ctrl Pts',(5.30415867809021,8.10905674098226,0.252260388590747));
#6232=CARTESIAN_POINT('Ctrl Pts',(5.29660747855636,8.11923595551276,0.127095494664423));
#6233=CARTESIAN_POINT('Ctrl Pts',(5.2890562790225,8.11812209636794,0.00175000182231128));
#6234=CARTESIAN_POINT('Origin',(6.,6.,0.));
#6235=CARTESIAN_POINT('',(4.4890562790225,8.11359750489683,-5.40837440764219E-5));
#6236=CARTESIAN_POINT('',(4.71094372097749,8.11619797856316,-0.00185818891683977));
#6237=CARTESIAN_POINT('',(6.,8.117,2.59257727379495E-16));
#6238=CARTESIAN_POINT('Ctrl Pts',(4.71094372097749,8.11619797856316,-0.00185818891683977));
#6239=CARTESIAN_POINT('Ctrl Pts',(4.74163086157564,8.11180556396272,0.508719219713788));
#6240=CARTESIAN_POINT('Ctrl Pts',(4.77231800217378,7.92596018761809,1.02216466154014));
#6241=CARTESIAN_POINT('Ctrl Pts',(4.80300514277192,7.58986553840906,1.40301867897351));
#6242=CARTESIAN_POINT('Ctrl Pts',(4.84516157037211,7.12815586230291,1.9262164908004));
#6243=CARTESIAN_POINT('Ctrl Pts',(4.8873179979723,6.38289782953163,2.19918959419595));
#6244=CARTESIAN_POINT('Ctrl Pts',(4.92947442557249,5.69248439913017,2.09799142014236));
#6245=CARTESIAN_POINT('Ctrl Pts',(4.97163085317269,5.00207096872872,1.99679324608877));
#6246=CARTESIAN_POINT('Ctrl Pts',(5.01378728077288,4.3665021406971,1.52142379458605));
#6247=CARTESIAN_POINT('Ctrl Pts',(5.05594370837307,4.07436523235441,0.887730018307272));
#6248=CARTESIAN_POINT('Ctrl Pts',(5.09810013597325,3.78222832401172,0.254036242028489));
#6249=CARTESIAN_POINT('Ctrl Pts',(5.14025656357344,3.83352333535799,-0.537981859026349));
#6250=CARTESIAN_POINT('Ctrl Pts',(5.18241299117363,4.20495917805882,-1.12869938040828));
#6251=CARTESIAN_POINT('Ctrl Pts',(5.22456941877383,4.57639502075965,-1.71941690179022));
#6252=CARTESIAN_POINT('Ctrl Pts',(5.26672584637402,5.26797169481504,-2.10883384349925));
#6253=CARTESIAN_POINT('Ctrl Pts',(5.30888227397421,5.96567087792268,-2.12013097594151));
#6254=CARTESIAN_POINT('Ctrl Pts',(5.3510387015744,6.66337006103032,-2.13142810838377));
#6255=CARTESIAN_POINT('Ctrl Pts',(5.39319512917459,7.36719175319021,-1.76460543155926));
#6256=CARTESIAN_POINT('Ctrl Pts',(5.43535155677478,7.75755764116054,-1.18622298990009));
#6257=CARTESIAN_POINT('Ctrl Pts',(5.46054894484235,7.99088388172379,-0.8405170640524));
#6258=CARTESIAN_POINT('Ctrl Pts',(5.48574633290992,8.11222514576236,-0.419229461356099));
#6259=CARTESIAN_POINT('Ctrl Pts',(5.51094372097749,8.11412427934883,0.00104751275875566));
#6260=CARTESIAN_POINT('Ctrl Pts',(5.2890562790225,8.11812209636794,0.00175000182231128));
#6261=CARTESIAN_POINT('Ctrl Pts',(5.25445105095617,8.11301756303291,-0.572676531000783));
#6262=CARTESIAN_POINT('Ctrl Pts',(5.21984582288983,7.87074087424131,-1.15089592264707));
#6263=CARTESIAN_POINT('Ctrl Pts',(5.1852405948235,7.45375569991587,-1.54360855241751));
#6264=CARTESIAN_POINT('Ctrl Pts',(5.14308416722331,6.94578027845333,-2.02201492248574));
#6265=CARTESIAN_POINT('Ctrl Pts',(5.10092773962311,6.17853133369889,-2.22512274824425));
#6266=CARTESIAN_POINT('Ctrl Pts',(5.05877131202292,5.500387050543,-2.06070859144841));
#6267=CARTESIAN_POINT('Ctrl Pts',(5.01661488442273,4.82224276738711,-1.89629443465257));
#6268=CARTESIAN_POINT('Ctrl Pts',(4.97445845682254,4.23320314582978,-1.36435829530238));
#6269=CARTESIAN_POINT('Ctrl Pts',(4.93230202922235,4.00072838322897,-0.706431879594986));
#6270=CARTESIAN_POINT('Ctrl Pts',(4.89014560162216,3.76825362062816,-0.0485054638875976));
#6271=CARTESIAN_POINT('Ctrl Pts',(4.84798917402197,3.89234371698386,0.735411228176989));
#6272=CARTESIAN_POINT('Ctrl Pts',(4.80583274642178,4.31665414054163,1.28937182983757));
#6273=CARTESIAN_POINT('Ctrl Pts',(4.76367631882158,4.74096456409941,1.84333243149815));
#6274=CARTESIAN_POINT('Ctrl Pts',(4.7215198912214,5.46549531485925,2.16733694275472));
#6275=CARTESIAN_POINT('Ctrl Pts',(4.6793634636212,6.1612648939573,2.11426739844126));
#6276=CARTESIAN_POINT('Ctrl Pts',(4.63720703602101,6.85703447305535,2.0611978541278));
#6277=CARTESIAN_POINT('Ctrl Pts',(4.59505060842082,7.5240428804916,1.63105425424432));
#6278=CARTESIAN_POINT('Ctrl Pts',(4.55289418082063,7.85942729725793,1.01914823472655));
#6279=CARTESIAN_POINT('Ctrl Pts',(4.53161488022125,8.02871929439777,0.710276423970282));
#6280=CARTESIAN_POINT('Ctrl Pts',(4.51033557962188,8.11351589694749,0.355092863157482));
#6281=CARTESIAN_POINT('Ctrl Pts',(4.4890562790225,8.11359750489683,-5.40837440764219E-5));
#6282=CARTESIAN_POINT('Origin',(6.,6.,0.));
#6283=CARTESIAN_POINT('',(3.6890562790225,8.11831511071496,-0.001702946356694));
#6284=CARTESIAN_POINT('',(3.91094372097749,8.12014460849304,0.000668395368594085));
#6285=CARTESIAN_POINT('',(6.,8.117,2.59257727379495E-16));
#6286=CARTESIAN_POINT('Ctrl Pts',(3.91094372097749,8.12014460849304,0.000668395368594085));
#6287=CARTESIAN_POINT('Ctrl Pts',(3.91320253504096,8.12030022770606,0.0380697174170374));
#6288=CARTESIAN_POINT('Ctrl Pts',(3.91546134910444,8.1193954443398,0.0754633589122573));
#6289=CARTESIAN_POINT('Ctrl Pts',(3.91772016316791,8.11740647361435,0.112799243186508));
#6290=CARTESIAN_POINT('Ctrl Pts',(3.9598765907681,8.08028615382247,0.80960183873867));
#6291=CARTESIAN_POINT('Ctrl Pts',(4.00203301836829,7.66553193262247,1.48628698456753));
#6292=CARTESIAN_POINT('Ctrl Pts',(4.04418944596848,7.06146772201725,1.83559802758844));
#6293=CARTESIAN_POINT('Ctrl Pts',(4.08634587356867,6.45740351141202,2.18490907060935));
#6294=CARTESIAN_POINT('Ctrl Pts',(4.12850230116887,5.66402931140155,2.20684601082232));
#6295=CARTESIAN_POINT('Ctrl Pts',(4.17065872876906,5.04158577872288,1.89144812887443));
#6296=CARTESIAN_POINT('Ctrl Pts',(4.21281515636925,4.41914224604421,1.57605024692654));
#6297=CARTESIAN_POINT('Ctrl Pts',(4.25497158396943,3.96762938069734,0.923317542817797));
#6298=CARTESIAN_POINT('Ctrl Pts',(4.29712801156963,3.8920617787392,0.22963078869555));
#6299=CARTESIAN_POINT('Ctrl Pts',(4.33928443916982,3.81649417678106,-0.464055965426697));
#6300=CARTESIAN_POINT('Ctrl Pts',(4.38144086677001,4.11687183821165,-1.19869676956244));
#6301=CARTESIAN_POINT('Ctrl Pts',(4.4235972943702,4.65680484006513,-1.64071953913431));
#6302=CARTESIAN_POINT('Ctrl Pts',(4.46575372197039,5.19673784191862,-2.08274230870617));
#6303=CARTESIAN_POINT('Ctrl Pts',(4.50791014957058,5.97622618419501,-2.23214704371415));
#6304=CARTESIAN_POINT('Ctrl Pts',(4.55006657717077,6.64133424315417,-2.0210948103261));
#6305=CARTESIAN_POINT('Ctrl Pts',(4.59222300477096,7.30644230211334,-1.81004257693804));
#6306=CARTESIAN_POINT('Ctrl Pts',(4.63437943237115,7.85717007775528,-1.23853337515395));
#6307=CARTESIAN_POINT('Ctrl Pts',(4.67653585997135,8.04345330585575,-0.566067514132789));
#6308=CARTESIAN_POINT('Ctrl Pts',(4.6880051469734,8.09413444579994,-0.383113113150845));
#6309=CARTESIAN_POINT('Ctrl Pts',(4.69947443397545,8.11783963896887,-0.192685966357322));
#6310=CARTESIAN_POINT('Ctrl Pts',(4.71094372097749,8.11619797856316,-0.00185818891683977));
#6311=CARTESIAN_POINT('Ctrl Pts',(4.4890562790225,8.11359750489683,-5.40837440764219E-5));
#6312=CARTESIAN_POINT('Ctrl Pts',(4.46817915202169,8.11367757047581,-0.348488839848436));
#6313=CARTESIAN_POINT('Ctrl Pts',(4.44730202502087,8.03221456672079,-0.696888352951045));
#6314=CARTESIAN_POINT('Ctrl Pts',(4.42642489802006,7.86900111094028,-1.00148282333643));
#6315=CARTESIAN_POINT('Ctrl Pts',(4.38426847041987,7.53943008175988,-1.61653942272961));
#6316=CARTESIAN_POINT('Ctrl Pts',(4.34211204281967,6.87652759730266,-2.05298418236391));
#6317=CARTESIAN_POINT('Ctrl Pts',(4.29995561521948,6.18129213514676,-2.11264435243372));
#6318=CARTESIAN_POINT('Ctrl Pts',(4.25779918761929,5.48605667299086,-2.17230452250352));
#6319=CARTESIAN_POINT('Ctrl Pts',(4.2156427600191,4.75848823313627,-1.85518010300883));
#6320=CARTESIAN_POINT('Ctrl Pts',(4.17348633241891,4.32894761202748,-1.30526507452847));
#6321=CARTESIAN_POINT('Ctrl Pts',(4.13132990481872,3.89940699091868,-0.755350046048115));
#6322=CARTESIAN_POINT('Ctrl Pts',(4.08917347721853,3.76789418855569,0.0273555914179174));
#6323=CARTESIAN_POINT('Ctrl Pts',(4.04701704961834,3.99412410150505,0.687455364346652));
#6324=CARTESIAN_POINT('Ctrl Pts',(4.00486062201815,4.22035401445442,1.34755513727539));
#6325=CARTESIAN_POINT('Ctrl Pts',(3.96270419441795,4.80432664271614,1.88504904566683));
#6326=CARTESIAN_POINT('Ctrl Pts',(3.92054776681776,5.48088251536499,2.05588181452455));
#6327=CARTESIAN_POINT('Ctrl Pts',(3.87839133921757,6.15743838801383,2.22671458338228));
#6328=CARTESIAN_POINT('Ctrl Pts',(3.83623491161738,6.9265775050498,2.03088621270629));
#6329=CARTESIAN_POINT('Ctrl Pts',(3.7940784840172,7.43906342717357,1.55731482067357));
#6330=CARTESIAN_POINT('Ctrl Pts',(3.7590710823523,7.86464029752753,1.1640532261399));
#6331=CARTESIAN_POINT('Ctrl Pts',(3.7240636806874,8.11323120292733,0.579262293111433));
#6332=CARTESIAN_POINT('Ctrl Pts',(3.6890562790225,8.11831511071496,-0.001702946356694));
#6333=CARTESIAN_POINT('Origin',(6.,6.,0.));
#6334=CARTESIAN_POINT('',(2.8890562790225,8.11858235385061,0.0016251550495));
#6335=CARTESIAN_POINT('',(3.11094372097749,8.11439370554494,0.0012559944889576));
#6336=CARTESIAN_POINT('',(6.,8.117,2.59257727379495E-16));
#6337=CARTESIAN_POINT('Ctrl Pts',(3.11094372097749,8.11439370554494,0.0012559944889576));
#6338=CARTESIAN_POINT('Ctrl Pts',(3.12693063610649,8.11584979458628,0.267822697439219));
#6339=CARTESIAN_POINT('Ctrl Pts',(3.14291755123548,8.06908489296678,0.533897341735394));
#6340=CARTESIAN_POINT('Ctrl Pts',(3.15890446636447,7.97174688398804,0.779966710265086));
#6341=CARTESIAN_POINT('Ctrl Pts',(3.20106089396466,7.71507305447496,1.42883520273831));
#6342=CARTESIAN_POINT('Ctrl Pts',(3.24321732156485,7.10674333009371,1.93859867439931));
#6343=CARTESIAN_POINT('Ctrl Pts',(3.28537374916504,6.42297680060745,2.07779317305597));
#6344=CARTESIAN_POINT('Ctrl Pts',(3.32753017676523,5.73921027112117,2.21698767171264));
#6345=CARTESIAN_POINT('Ctrl Pts',(3.36968660436542,4.98000693652988,1.98561319736497));
#6346=CARTESIAN_POINT('Ctrl Pts',(3.41184303196562,4.49009178017005,1.48872798437086));
#6347=CARTESIAN_POINT('Ctrl Pts',(3.45399945956581,4.00017662381023,0.99184277137675));
#6348=CARTESIAN_POINT('Ctrl Pts',(3.496155887166,3.77954964568186,0.229446819736206));
#6349=CARTESIAN_POINT('Ctrl Pts',(3.53831231476619,3.92838905611583,-0.452285242886036));
#6350=CARTESIAN_POINT('Ctrl Pts',(3.58046874236638,4.0772284665498,-1.13401730550828));
#6351=CARTESIAN_POINT('Ctrl Pts',(3.62262516996657,4.59553426554611,-1.73508547911222));
#6352=CARTESIAN_POINT('Ctrl Pts',(3.66478159756676,5.24796375931615,-1.98256786428093));
#6353=CARTESIAN_POINT('Ctrl Pts',(3.70693802516695,5.90039325308621,-2.23005024944964));
#6354=CARTESIAN_POINT('Ctrl Pts',(3.74909445276714,6.68694644163,-2.12394684618312));
#6355=CARTESIAN_POINT('Ctrl Pts',(3.79125088036733,7.25047982671001,-1.71243512191212));
#6356=CARTESIAN_POINT('Ctrl Pts',(3.83114849390405,7.78381812155308,-1.32297290522469));
#6357=CARTESIAN_POINT('Ctrl Pts',(3.87104610744077,8.11739589388198,-0.659954148550725));
#6358=CARTESIAN_POINT('Ctrl Pts',(3.91094372097749,8.12014460849304,0.000668395368594085));
#6359=CARTESIAN_POINT('Ctrl Pts',(3.6890562790225,8.11831511071496,-0.001702946356694));
#6360=CARTESIAN_POINT('Ctrl Pts',(3.68190725308721,8.11935331940506,-0.120344586893705));
#6361=CARTESIAN_POINT('Ctrl Pts',(3.67475822715191,8.11023639929483,-0.238826682073759));
#6362=CARTESIAN_POINT('Ctrl Pts',(3.66760920121662,8.09039782422567,-0.355485491400828));
#6363=CARTESIAN_POINT('Ctrl Pts',(3.62545277361643,7.97341357194241,-1.04339999805302));
#6364=CARTESIAN_POINT('Ctrl Pts',(3.58329634601624,7.48361234016431,-1.66791459796793));
#6365=CARTESIAN_POINT('Ctrl Pts',(3.54113991841605,6.84339399694864,-1.94546127284174));
#6366=CARTESIAN_POINT('Ctrl Pts',(3.49898349081586,6.20317565373296,-2.22300794771556));
#6367=CARTESIAN_POINT('Ctrl Pts',(3.45682706321567,5.41254019907969,-2.15358669754827));
#6368=CARTESIAN_POINT('Ctrl Pts',(3.41467063561547,4.83048473098684,-1.76871903748089));
#6369=CARTESIAN_POINT('Ctrl Pts',(3.37251420801528,4.24842926289399,-1.38385137741351));
#6370=CARTESIAN_POINT('Ctrl Pts',(3.33035778041509,3.87495378136155,-0.683537307446053));
#6371=CARTESIAN_POINT('Ctrl Pts',(3.2882013528149,3.87963911310041,0.014237535530621));
#6372=CARTESIAN_POINT('Ctrl Pts',(3.24604492521471,3.88432444483927,0.712012378507305));
#6373=CARTESIAN_POINT('Ctrl Pts',(3.20388849761452,4.26717058984945,1.40724799449321));
#6374=CARTESIAN_POINT('Ctrl Pts',(3.16173207001433,4.85434186418734,1.78426467613756));
#6375=CARTESIAN_POINT('Ctrl Pts',(3.11957564241414,5.44151313852524,2.16128135778191));
#6376=CARTESIAN_POINT('Ctrl Pts',(3.07741921481395,6.23300954219084,2.22007910508473));
#6377=CARTESIAN_POINT('Ctrl Pts',(3.03526278721375,6.86944305335818,1.93396012732273));
#6378=CARTESIAN_POINT('Ctrl Pts',(2.99310635961356,7.50587656452552,1.64784114956073));
#6379=CARTESIAN_POINT('Ctrl Pts',(2.95094993201337,7.9872471831946,1.01680544673392));
#6380=CARTESIAN_POINT('Ctrl Pts',(2.90879350441318,8.0949830580151,0.327382016861069));
#6381=CARTESIAN_POINT('Ctrl Pts',(2.90221442928295,8.11179668419298,0.219788257145721));
#6382=CARTESIAN_POINT('Ctrl Pts',(2.89563535415273,8.11951014375889,0.110772418640964));
#6383=CARTESIAN_POINT('Ctrl Pts',(2.8890562790225,8.11858235385061,0.00162515504950001));
#6384=CARTESIAN_POINT('Origin',(6.,6.,0.));
#6385=CARTESIAN_POINT('',(2.0890562790225,8.11361510105375,0.000206967465626595));
#6386=CARTESIAN_POINT('',(2.31094372097749,8.11574927685536,-0.00178855551209614));
#6387=CARTESIAN_POINT('',(6.,8.117,2.59257727379495E-16));
#6388=CARTESIAN_POINT('Ctrl Pts',(2.31094372097749,8.11574927685536,-0.00178855551209614));
#6389=CARTESIAN_POINT('Ctrl Pts',(2.340658737172,8.1117226042171,0.492880798811412));
#6390=CARTESIAN_POINT('Ctrl Pts',(2.37037375336652,7.93849788809162,0.990091593431114));
#6391=CARTESIAN_POINT('Ctrl Pts',(2.40008876956103,7.62158202934387,1.36623773853909));
#6392=CARTESIAN_POINT('Ctrl Pts',(2.44224519716122,7.17197633614156,1.89987290903797));
#6393=CARTESIAN_POINT('Ctrl Pts',(2.48440162476141,6.43316573578127,2.18984315988211));
#6394=CARTESIAN_POINT('Ctrl Pts',(2.5265580523616,5.74061565324586,2.1044841666656));
#6395=CARTESIAN_POINT('Ctrl Pts',(2.5687144799618,5.04806557071046,2.01912517344909));
#6396=CARTESIAN_POINT('Ctrl Pts',(2.61087090756198,4.40177600599992,1.55843693617193));
#6397=CARTESIAN_POINT('Ctrl Pts',(2.65302733516217,4.09520215168382,0.931600236700099));
#6398=CARTESIAN_POINT('Ctrl Pts',(2.69518376276237,3.78862829736771,0.30476353722827));
#6399=CARTESIAN_POINT('Ctrl Pts',(2.73734019036256,3.82177015344603,-0.488221624438216));
#6400=CARTESIAN_POINT('Ctrl Pts',(2.77949661796275,4.17957927904964,-1.08729124041551));
#6401=CARTESIAN_POINT('Ctrl Pts',(2.82165304556294,4.53738840465323,-1.6863608563928));
#6402=CARTESIAN_POINT('Ctrl Pts',(2.86380947316313,5.21986479978211,-2.09151492668089));
#6403=CARTESIAN_POINT('Ctrl Pts',(2.90596590076332,5.91712222865987,-2.11878859712663));
#6404=CARTESIAN_POINT('Ctrl Pts',(2.94812232836351,6.61437965753764,-2.14606226757236));
#6405=CARTESIAN_POINT('Ctrl Pts',(2.99027875596371,7.32641812016429,-1.79545553817573));
#6406=CARTESIAN_POINT('Ctrl Pts',(3.0324351835639,7.72992838415516,-1.22616541683467));
#6407=CARTESIAN_POINT('Ctrl Pts',(3.0586046960351,7.98041609117609,-0.87276628464403));
#6408=CARTESIAN_POINT('Ctrl Pts',(3.0847742085063,8.11201018502086,-0.435095897103462));
#6409=CARTESIAN_POINT('Ctrl Pts',(3.11094372097749,8.11439370554494,0.0012559944889576));
#6410=CARTESIAN_POINT('Ctrl Pts',(2.8890562790225,8.11858235385061,0.00162515504950001));
#6411=CARTESIAN_POINT('Ctrl Pts',(2.85347892655254,8.11356518837803,-0.588605324320554));
#6412=CARTESIAN_POINT('Ctrl Pts',(2.81790157408257,7.85585450325349,-1.18267902888964));
#6413=CARTESIAN_POINT('Ctrl Pts',(2.78232422161261,7.41802088245732,-1.57649921610984));
#6414=CARTESIAN_POINT('Ctrl Pts',(2.74016779401242,6.89922170110715,-2.04314586228899));
#6415=CARTESIAN_POINT('Ctrl Pts',(2.69801136641222,6.12752220743493,-2.22862799772838));
#6416=CARTESIAN_POINT('Ctrl Pts',(2.65585493881203,5.45332140955135,-2.04872533765658));
#6417=CARTESIAN_POINT('Ctrl Pts',(2.61369851121184,4.77912061166776,-1.86882267758478));
#6418=CARTESIAN_POINT('Ctrl Pts',(2.57154208361165,4.20241850957281,-1.3235352220018));
#6419=CARTESIAN_POINT('Ctrl Pts',(2.52938565601146,3.9850733075603,-0.660456982788181));
#6420=CARTESIAN_POINT('Ctrl Pts',(2.48722922841127,3.7677281055478,0.00262125642543298));
#6421=CARTESIAN_POINT('Ctrl Pts',(2.44507280081108,3.90973980361775,0.783490279269671));
#6422=CARTESIAN_POINT('Ctrl Pts',(2.40291637321089,4.34662636274209,1.32758752401669));
#6423=CARTESIAN_POINT('Ctrl Pts',(2.36075994561069,4.78351292186642,1.87168476876371));
#6424=CARTESIAN_POINT('Ctrl Pts',(2.31860351801051,5.51527434204514,2.17901023541351));
#6425=CARTESIAN_POINT('Ctrl Pts',(2.27644709041031,6.20964595300729,2.11001931653322));
#6426=CARTESIAN_POINT('Ctrl Pts',(2.23429066281012,6.90401756396943,2.04102839765292));
#6427=CARTESIAN_POINT('Ctrl Pts',(2.19213423520993,7.56099936571499,1.59572109324253));
#6428=CARTESIAN_POINT('Ctrl Pts',(2.14997780760974,7.882281240332,0.976294204819711));
#6429=CARTESIAN_POINT('Ctrl Pts',(2.129670631414,8.03704595849608,0.677910027609945));
#6430=CARTESIAN_POINT('Ctrl Pts',(2.10936345521825,8.11391332031157,0.33912234063746));
#6431=CARTESIAN_POINT('Ctrl Pts',(2.0890562790225,8.11361510105375,0.000206967465626595));
#6432=CARTESIAN_POINT('Origin',(6.,6.,0.));
#6433=CARTESIAN_POINT('',(1.2890562790225,8.11784406625472,-0.00180833638339553));
#6434=CARTESIAN_POINT('',(1.51094372097749,8.12031955932164,0.000387557394038608));
#6435=CARTESIAN_POINT('',(6.,8.117,2.59257727379495E-16));
#6436=CARTESIAN_POINT('Ctrl Pts',(1.51094372097749,8.12031955932164,0.000387557394038608));
#6437=CARTESIAN_POINT('Ctrl Pts',(1.51223041063733,8.12037363613379,0.0216878003480682));
#6438=CARTESIAN_POINT('Ctrl Pts',(1.51351710029718,8.1200801867452,0.0429865167899391));
#6439=CARTESIAN_POINT('Ctrl Pts',(1.51480378995702,8.11943460408254,0.064274553967799));
#6440=CARTESIAN_POINT('Ctrl Pts',(1.55696021755721,8.09828307109983,0.761744679086335));
#6441=CARTESIAN_POINT('Ctrl Pts',(1.5991166451574,7.6991356766239,1.44775119682358));
#6442=CARTESIAN_POINT('Ctrl Pts',(1.64127307275759,7.10323019476973,1.81080550658276));
#6443=CARTESIAN_POINT('Ctrl Pts',(1.68342950035778,6.50732471291556,2.17385981634195));
#6444=CARTESIAN_POINT('Ctrl Pts',(1.72558592795797,5.71466114368315,2.21396191812306));
#6445=CARTESIAN_POINT('Ctrl Pts',(1.76774235555816,5.08515730617276,1.91290271660692));
#6446=CARTESIAN_POINT('Ctrl Pts',(1.80989878315835,4.45565346866237,1.61184351509078));
#6447=CARTESIAN_POINT('Ctrl Pts',(1.85205521075855,3.98930936287399,0.969623010277392));
#6448=CARTESIAN_POINT('Ctrl Pts',(1.89421163835874,3.89787396725924,0.277848933787433));
#6449=CARTESIAN_POINT('Ctrl Pts',(1.93636806595893,3.80643857164448,-0.413925142702522));
#6450=CARTESIAN_POINT('Ctrl Pts',(1.97852449355912,4.08991188620336,-1.15525279086904));
#6451=CARTESIAN_POINT('Ctrl Pts',(2.02068092115931,4.61957955486217,-1.60952576319302));
#6452=CARTESIAN_POINT('Ctrl Pts',(2.0628373487595,5.14924722352099,-2.06379873551699));
#6453=CARTESIAN_POINT('Ctrl Pts',(2.10499377635969,5.92510924627976,-2.23101703199842));
#6454=CARTESIAN_POINT('Ctrl Pts',(2.14715020395988,6.59487659525853,-2.03525322753699));
#6455=CARTESIAN_POINT('Ctrl Pts',(2.18930663156007,7.2646439442373,-1.83948942307556));
#6456=CARTESIAN_POINT('Ctrl Pts',(2.23146305916027,7.82831661943608,-1.28074351767128));
#6457=CARTESIAN_POINT('Ctrl Pts',(2.27361948676046,8.0299525640133,-0.612720519892336));
#6458=CARTESIAN_POINT('Ctrl Pts',(2.28606089816614,8.08946035163823,-0.415570300650682));
#6459=CARTESIAN_POINT('Ctrl Pts',(2.29850230957181,8.11743520866037,-0.208902188115691));
#6460=CARTESIAN_POINT('Ctrl Pts',(2.31094372097749,8.11574927685536,-0.00178855551209614));
#6461=CARTESIAN_POINT('Ctrl Pts',(2.0890562790225,8.11361510105375,0.000206967465626595));
#6462=CARTESIAN_POINT('Ctrl Pts',(2.06720702761806,8.11329423578549,-0.36444477543956));
#6463=CARTESIAN_POINT('Ctrl Pts',(2.04535777621361,8.02364329923712,-0.729244333175282));
#6464=CARTESIAN_POINT('Ctrl Pts',(2.02350852480917,7.84557375391058,-1.04402616427932));
#6465=CARTESIAN_POINT('Ctrl Pts',(1.98135209720898,7.5020024453837,-1.65137317252026));
#6466=CARTESIAN_POINT('Ctrl Pts',(1.93919566960879,6.8292778808415,-2.07252071656688));
#6467=CARTESIAN_POINT('Ctrl Pts',(1.8970392420086,6.13285838710263,-2.11624224665416));
#6468=CARTESIAN_POINT('Ctrl Pts',(1.8548828144084,5.43643889336376,-2.15996377674144));
#6469=CARTESIAN_POINT('Ctrl Pts',(1.81272638680821,4.71632447042824,-1.82625929286939));
#6470=CARTESIAN_POINT('Ctrl Pts',(1.77056995920802,4.29949129246079,-1.26665052430996));
#6471=CARTESIAN_POINT('Ctrl Pts',(1.72841353160783,3.88265811449333,-0.707041755750532));
#6472=CARTESIAN_POINT('Ctrl Pts',(1.68625710400764,3.76910618149396,0.0784712974962866));
#6473=CARTESIAN_POINT('Ctrl Pts',(1.64410067640745,4.0103951285527,0.733216236499067));
#6474=CARTESIAN_POINT('Ctrl Pts',(1.60194424880726,4.25168407561144,1.38796117550185));
#6475=CARTESIAN_POINT('Ctrl Pts',(1.55978782120707,4.84781390272829,1.9119380002606));
#6476=CARTESIAN_POINT('Ctrl Pts',(1.51763139360688,5.5281048754434,2.0672312925924));
#6477=CARTESIAN_POINT('Ctrl Pts',(1.47547496600669,6.20839584815852,2.2225245849242));
#6478=CARTESIAN_POINT('Ctrl Pts',(1.4333185384065,6.97284796647189,2.00913434482906));
#6479=CARTESIAN_POINT('Ctrl Pts',(1.3911621108063,7.47435325973884,1.52394851450554));
#6480=CARTESIAN_POINT('Ctrl Pts',(1.35712683354504,7.87924695391555,1.13223044923417));
#6481=CARTESIAN_POINT('Ctrl Pts',(1.32309155628377,8.11274534553969,0.563349235438652));
#6482=CARTESIAN_POINT('Ctrl Pts',(1.2890562790225,8.11784406625472,-0.00180833638339553));
#6483=CARTESIAN_POINT('Origin',(6.,6.,0.));
#6484=CARTESIAN_POINT('',(0.489056279022499,8.11901932033641,0.00140296810865748));
#6485=CARTESIAN_POINT('',(0.710943720977492,8.11470858782477,0.00143578057856379));
#6486=CARTESIAN_POINT('',(6.,8.117,2.59257727379495E-16));
#6487=CARTESIAN_POINT('',(0.,4.38007430561128,1.36291222925734));
#6488=CARTESIAN_POINT('Ctrl Pts',(0.489056279022499,8.11901932033641,0.00140296810865748));
#6489=CARTESIAN_POINT('Ctrl Pts',(0.452506802148906,8.11421578579102,-0.604476942141384));
#6490=CARTESIAN_POINT('Ctrl Pts',(0.415957325275312,7.84046069996979,-1.21398493528909));
#6491=CARTESIAN_POINT('Ctrl Pts',(0.379407848401719,7.38152818454084,-1.60833829653761));
#6492=CARTESIAN_POINT('Ctrl Pts',(0.337251420801528,6.85219214432977,-2.0631882792025));
#6493=CARTESIAN_POINT('Ctrl Pts',(0.295094993201336,6.07650567520028,-2.23180772089687));
#6494=CARTESIAN_POINT('Ctrl Pts',(0.252938565601145,5.40656319001716,-2.0360753062762));
#6495=CARTESIAN_POINT('Ctrl Pts',(0.210782138000954,4.73662070483403,-1.84034289165553));
#6496=CARTESIAN_POINT('Ctrl Pts',(0.168625710400764,4.17242220359727,-1.28025862071982));
#6497=CARTESIAN_POINT('Ctrl Pts',(0.126469282800573,3.97047197230393,-0.613532492213474));
#6498=CARTESIAN_POINT('Ctrl Pts',(0.0843128552003818,3.76852174101059,0.0531936362928676));
#6499=CARTESIAN_POINT('Ctrl Pts',(0.0421564276001906,3.92881977966068,0.826561622369841));
#6500=CARTESIAN_POINT('Ctrl Pts',(-4.10547488943358E-16,4.38007430561128,
1.36291222925734));
#6501=CARTESIAN_POINT('',(2.73941575321014E-15,7.62290969130025,1.36522594117828));
#6502=CARTESIAN_POINT('Origin',(0.,6.,0.));
#6503=CARTESIAN_POINT('Ctrl Pts',(1.83880688453542E-15,7.62291087731917,
1.36522686078582));
#6504=CARTESIAN_POINT('Ctrl Pts',(0.0412138930502395,7.1828846899475,1.88675593559338));
#6505=CARTESIAN_POINT('Ctrl Pts',(0.0824277861004772,6.4676702007091,2.17777752652732));
#6506=CARTESIAN_POINT('Ctrl Pts',(0.123641679150715,5.78876582874893,2.10968122595389));
#6507=CARTESIAN_POINT('Ctrl Pts',(0.165798106750906,5.09433536159783,2.04002760790171));
#6508=CARTESIAN_POINT('Ctrl Pts',(0.207954534351097,4.4378947790257,1.59464269864839));
#6509=CARTESIAN_POINT('Ctrl Pts',(0.250110961951288,4.11709999477822,0.975083054204924));
#6510=CARTESIAN_POINT('Ctrl Pts',(0.292267389551479,3.79630521053073,0.355523409761457));
#6511=CARTESIAN_POINT('Ctrl Pts',(0.33442381715167,3.81115622460789,-0.438210969872159));
#6512=CARTESIAN_POINT('Ctrl Pts',(0.376580244751861,4.15512217736644,-1.0453657543706));
#6513=CARTESIAN_POINT('Ctrl Pts',(0.418736672352052,4.49908813012499,-1.65252053886904));
#6514=CARTESIAN_POINT('Ctrl Pts',(0.460893099952243,5.17216902156494,-2.07309572823231));
#6515=CARTESIAN_POINT('Ctrl Pts',(0.503049527552434,5.86863390287868,-2.1163069168661));
#6516=CARTESIAN_POINT('Ctrl Pts',(0.545205955152625,6.56509878419243,-2.15951810549988));
#6517=CARTESIAN_POINT('Ctrl Pts',(0.587362382752816,7.28494765537997,-1.82536529340419));
#6518=CARTESIAN_POINT('Ctrl Pts',(0.629518810353007,7.70138276868319,-1.2654790598419));
#6519=CARTESIAN_POINT('Ctrl Pts',(0.656660447227835,7.96949682081299,-0.905006654858185));
#6520=CARTESIAN_POINT('Ctrl Pts',(0.683802084102664,8.11184009736432,-0.450963451734649));
#6521=CARTESIAN_POINT('Ctrl Pts',(0.710943720977492,8.11470858782477,0.00143578057856379));
#6522=CARTESIAN_POINT('Origin',(-1.7667098902285,6.,0.));
#6523=CARTESIAN_POINT('',(10.5667098902285,8.55613055881109,0.000692374991768108));
#6524=CARTESIAN_POINT('',(10.6332901097715,8.56294738394715,-0.00151514723911262));
#6525=CARTESIAN_POINT('',(-1.7667098902285,8.56,1.96795797265743E-13));
#6526=CARTESIAN_POINT('',(11.,3.52700509758159,0.661737268568548));
#6527=CARTESIAN_POINT('Ctrl Pts',(10.6332901097715,8.56294738394715,-0.00151514723911253));
#6528=CARTESIAN_POINT('Ctrl Pts',(10.6712138846473,8.55815224021585,0.75856012002275));
#6529=CARTESIAN_POINT('Ctrl Pts',(10.7512940871233,7.80014953821704,2.37288083670226));
#6530=CARTESIAN_POINT('Ctrl Pts',(10.8735307171994,5.05723750909054,2.86964862298535));
#6531=CARTESIAN_POINT('Ctrl Pts',(10.9578435723998,3.7461035332853,1.48053551427594));
#6532=CARTESIAN_POINT('Ctrl Pts',(11.,3.52700509758159,0.661737268568548));
#6533=CARTESIAN_POINT('',(11.,3.52264482516731,-0.663092573187412));
#6534=CARTESIAN_POINT('Origin',(11.,6.,0.));
#6535=CARTESIAN_POINT('Ctrl Pts',(10.5667098902285,8.55613055881109,0.000692374991768455));
#6536=CARTESIAN_POINT('Ctrl Pts',(10.5856131785684,8.55709447998632,0.382135007947172));
#6537=CARTESIAN_POINT('Ctrl Pts',(10.6466728945084,8.29863237656664,1.61303232131533));
#6538=CARTESIAN_POINT('Ctrl Pts',(10.7498890380487,6.39745114979413,2.99513375481657));
#6539=CARTESIAN_POINT('Ctrl Pts',(10.8754157862993,3.72901154801984,1.97617806422123));
#6540=CARTESIAN_POINT('Ctrl Pts',(10.9587861069498,3.31045923851014,0.134309204987493));
#6541=CARTESIAN_POINT('Ctrl Pts',(11.,3.52264309213417,-0.663093111866542));
#6542=CARTESIAN_POINT('Origin',(-1.7667098902285,6.,0.));
#6543=CARTESIAN_POINT('',(9.76670989022852,8.56017794259811,-0.00227838993089917));
#6544=CARTESIAN_POINT('',(9.8332901097715,8.56018969728858,0.00227386745556037));
#6545=CARTESIAN_POINT('',(-1.7667098902285,8.56,1.96795797265743E-13));
#6546=CARTESIAN_POINT('Ctrl Pts',(9.8332901097715,8.56018969728858,0.00227386745556094));
#6547=CARTESIAN_POINT('Ctrl Pts',(9.84278555811261,8.5619239206668,0.19309848024452));
#6548=CARTESIAN_POINT('Ctrl Pts',(9.89443743405392,8.45560130267874,1.22920413673615));
#6549=CARTESIAN_POINT('Ctrl Pts',(9.98824573759542,7.04679029023846,2.83433283661117));
#6550=CARTESIAN_POINT('Ctrl Pts',(10.114715020396,4.19673876478062,2.42431673808699));
#6551=CARTESIAN_POINT('Ctrl Pts',(10.2411843031966,2.98450817703985,-0.187132765170506));
#6552=CARTESIAN_POINT('Ctrl Pts',(10.3676535859971,4.51025928781023,-2.62891879005706));
#6553=CARTESIAN_POINT('Ctrl Pts',(10.4941228687977,7.38975050690281,-2.68279483089907));
#6554=CARTESIAN_POINT('Ctrl Pts',(10.5826683767225,8.52099523795925,-1.01548145510355));
#6555=CARTESIAN_POINT('Ctrl Pts',(10.6290574570471,8.56348256743679,-0.0863467511938518));
#6556=CARTESIAN_POINT('Ctrl Pts',(10.6332901097715,8.56294738394715,-0.00151514723911253));
#6557=CARTESIAN_POINT('Ctrl Pts',(9.76670989022852,8.56017794259811,-0.00227838993089905));
#6558=CARTESIAN_POINT('Ctrl Pts',(9.79934127963391,8.55422015044893,0.653508106499575));
#6559=CARTESIAN_POINT('Ctrl Pts',(9.8741290966395,7.96469177299003,2.16602528015955));
#6560=CARTESIAN_POINT('Ctrl Pts',(9.99107334124527,5.42536021041376,2.96628144383517));
#6561=CARTESIAN_POINT('Ctrl Pts',(10.1175426240458,3.20108469038192,1.13796721707783));
#6562=CARTESIAN_POINT('Ctrl Pts',(10.2440119068464,3.51849277787554,-1.72375628994429));
#6563=CARTESIAN_POINT('Ctrl Pts',(10.370481189647,6.08955924048204,-3.02010646233692));
#6564=CARTESIAN_POINT('Ctrl Pts',(10.4780471841077,8.20691992499105,-1.7899878009994));
#6565=CARTESIAN_POINT('Ctrl Pts',(10.5434567509682,8.55494482895709,-0.468524329766603));
#6566=CARTESIAN_POINT('Ctrl Pts',(10.5667098902285,8.55613055881109,0.000692374991768455));
#6567=CARTESIAN_POINT('Origin',(-1.7667098902285,6.,0.));
#6568=CARTESIAN_POINT('',(8.96670989022851,8.56310914092999,0.00141529283217118));
#6569=CARTESIAN_POINT('',(9.03329010977151,8.55605974906037,-0.000687443903475848));
#6570=CARTESIAN_POINT('',(-1.7667098902285,8.56,1.96795797265743E-13));
#6571=CARTESIAN_POINT('Ctrl Pts',(9.03329010977151,8.55605974906037,-0.000687443903475485));
#6572=CARTESIAN_POINT('Ctrl Pts',(9.05651365917814,8.55492325759865,0.467936413943757));
#6573=CARTESIAN_POINT('Ctrl Pts',(9.12189363618496,8.20770079733103,1.78879459009414));
#6574=CARTESIAN_POINT('Ctrl Pts',(9.22943004079197,6.09158700182589,3.02003844763038));
#6575=CARTESIAN_POINT('Ctrl Pts',(9.35589932359257,3.51973505278771,1.72548757686079));
#6576=CARTESIAN_POINT('Ctrl Pts',(9.48236860639312,3.20027345136559,-1.1360152149446));
#6577=CARTESIAN_POINT('Ctrl Pts',(9.6088378891937,5.42329849222802,-2.96588214441775));
#6578=CARTESIAN_POINT('Ctrl Pts',(9.72581172365316,7.96382758357787,-2.16718740977869));
#6579=CARTESIAN_POINT('Ctrl Pts',(9.80062913051243,8.55422458308311,-0.654095215554129));
#6580=CARTESIAN_POINT('Ctrl Pts',(9.8332901097715,8.56018969728858,0.00227386745556094));
#6581=CARTESIAN_POINT('Ctrl Pts',(8.96670989022851,8.56310914092999,0.00141529283217119));
#6582=CARTESIAN_POINT('Ctrl Pts',(8.97091295309924,8.56367105037093,0.0856328852446299));
#6583=CARTESIAN_POINT('Ctrl Pts',(9.01727244357015,8.52181940809711,1.01398191393194));
#6584=CARTESIAN_POINT('Ctrl Pts',(9.10578836164127,7.39114764994812,2.68211257580753));
#6585=CARTESIAN_POINT('Ctrl Pts',(9.23225764444183,4.51233920524947,2.62980711778656));
#6586=CARTESIAN_POINT('Ctrl Pts',(9.35872692724241,2.98451046190918,0.189313428699894));
#6587=CARTESIAN_POINT('Ctrl Pts',(9.48519621004298,4.19511541707917,-2.42310002974361));
#6588=CARTESIAN_POINT('Ctrl Pts',(9.61166549284355,7.04478041145962,-2.83504094672479));
#6589=CARTESIAN_POINT('Ctrl Pts',(9.70550338623873,8.4551913903482,-1.2304126453748));
#6590=CARTESIAN_POINT('Ctrl Pts',(9.75718485203372,8.5619170103734,-0.193701174554917));
#6591=CARTESIAN_POINT('Ctrl Pts',(9.76670989022852,8.56017794259811,-0.00227838993089905));
#6592=CARTESIAN_POINT('Origin',(-1.7667098902285,6.,0.));
#6593=CARTESIAN_POINT('',(8.16670989022851,8.55626010879674,0.000990877615878738));
#6594=CARTESIAN_POINT('',(8.23329010977151,8.56264128899482,-0.00167649574357658));
#6595=CARTESIAN_POINT('',(-1.7667098902285,8.56,1.96795797265743E-13));
#6596=CARTESIAN_POINT('Ctrl Pts',(8.23329010977151,8.56264128899483,-0.00167649574357656));
#6597=CARTESIAN_POINT('Ctrl Pts',(8.27024176024366,8.55700984281851,0.739085961748945));
#6598=CARTESIAN_POINT('Ctrl Pts',(8.349349838316,7.83073784367277,2.33458261140701));
#6599=CARTESIAN_POINT('Ctrl Pts',(8.47061434398854,5.12691841598226,2.89253283821776));
#6600=CARTESIAN_POINT('Ctrl Pts',(8.59708362678912,3.09991409354922,0.847655304587422));
#6601=CARTESIAN_POINT('Ctrl Pts',(8.72355290958968,3.70654441823305,-1.96699739921706));
#6602=CARTESIAN_POINT('Ctrl Pts',(8.85002219239026,6.39591418697016,-2.99537475015773));
#6603=CARTESIAN_POINT('Ctrl Pts',(8.9532679257842,8.29791871706444,-1.61424693683209));
#6604=CARTESIAN_POINT('Ctrl Pts',(9.01435723157795,8.55698626782957,-0.382730613268568));
#6605=CARTESIAN_POINT('Ctrl Pts',(9.03329010977151,8.55605974906037,-0.000687443903475485));
#6606=CARTESIAN_POINT('Ctrl Pts',(8.16670989022851,8.55626010879675,0.000990877615879154));
#6607=CARTESIAN_POINT('Ctrl Pts',(8.18464105416476,8.55753072141938,0.362749854559649));
#6608=CARTESIAN_POINT('Ctrl Pts',(8.24472864570121,8.31724292724533,1.57339815673698));
#6609=CARTESIAN_POINT('Ctrl Pts',(8.34697266483782,6.46649534115966,2.98519705577739));
#6610=CARTESIAN_POINT('Ctrl Pts',(8.4734419476384,3.75360435149572,2.02057565464541));
#6611=CARTESIAN_POINT('Ctrl Pts',(8.59991123043897,3.08071680575365,-0.778976857734081));
#6612=CARTESIAN_POINT('Ctrl Pts',(8.72638051323954,5.05889727484518,-2.87112261147709));
#6613=CARTESIAN_POINT('Ctrl Pts',(8.8486467331694,7.79756931010518,-2.37305769290695));
#6614=CARTESIAN_POINT('Ctrl Pts',(8.92875652549905,8.55803513784869,-0.759063695890689));
#6615=CARTESIAN_POINT('Ctrl Pts',(8.96670989022851,8.56310914092999,0.00141529283217119));
#6616=CARTESIAN_POINT('Origin',(-1.7667098902285,6.,0.));
#6617=CARTESIAN_POINT('',(7.36670989022851,8.55959691261755,-0.00228610741251245));
#6618=CARTESIAN_POINT('',(7.4332901097715,8.56078024286682,0.00222060320983035));
#6619=CARTESIAN_POINT('',(-1.7667098902285,8.56,1.96795797265743E-13));
#6620=CARTESIAN_POINT('Ctrl Pts',(7.4332901097715,8.56078024286682,0.00222060320983052));
#6621=CARTESIAN_POINT('Ctrl Pts',(7.44181343370898,8.56233438151834,0.173408601452246));
#6622=CARTESIAN_POINT('Ctrl Pts',(7.49249318524666,8.46889945863842,1.18960690922781));
#6623=CARTESIAN_POINT('Ctrl Pts',(7.58532936438453,7.11139509225075,2.80959402670167));
#6624=CARTESIAN_POINT('Ctrl Pts',(7.71179864718509,4.25280462794925,2.46502048238232));
#6625=CARTESIAN_POINT('Ctrl Pts',(7.83826792998568,2.98088236599169,-0.118094717771357));
#6626=CARTESIAN_POINT('Ctrl Pts',(7.96473721278624,4.45069009732305,-2.59396539404523));
#6627=CARTESIAN_POINT('Ctrl Pts',(8.09120649558682,7.32746169336768,-2.71419658477305));
#6628=CARTESIAN_POINT('Ctrl Pts',(8.18072412791524,8.51042418873668,-1.05464408413909));
#6629=CARTESIAN_POINT('Ctrl Pts',(8.22808533264347,8.56343449909185,-0.10601563748153));
#6630=CARTESIAN_POINT('Ctrl Pts',(8.23329010977151,8.56264128899483,-0.00167649574357656));
#6631=CARTESIAN_POINT('Ctrl Pts',(7.36670989022851,8.55959691261755,-0.00228610741251249));
#6632=CARTESIAN_POINT('Ctrl Pts',(7.39836915523028,8.55391651318035,0.634333487971607));
#6633=CARTESIAN_POINT('Ctrl Pts',(7.47218484783223,7.99282991711364,2.12759389951714));
#6634=CARTESIAN_POINT('Ctrl Pts',(7.58815696803438,5.49345927251859,2.97866343435355));
#6635=CARTESIAN_POINT('Ctrl Pts',(7.71462625083496,3.22786051088117,1.20177452844665));
#6636=CARTESIAN_POINT('Ctrl Pts',(7.84109553363553,3.47970522104534,-1.66647339916602));
#6637=CARTESIAN_POINT('Ctrl Pts',(7.96756481643612,6.02028744265461,-3.02135859893257));
#6638=CARTESIAN_POINT('Ctrl Pts',(8.07610293530042,8.1848475480372,-1.82939795575266));
#6639=CARTESIAN_POINT('Ctrl Pts',(8.14248462656457,8.55454349263577,-0.487750769631392));
#6640=CARTESIAN_POINT('Ctrl Pts',(8.16670989022851,8.55626010879675,0.000990877615879154));
#6641=CARTESIAN_POINT('Origin',(-1.7667098902285,6.,0.));
#6642=CARTESIAN_POINT('',(6.56670989022851,8.5634960952547,0.00112627048192981));
#6643=CARTESIAN_POINT('',(6.6332901097715,8.55593675522896,-0.000379914223101242));
#6644=CARTESIAN_POINT('',(-1.7667098902285,8.56,1.96795797265743E-13));
#6645=CARTESIAN_POINT('Ctrl Pts',(6.6332901097715,8.55593675522896,-0.000379914223101185));
#6646=CARTESIAN_POINT('Ctrl Pts',(6.65554153477451,8.55533662221984,0.448681681498062));
#6647=CARTESIAN_POINT('Ctrl Pts',(6.7199493873777,8.22922127149936,1.74932780794198));
#6648=CARTESIAN_POINT('Ctrl Pts',(6.8265136675811,6.16073061022695,3.01714820944448));
#6649=CARTESIAN_POINT('Ctrl Pts',(6.95298295038165,3.55990612749904,1.78184161478998));
#6650=CARTESIAN_POINT('Ctrl Pts',(7.07945223318224,3.17498687362254,-1.07159623119251));
#6651=CARTESIAN_POINT('Ctrl Pts',(7.2059215159828,5.35552685433585,-2.95189295389255));
#6652=CARTESIAN_POINT('Ctrl Pts',(7.3238674748459,7.93492814248258,-2.20544944201462));
#6653=CARTESIAN_POINT('Ctrl Pts',(7.39965700610879,8.55464759945723,-0.673288591668638));
#6654=CARTESIAN_POINT('Ctrl Pts',(7.4332901097715,8.56078024286682,0.00222060320983052));
#6655=CARTESIAN_POINT('Ctrl Pts',(6.56670989022851,8.5634960952547,0.00112627048193009));
#6656=CARTESIAN_POINT('Ctrl Pts',(6.56994082869561,8.56385434388583,0.065839391593463));
#6657=CARTESIAN_POINT('Ctrl Pts',(6.61532819476289,8.53238654770584,0.974558164011263));
#6658=CARTESIAN_POINT('Ctrl Pts',(6.70287198843037,7.45221141439524,2.64954738997428));
#6659=CARTESIAN_POINT('Ctrl Pts',(6.82934127123096,4.57296049994168,2.66318937161644));
#6660=CARTESIAN_POINT('Ctrl Pts',(6.95581055403151,2.9896368961606,0.258327983142764));
#6661=CARTESIAN_POINT('Ctrl Pts',(7.0822798368321,4.14009309396666,-2.38112697366136));
#6662=CARTESIAN_POINT('Ctrl Pts',(7.20874911963266,6.97957342511075,-2.8582258953101));
#6663=CARTESIAN_POINT('Ctrl Pts',(7.30355913743147,8.44135714864897,-1.27003732301619));
#6664=CARTESIAN_POINT('Ctrl Pts',(7.35621272763009,8.5614803447349,-0.213368057853144));
#6665=CARTESIAN_POINT('Ctrl Pts',(7.36670989022851,8.55959691261755,-0.00228610741251249));
#6666=CARTESIAN_POINT('Origin',(-1.7667098902285,6.,0.));
#6667=CARTESIAN_POINT('',(5.76670989022851,8.55652251069107,0.00126671358662234));
#6668=CARTESIAN_POINT('',(5.83329010977151,8.56213489230814,-0.00188959574180147));
#6669=CARTESIAN_POINT('',(-1.7667098902285,8.56,1.96795797265743E-13));
#6670=CARTESIAN_POINT('Ctrl Pts',(5.8332901097715,8.56213489230814,-0.00188959574180133));
#6671=CARTESIAN_POINT('Ctrl Pts',(5.86926963584003,8.55615869774258,0.719757450352359));
#6672=CARTESIAN_POINT('Ctrl Pts',(5.94740558950873,7.8621596890749,2.29700868724777));
#6673=CARTESIAN_POINT('Ctrl Pts',(6.06769797077765,5.19339550153742,2.91177039443194));
#6674=CARTESIAN_POINT('Ctrl Pts',(6.19416725357823,3.12008881427174,0.913854041489789));
#6675=CARTESIAN_POINT('Ctrl Pts',(6.32063653637879,3.66209554878131,-1.91395413315054));
#6676=CARTESIAN_POINT('Ctrl Pts',(6.44710581917937,6.32720695415856,-3.00365664748478));
#6677=CARTESIAN_POINT('Ctrl Pts',(6.55132367697694,8.27854620458815,-1.653862511724));
#6678=CARTESIAN_POINT('Ctrl Pts',(6.61338510717432,8.5564736039523,-0.402087770143315));
#6679=CARTESIAN_POINT('Ctrl Pts',(6.6332901097715,8.55593675522896,-0.000379914223101185));
#6680=CARTESIAN_POINT('Ctrl Pts',(5.76670989022851,8.55652251069107,0.00126671358662286));
#6681=CARTESIAN_POINT('Ctrl Pts',(5.78366892976113,8.55806819340342,0.343325249083328));
#6682=CARTESIAN_POINT('Ctrl Pts',(5.84278439689394,8.33538619924687,1.53373602056116));
#6683=CARTESIAN_POINT('Ctrl Pts',(5.94405629162693,6.53474335439746,2.97372979753514));
#6684=CARTESIAN_POINT('Ctrl Pts',(6.07052557442751,3.80047113580028,2.07149514587238));
#6685=CARTESIAN_POINT('Ctrl Pts',(6.19699485722809,3.06364154273657,-0.711911774223792));
#6686=CARTESIAN_POINT('Ctrl Pts',(6.32346414002865,4.99338643380372,-2.84881527870274));
#6687=CARTESIAN_POINT('Ctrl Pts',(6.44670248436214,7.76460713319277,-2.41014488541846));
#6688=CARTESIAN_POINT('Ctrl Pts',(6.52778440109542,8.55918001082909,-0.778520237258299));
#6689=CARTESIAN_POINT('Ctrl Pts',(6.56670989022851,8.5634960952547,0.00112627048193009));
#6690=CARTESIAN_POINT('Origin',(-1.7667098902285,6.,0.));
#6691=CARTESIAN_POINT('',(4.96670989022851,8.55903014885295,-0.00224703052746647));
#6692=CARTESIAN_POINT('',(5.0332901097715,8.56135690444116,0.00211620437658548));
#6693=CARTESIAN_POINT('',(-1.7667098902285,8.56,1.96795797265743E-13));
#6694=CARTESIAN_POINT('Ctrl Pts',(5.0332901097715,8.56135690444116,0.00211620437658528));
#6695=CARTESIAN_POINT('Ctrl Pts',(5.04084130930536,8.56270384795118,0.153691292555975));
#6696=CARTESIAN_POINT('Ctrl Pts',(5.0905489364394,8.48167485146914,1.15003395919758));
#6697=CARTESIAN_POINT('Ctrl Pts',(5.18241299117364,7.17545208301331,2.78340260245806));
#6698=CARTESIAN_POINT('Ctrl Pts',(5.30888227397421,4.30971964307301,2.50439013770165));
#6699=CARTESIAN_POINT('Ctrl Pts',(5.43535155677478,2.97896957548569,-0.0489164695102037));
#6700=CARTESIAN_POINT('Ctrl Pts',(5.56182083957536,4.39168654812479,-2.55780090846567));
#6701=CARTESIAN_POINT('Ctrl Pts',(5.68829012237593,7.26494986606656,-2.74388765862757));
#6702=CARTESIAN_POINT('Ctrl Pts',(5.77877987910798,8.49886688840039,-1.0941409336459));
#6703=CARTESIAN_POINT('Ctrl Pts',(5.82711320823984,8.56316087484319,-0.125780686909922));
#6704=CARTESIAN_POINT('Ctrl Pts',(5.8332901097715,8.56213489230814,-0.00188959574180133));
#6705=CARTESIAN_POINT('Ctrl Pts',(4.96670989022851,8.55903014885295,-0.00224703052746637));
#6706=CARTESIAN_POINT('Ctrl Pts',(4.99739703082665,8.55371858466909,0.615172981798587));
#6707=CARTESIAN_POINT('Ctrl Pts',(5.07024059902498,8.02025392240756,2.08900571630608));
#6708=CARTESIAN_POINT('Ctrl Pts',(5.18524059482349,5.56181288602103,2.98948346992642));
#6709=CARTESIAN_POINT('Ctrl Pts',(5.31170987762408,3.2561120833366,1.26494998502281));
#6710=CARTESIAN_POINT('Ctrl Pts',(5.43817916042463,3.44219885099807,-1.60831360312132));
#6711=CARTESIAN_POINT('Ctrl Pts',(5.56464844322522,5.9510835258896,-3.02103070861275));
#6712=CARTESIAN_POINT('Ctrl Pts',(5.67415868649317,8.16200184373334,-1.86872894720649));
#6713=CARTESIAN_POINT('Ctrl Pts',(5.74151250216094,8.55422596747839,-0.506956741176808));
#6714=CARTESIAN_POINT('Ctrl Pts',(5.76670989022851,8.55652251069107,0.00126671358662286));
#6715=CARTESIAN_POINT('Origin',(-1.7667098902285,6.,0.));
#6716=CARTESIAN_POINT('',(4.16670989022851,8.56380264418621,0.000808262703818619));
#6717=CARTESIAN_POINT('',(4.2332901097715,8.55588550426825,-6.54012209720356E-5));
#6718=CARTESIAN_POINT('',(-1.7667098902285,8.56,1.96795797265743E-13));
#6719=CARTESIAN_POINT('Ctrl Pts',(4.2332901097715,8.55588550426825,-6.54012209719279E-5));
#6720=CARTESIAN_POINT('Ctrl Pts',(4.25456941037088,8.55578681917127,0.429399022051573));
#6721=CARTESIAN_POINT('Ctrl Pts',(4.31800513857044,8.2501018113131,1.70980750910722));
#6722=CARTESIAN_POINT('Ctrl Pts',(4.42359729437019,6.22979061312465,3.01267554193145));
#6723=CARTESIAN_POINT('Ctrl Pts',(4.55006657717078,3.60135595755754,1.83726002636678));
#6724=CARTESIAN_POINT('Ctrl Pts',(4.67653585997134,3.1511849892005,-1.00661347153406));
#6725=CARTESIAN_POINT('Ctrl Pts',(4.80300514277192,5.28808829272449,-2.93635818112757));
#6726=CARTESIAN_POINT('Ctrl Pts',(4.92192322603863,7.90530393143438,-2.24352310907718));
#6727=CARTESIAN_POINT('Ctrl Pts',(4.99868488170516,8.55518420470679,-0.692513896722687));
#6728=CARTESIAN_POINT('Ctrl Pts',(5.0332901097715,8.56135690444116,0.00211620437658528));
#6729=CARTESIAN_POINT('Ctrl Pts',(4.16670989022851,8.56380264418621,0.000808262703819061));
#6730=CARTESIAN_POINT('Ctrl Pts',(4.16896870429198,8.56399082802434,0.0460361249824619));
#6731=CARTESIAN_POINT('Ctrl Pts',(4.21338394595564,8.54247712043068,0.935172573537014));
#6732=CARTESIAN_POINT('Ctrl Pts',(4.29995561521948,7.51251343469132,2.61559218413545));
#6733=CARTESIAN_POINT('Ctrl Pts',(4.42642489802006,4.63433022445025,2.69517447078429));
#6734=CARTESIAN_POINT('Ctrl Pts',(4.55289418082063,2.99634307005063,0.327206984929225));
#6735=CARTESIAN_POINT('Ctrl Pts',(4.6793634636212,4.08604568686072,-2.33790467107576));
#6736=CARTESIAN_POINT('Ctrl Pts',(4.80583274642178,6.91385412742878,-2.87991145655582));
#6737=CARTESIAN_POINT('Ctrl Pts',(4.90161488862421,8.4269861859368,-1.30968214690492));
#6738=CARTESIAN_POINT('Ctrl Pts',(4.95524060322645,8.56101534046309,-0.23300712039416));
#6739=CARTESIAN_POINT('Ctrl Pts',(4.96670989022851,8.55903014885295,-0.00224703052746637));
#6740=CARTESIAN_POINT('Origin',(-1.7667098902285,6.,0.));
#6741=CARTESIAN_POINT('',(3.36670989022851,8.55684831657772,0.00151882186684854));
#6742=CARTESIAN_POINT('',(3.4332901097715,8.56159030865862,-0.00205930216014198));
#6743=CARTESIAN_POINT('',(-1.7667098902285,8.56,1.96795797265743E-13));
#6744=CARTESIAN_POINT('Ctrl Pts',(3.4332901097715,8.56159030865862,-0.00205930216014198));
#6745=CARTESIAN_POINT('Ctrl Pts',(3.46829751143639,8.55544255054036,0.700477784773422));
#6746=CARTESIAN_POINT('Ctrl Pts',(3.54546134070149,7.89283216702593,2.25921760989519));
#6747=CARTESIAN_POINT('Ctrl Pts',(3.66478159756676,5.26029576462132,2.92948037902181));
#6748=CARTESIAN_POINT('Ctrl Pts',(3.79125088036734,3.14177437347817,0.979573332991449));
#6749=CARTESIAN_POINT('Ctrl Pts',(3.9177201631679,3.61887325026032,-1.85990673112716));
#6750=CARTESIAN_POINT('Ctrl Pts',(4.04418944596849,6.25832795884948,-3.01036282074418));
#6751=CARTESIAN_POINT('Ctrl Pts',(4.14937942816968,8.2585551860386,-1.69344410064111));
#6752=CARTESIAN_POINT('Ctrl Pts',(4.21241298277068,8.55598232424093,-0.421413051493609));
#6753=CARTESIAN_POINT('Ctrl Pts',(4.2332901097715,8.55588550426825,-6.54012209719279E-5));
#6754=CARTESIAN_POINT('Ctrl Pts',(3.36670989022851,8.55684831657772,0.00151882186684858));
#6755=CARTESIAN_POINT('Ctrl Pts',(3.3826968053575,8.55860910445953,0.323866842439612));
#6756=CARTESIAN_POINT('Ctrl Pts',(3.44084014808668,8.3529374416759,1.49406099706874));
#6757=CARTESIAN_POINT('Ctrl Pts',(3.54113991841604,6.60271083165986,2.96070245343145));
#6758=CARTESIAN_POINT('Ctrl Pts',(3.66760920121663,3.84849183796069,2.12132788423443));
#6759=CARTESIAN_POINT('Ctrl Pts',(3.79407848401719,3.0481067685106,-0.644473206270731));
#6760=CARTESIAN_POINT('Ctrl Pts',(3.92054776681777,4.92840366803431,-2.82501339204223));
#6761=CARTESIAN_POINT('Ctrl Pts',(4.04475823555487,7.73087773797067,-2.44696898167379));
#6762=CARTESIAN_POINT('Ctrl Pts',(4.12681227669178,8.56047873799623,-0.79805508752461));
#6763=CARTESIAN_POINT('Ctrl Pts',(4.16670989022851,8.56380264418621,0.000808262703819061));
#6764=CARTESIAN_POINT('Origin',(-1.7667098902285,6.,0.));
#6765=CARTESIAN_POINT('',(2.56670989022851,8.55848755255065,-0.00216282574899321));
#6766=CARTESIAN_POINT('',(2.6332901097715,8.56191347466111,0.00196523236974941));
#6767=CARTESIAN_POINT('',(-1.7667098902285,8.56,1.96795797265743E-13));
#6768=CARTESIAN_POINT('Ctrl Pts',(2.6332901097715,8.56191347466111,0.00196523236974947));
#6769=CARTESIAN_POINT('Ctrl Pts',(2.63986918490172,8.56303541238676,0.133952476013648));
#6770=CARTESIAN_POINT('Ctrl Pts',(2.68860468763214,8.49394004679471,1.11049084410191));
#6771=CARTESIAN_POINT('Ctrl Pts',(2.77949661796275,7.23889240500353,2.75575094100713));
#6772=CARTESIAN_POINT('Ctrl Pts',(2.90596590076332,4.36752141768572,2.5424459342591));
#6773=CARTESIAN_POINT('Ctrl Pts',(3.0324351835639,2.97864168519721,0.0202874407439004));
#6774=CARTESIAN_POINT('Ctrl Pts',(3.15890446636446,4.33352675754921,-2.52029454194393));
#6775=CARTESIAN_POINT('Ctrl Pts',(3.28537374916504,7.20177441543159,-2.77213922842707));
#6776=CARTESIAN_POINT('Ctrl Pts',(3.37683563030072,8.48681045755432,-1.13367097303057));
#6777=CARTESIAN_POINT('Ctrl Pts',(3.4261410838362,8.562845771222,-0.145527700731133));
#6778=CARTESIAN_POINT('Ctrl Pts',(3.4332901097715,8.56159030865862,-0.00205930216014198));
#6779=CARTESIAN_POINT('Ctrl Pts',(2.56670989022851,8.55848755255065,-0.00216282574899286));
#6780=CARTESIAN_POINT('Ctrl Pts',(2.59642490642302,8.55361826490113,0.596020238525012));
#6781=CARTESIAN_POINT('Ctrl Pts',(2.66829635021771,8.04696672892027,2.05027352543945));
#6782=CARTESIAN_POINT('Ctrl Pts',(2.78232422161261,5.63039638482652,2.99873515893208));
#6783=CARTESIAN_POINT('Ctrl Pts',(2.90879350441318,3.28580315999094,1.32746181821946));
#6784=CARTESIAN_POINT('Ctrl Pts',(3.03526278721375,3.4060343620134,-1.54931004838359));
#6785=CARTESIAN_POINT('Ctrl Pts',(3.16173207001433,5.88190527112525,-3.01911791792189));
#6786=CARTESIAN_POINT('Ctrl Pts',(3.27221443768591,8.13849045765698,-1.90797857169019));
#6787=CARTESIAN_POINT('Ctrl Pts',(3.34054037775731,8.55396602439938,-0.526143361636563));
#6788=CARTESIAN_POINT('Ctrl Pts',(3.36670989022851,8.55684831657772,0.00151882186684858));
#6789=CARTESIAN_POINT('Origin',(-1.7667098902285,6.,0.));
#6790=CARTESIAN_POINT('',(1.76670989022851,8.56401420494256,0.000468657028373232));
#6791=CARTESIAN_POINT('',(1.8332901097715,8.55590678256854,0.000250277143156217));
#6792=CARTESIAN_POINT('',(-1.7667098902285,8.56,1.96795797265743E-13));
#6793=CARTESIAN_POINT('Ctrl Pts',(1.8332901097715,8.55590678256854,0.000250277143156244));
#6794=CARTESIAN_POINT('Ctrl Pts',(1.85359728596724,8.55626740670647,0.410086533789295));
#6795=CARTESIAN_POINT('Ctrl Pts',(1.91606088976318,8.27035132529504,1.67024228262478));
#6796=CARTESIAN_POINT('Ctrl Pts',(2.02068092115931,6.29873006674212,3.00662229441761));
#6797=CARTESIAN_POINT('Ctrl Pts',(2.14715020395988,3.6440641683139,1.89171460246179));
#6798=CARTESIAN_POINT('Ctrl Pts',(2.27361948676046,3.12887765854667,-0.941102636765302));
#6799=CARTESIAN_POINT('Ctrl Pts',(2.40008876956103,5.221023215509,-2.91928291965494));
#6800=CARTESIAN_POINT('Ctrl Pts',(2.51997897723137,7.87493959029486,-2.28139980516642));
#6801=CARTESIAN_POINT('Ctrl Pts',(2.59771275730153,8.55584642524694,-0.711775923599712));
#6802=CARTESIAN_POINT('Ctrl Pts',(2.6332901097715,8.56191347466111,0.00196523236974947));
#6803=CARTESIAN_POINT('Ctrl Pts',(1.76670989022851,8.56401420494256,0.000468657028373227));
#6804=CARTESIAN_POINT('Ctrl Pts',(1.76799657988834,8.56407959778106,0.0262261544125052));
#6805=CARTESIAN_POINT('Ctrl Pts',(1.81143969714837,8.55209842073233,0.895826509796029));
#6806=CARTESIAN_POINT('Ctrl Pts',(1.89703924200859,7.57202172994746,2.58026440683785));
#6807=CARTESIAN_POINT('Ctrl Pts',(2.02350852480917,4.69641652838636,2.72574581528328));
#6808=CARTESIAN_POINT('Ctrl Pts',(2.14997780760974,3.00462496841716,0.395914224840739));
#6809=CARTESIAN_POINT('Ctrl Pts',(2.27644709041032,4.03300241565958,-2.29345579779455));
#6810=CARTESIAN_POINT('Ctrl Pts',(2.40291637321088,6.8476553843829,-2.90008617898366));
#6811=CARTESIAN_POINT('Ctrl Pts',(2.49967063981696,8.41207197849935,-1.34934333695958));
#6812=CARTESIAN_POINT('Ctrl Pts',(2.55426847882283,8.56052627972158,-0.252616722520519));
#6813=CARTESIAN_POINT('Ctrl Pts',(2.56670989022851,8.55848755255065,-0.00216282574899286));
#6814=CARTESIAN_POINT('Origin',(-1.7667098902285,6.,0.));
#6815=CARTESIAN_POINT('',(0.966709890228505,8.55722909061475,0.00173622970309428));
#6816=CARTESIAN_POINT('',(1.0332901097715,8.5610206941956,-0.00218674593362891));
#6817=CARTESIAN_POINT('',(-1.7667098902285,8.56,1.96795797265743E-13));
#6818=CARTESIAN_POINT('Ctrl Pts',(1.0332901097715,8.5610206941956,-0.00218674593362883));
#6819=CARTESIAN_POINT('Ctrl Pts',(1.06732538703276,8.55485502342069,0.681234786359444));
#6820=CARTESIAN_POINT('Ctrl Pts',(1.14351709189422,7.92276141437229,2.22122903234413));
#6821=CARTESIAN_POINT('Ctrl Pts',(1.26186522435587,5.32758429305789,2.94565042609802));
#6822=CARTESIAN_POINT('Ctrl Pts',(1.38833450715645,3.16495931797173,1.0447803202184));
#6823=CARTESIAN_POINT('Ctrl Pts',(1.51480378995702,3.57690019914092,-1.80488441711536));
#6824=CARTESIAN_POINT('Ctrl Pts',(1.64127307275759,6.18931341035722,-3.01548925232429));
#6825=CARTESIAN_POINT('Ctrl Pts',(1.74743517936242,8.23793676912792,-1.73298413552372));
#6826=CARTESIAN_POINT('Ctrl Pts',(1.81144085836705,8.5555187735526,-0.440707900389815));
#6827=CARTESIAN_POINT('Ctrl Pts',(1.8332901097715,8.55590678256854,0.000250277143156244));
#6828=CARTESIAN_POINT('Ctrl Pts',(0.966709890228505,8.55722909061475,0.00173622970309435));
#6829=CARTESIAN_POINT('Ctrl Pts',(0.981724680953864,8.55914800573449,0.304374756490232));
#6830=CARTESIAN_POINT('Ctrl Pts',(1.03889589927941,8.36991977797047,1.45440284520618));
#6831=CARTESIAN_POINT('Ctrl Pts',(1.13822354520516,6.67035096999308,2.94610350710691));
#6832=CARTESIAN_POINT('Ctrl Pts',(1.26469282800573,3.89764709051462,2.17005731163833));
#6833=CARTESIAN_POINT('Ctrl Pts',(1.39116211080631,3.0341175837159,-0.576701540113256));
#6834=CARTESIAN_POINT('Ctrl Pts',(1.51763139360688,4.8639846740404,-2.79972682418719));
#6835=CARTESIAN_POINT('Ctrl Pts',(1.64281398674761,7.69637500900364,-2.48351535416102));
#6836=CARTESIAN_POINT('Ctrl Pts',(1.72584015228815,8.56193710099446,-0.817679029197883));
#6837=CARTESIAN_POINT('Ctrl Pts',(1.76670989022851,8.56401420494256,0.000468657028373227));
#6838=CARTESIAN_POINT('Origin',(-1.7667098902285,6.,0.));
#6839=CARTESIAN_POINT('',(0.166709890228505,8.55738198002468,-0.00304066224802793));
#6840=CARTESIAN_POINT('',(0.233290109771496,8.56244188004781,0.00169655094858915));
#6841=CARTESIAN_POINT('',(-1.7667098902285,8.56,1.96795797265743E-13));
#6842=CARTESIAN_POINT('',(0.,6.66173726856851,-2.47299490241842));
#6843=CARTESIAN_POINT('Ctrl Pts',(0.,6.66173726856851,-2.47299490241842));
#6844=CARTESIAN_POINT('Ctrl Pts',(0.042156427600191,7.4805355142759,-2.25389646671472));
#6845=CARTESIAN_POINT('Ctrl Pts',(0.0977263910096926,8.39608892768013,-1.38973499298135));
#6846=CARTESIAN_POINT('Ctrl Pts',(0.153296354419194,8.55936199509083,-0.273279593862165));
#6847=CARTESIAN_POINT('Ctrl Pts',(0.166709890228505,8.55738198002468,-0.00304066224802793));
#6848=CARTESIAN_POINT('',(1.04028710533623E-16,5.33690806430729,-2.47735557113815));
#6849=CARTESIAN_POINT('Origin',(0.,6.,0.));
#6850=CARTESIAN_POINT('Ctrl Pts',(-1.76182853028894E-18,5.33690753016716,
-2.47735729053333));
#6851=CARTESIAN_POINT('Ctrl Pts',(0.0412138930502383,6.13431011265186,-2.68954137333078));
#6852=CARTESIAN_POINT('Ctrl Pts',(0.11897726297407,7.85230474856696,-2.29913620624405));
#6853=CARTESIAN_POINT('Ctrl Pts',(0.196740632897902,8.55663316562353,-0.730968810525245));
#6854=CARTESIAN_POINT('Ctrl Pts',(0.233290109771496,8.56244188004781,0.00169655094858908));
#6855=CARTESIAN_POINT('Origin',(2.5,0.,-3.));
#6856=CARTESIAN_POINT('',(0.,1.,-3.));
#6857=CARTESIAN_POINT('Origin',(0.,0.,-3.));
#6858=CARTESIAN_POINT('',(5.,1.,-3.));
#6859=CARTESIAN_POINT('',(2.5,1.,-3.));
#6860=CARTESIAN_POINT('Origin',(5.,0.,-3.));
#6861=CARTESIAN_POINT('Origin',(5.,0.,-3.));
#6862=CARTESIAN_POINT('Origin',(2.5,0.,3.));
#6863=CARTESIAN_POINT('',(0.,1.,3.));
#6864=CARTESIAN_POINT('Origin',(0.,0.,3.));
#6865=CARTESIAN_POINT('',(5.,1.,3.));
#6866=CARTESIAN_POINT('',(2.5,1.,3.));
#6867=CARTESIAN_POINT('Origin',(5.,0.,3.));
#6868=CARTESIAN_POINT('Origin',(5.,0.,3.));
#6869=CARTESIAN_POINT('Origin',(11.,6.,0.));
#6870=CARTESIAN_POINT('Ctrl Pts',(11.,7.36291222925731,-1.61992569438875));
#6871=CARTESIAN_POINT('Ctrl Pts',(11.,7.31083931682775,-1.67389112219309));
#6872=CARTESIAN_POINT('Ctrl Pts',(11.,7.25581777272501,-1.72471964452079));
#6873=CARTESIAN_POINT('Ctrl Pts',(11.,7.19820656866207,-1.77240154562655));
#6874=CARTESIAN_POINT('Ctrl Pts',(11.,7.13906939943468,-1.82134641148449));
#6875=CARTESIAN_POINT('Ctrl Pts',(11.,7.07720303473932,-1.86697624806703));
#6876=CARTESIAN_POINT('Ctrl Pts',(11.,7.0129505096539,-1.90924986985927));
#6877=CARTESIAN_POINT('Ctrl Pts',(11.,6.99905883361936,-1.91838961118404));
#6878=CARTESIAN_POINT('Ctrl Pts',(11.,6.98505362557214,-1.92737349175926));
#6879=CARTESIAN_POINT('Ctrl Pts',(11.,6.97094405837831,-1.93619717947497));
#6880=CARTESIAN_POINT('Ctrl Pts',(11.,6.90417313060292,-1.97795365627432));
#6881=CARTESIAN_POINT('Ctrl Pts',(11.,6.83519118466879,-2.01605003484858));
#6882=CARTESIAN_POINT('Ctrl Pts',(11.,6.76437461164589,-2.05045793329471));
#6883=CARTESIAN_POINT('Ctrl Pts',(11.,6.70878554997294,-2.07746718702039));
#6884=CARTESIAN_POINT('Ctrl Pts',(11.,6.65206493296289,-2.10220311337323));
#6885=CARTESIAN_POINT('Ctrl Pts',(11.,6.59437882701511,-2.12463622451561));
#6886=CARTESIAN_POINT('Ctrl Pts',(11.,6.57496243421673,-2.13218691788403));
#6887=CARTESIAN_POINT('Ctrl Pts',(11.,6.55543656169613,-2.13947659865928));
#6888=CARTESIAN_POINT('Ctrl Pts',(11.,6.53580726721147,-2.14650375048553));
#6889=CARTESIAN_POINT('Ctrl Pts',(11.,6.51922223942772,-2.15244107586267));
#6890=CARTESIAN_POINT('Ctrl Pts',(11.,6.5025612632835,-2.15819155491499));
#6891=CARTESIAN_POINT('Ctrl Pts',(11.,6.48585004814776,-2.16374720263022));
#6892=CARTESIAN_POINT('Ctrl Pts',(11.,6.40908866330734,-2.18926654451187));
#6893=CARTESIAN_POINT('Ctrl Pts',(11.,6.33117162879884,-2.21071471076539));
#6894=CARTESIAN_POINT('Ctrl Pts',(11.,6.25247824483006,-2.22806194232001));
#6895=CARTESIAN_POINT('Ctrl Pts',(11.,6.17264608791968,-2.24566020587898));
#6896=CARTESIAN_POINT('Ctrl Pts',(11.,6.09201408999904,-2.25903848278578));
#6897=CARTESIAN_POINT('Ctrl Pts',(11.,6.0109467640778,-2.26812293923578));
#6898=CARTESIAN_POINT('Ctrl Pts',(11.,5.93065938032486,-2.277119994867));
#6899=CARTESIAN_POINT('Ctrl Pts',(11.,5.84994403510389,-2.28190578244251));
#6900=CARTESIAN_POINT('Ctrl Pts',(11.,5.76913803616273,-2.28236102601123));
#6901=CARTESIAN_POINT('Ctrl Pts',(11.,5.73623455271216,-2.28254639713993));
#6902=CARTESIAN_POINT('Ctrl Pts',(11.,5.70331592490547,-2.28201316467977));
#6903=CARTESIAN_POINT('Ctrl Pts',(11.,5.67040468508686,-2.28075078754997));
#6904=CARTESIAN_POINT('Ctrl Pts',(11.,5.65686480751649,-2.28023143817633));
#6905=CARTESIAN_POINT('Ctrl Pts',(11.,5.64332427555182,-2.27958848039974));
#6906=CARTESIAN_POINT('Ctrl Pts',(11.,5.62980206611338,-2.27882230599476));
#6907=CARTESIAN_POINT('Ctrl Pts',(11.,5.54615795497388,-2.27408299343094));
#6908=CARTESIAN_POINT('Ctrl Pts',(11.,5.46307785440037,-2.26462914348589));
#6909=CARTESIAN_POINT('Ctrl Pts',(11.,5.38093981928942,-2.25039680394637));
#6910=CARTESIAN_POINT('Ctrl Pts',(11.,5.36156670336747,-2.24703995759173));
#6911=CARTESIAN_POINT('Ctrl Pts',(11.,5.34224591428098,-2.24341706956682));
#6912=CARTESIAN_POINT('Ctrl Pts',(11.,5.32298228814404,-2.23952689585244));
#6913=CARTESIAN_POINT('Ctrl Pts',(11.,5.24431074388793,-2.22363964952824));
#6914=CARTESIAN_POINT('Ctrl Pts',(11.,5.1665925882148,-2.2032986905466));
#6915=CARTESIAN_POINT('Ctrl Pts',(11.,5.0900490421026,-2.1787929080781));
#6916=CARTESIAN_POINT('Ctrl Pts',(11.,5.01174129876329,-2.1537223094275));
#6917=CARTESIAN_POINT('Ctrl Pts',(11.,4.93466218929701,-2.12429244228821));
#6918=CARTESIAN_POINT('Ctrl Pts',(11.,4.85905468736252,-2.09075876968975));
#6919=CARTESIAN_POINT('Ctrl Pts',(11.,4.84209216260409,-2.08323549835901));
#6920=CARTESIAN_POINT('Ctrl Pts',(11.,4.82520375806804,-2.07550546979706));
#6921=CARTESIAN_POINT('Ctrl Pts',(11.,4.80839231975368,-2.06757122910378));
#6922=CARTESIAN_POINT('Ctrl Pts',(11.,4.79129520538481,-2.05950216219669));
#6923=CARTESIAN_POINT('Ctrl Pts',(11.,4.77427243502448,-2.05121911042241));
#6924=CARTESIAN_POINT('Ctrl Pts',(11.,4.7573567617439,-2.04273992899805));
#6925=CARTESIAN_POINT('Ctrl Pts',(11.,4.68205610488726,-2.00499458358553));
#6926=CARTESIAN_POINT('Ctrl Pts',(11.,4.60878482621383,-1.96332639890493));
#6927=CARTESIAN_POINT('Ctrl Pts',(11.,4.53777905821884,-1.91806485765549));
#6928=CARTESIAN_POINT('Ctrl Pts',(11.,4.46532239493622,-1.87187846538671));
#6929=CARTESIAN_POINT('Ctrl Pts',(11.,4.39522396629416,-1.82195001563772));
#6930=CARTESIAN_POINT('Ctrl Pts',(11.,4.32774333179297,-1.76857493043294));
#6931=CARTESIAN_POINT('Ctrl Pts',(11.,4.25977928024263,-1.71481747736249));
#6932=CARTESIAN_POINT('Ctrl Pts',(11.,4.19446979653655,-1.65756332034335));
#6933=CARTESIAN_POINT('Ctrl Pts',(11.,4.13210143705822,-1.59706609202154));
#6934=CARTESIAN_POINT('Ctrl Pts',(11.,4.11241075428857,-1.57796615510975));
#6935=CARTESIAN_POINT('Ctrl Pts',(11.,4.09301344480314,-1.55854263321621));
#6936=CARTESIAN_POINT('Ctrl Pts',(11.,4.07391918281171,-1.53880264867837));
#6937=CARTESIAN_POINT('Ctrl Pts',(11.,4.06113823260671,-1.5255894771225));
#6938=CARTESIAN_POINT('Ctrl Pts',(11.,4.04849306806107,-1.51223450831911));
#6939=CARTESIAN_POINT('Ctrl Pts',(11.,4.03598668555857,-1.49873978569596));
#6940=CARTESIAN_POINT('Ctrl Pts',(11.,4.02703668266137,-1.48908249218603));
#6941=CARTESIAN_POINT('Ctrl Pts',(11.,4.01815874529529,-1.47935459918655));
#6942=CARTESIAN_POINT('Ctrl Pts',(11.,4.00936203992878,-1.46956616048432));
#6943=CARTESIAN_POINT('Ctrl Pts',(11.,3.94979319594867,-1.40328157397517));
#6944=CARTESIAN_POINT('Ctrl Pts',(11.,3.89384398506478,-1.33411346169234));
#6945=CARTESIAN_POINT('Ctrl Pts',(11.,3.84178206189435,-1.26237691191309));
#6946=CARTESIAN_POINT('Ctrl Pts',(11.,3.7896896723596,-1.19059838228127));
#6947=CARTESIAN_POINT('Ctrl Pts',(11.,3.74148825905101,-1.11624778861253));
#6948=CARTESIAN_POINT('Ctrl Pts',(11.,3.69747310618552,-1.03959646371966));
#6949=CARTESIAN_POINT('Ctrl Pts',(11.,3.65443166340002,-0.964640831397038));
#6950=CARTESIAN_POINT('Ctrl Pts',(11.,3.61539263220366,-0.887484432473658));
#6951=CARTESIAN_POINT('Ctrl Pts',(11.,3.58066926892089,-0.808348627556223));
#6952=CARTESIAN_POINT('Ctrl Pts',(11.,3.56732500935102,-0.777936575777442));
#6953=CARTESIAN_POINT('Ctrl Pts',(11.,3.55461857152964,-0.747231898960612));
#6954=CARTESIAN_POINT('Ctrl Pts',(11.,3.54256956733971,-0.716246178019685));
#6955=CARTESIAN_POINT('Ctrl Pts',(11.,3.53571486427718,-0.698618338168349));
#6956=CARTESIAN_POINT('Ctrl Pts',(11.,3.52907296049142,-0.680899529254575));
#6957=CARTESIAN_POINT('Ctrl Pts',(11.,3.52264309213416,-0.663093111866506));
#6958=CARTESIAN_POINT('Ctrl Pts',(11.,3.52700509758159,0.661737268568549));
#6959=CARTESIAN_POINT('Ctrl Pts',(11.,3.55700783839337,0.744600185400307));
#6960=CARTESIAN_POINT('Ctrl Pts',(11.,3.59157342721284,0.825613106651542));
#6961=CARTESIAN_POINT('Ctrl Pts',(11.,3.63039754344568,0.904544394731748));
#6962=CARTESIAN_POINT('Ctrl Pts',(11.,3.67052378457075,0.9861229650931));
#6963=CARTESIAN_POINT('Ctrl Pts',(11.,3.71519964166936,1.06547878949095));
#6964=CARTESIAN_POINT('Ctrl Pts',(11.,3.76413235433514,1.14231972468823));
#6965=CARTESIAN_POINT('Ctrl Pts',(11.,3.77380220479441,1.1575046656414));
#6966=CARTESIAN_POINT('Ctrl Pts',(11.,3.78363840594323,1.17259126130582));
#6967=CARTESIAN_POINT('Ctrl Pts',(11.,3.79363885408994,1.18757704999784));
#6968=CARTESIAN_POINT('Ctrl Pts',(11.,3.80363720316686,1.20255969320921));
#6969=CARTESIAN_POINT('Ctrl Pts',(11.,3.81379421168505,1.21743327691453));
#6970=CARTESIAN_POINT('Ctrl Pts',(11.,3.8241061116684,1.23219400682824));
#6971=CARTESIAN_POINT('Ctrl Pts',(11.,3.87459514587875,1.30446536310462));
#6972=CARTESIAN_POINT('Ctrl Pts',(11.,3.92880390516673,1.37404842935174));
#6973=CARTESIAN_POINT('Ctrl Pts',(11.,3.98645173205705,1.44068424654798));
#6974=CARTESIAN_POINT('Ctrl Pts',(11.,4.02844581867207,1.48922571688519));
#6975=CARTESIAN_POINT('Ctrl Pts',(11.,4.07226572854448,1.5362025213652));
#6976=CARTESIAN_POINT('Ctrl Pts',(11.,4.11781249583983,1.58149996077335));
#6977=CARTESIAN_POINT('Ctrl Pts',(11.,4.13416564266894,1.59776358872352));
#6978=CARTESIAN_POINT('Ctrl Pts',(11.,4.15074145945183,1.61381060316234));
#6979=CARTESIAN_POINT('Ctrl Pts',(11.,4.16753554575574,1.62963525480062));
#6980=CARTESIAN_POINT('Ctrl Pts',(11.,4.17867242794955,1.64012926309999));
#6981=CARTESIAN_POINT('Ctrl Pts',(11.,4.18989915573443,1.65051965601333));
#6982=CARTESIAN_POINT('Ctrl Pts',(11.,4.20121078938897,1.66080208045739));
#6983=CARTESIAN_POINT('Ctrl Pts',(11.,4.26495358312366,1.71874512214768));
#6984=CARTESIAN_POINT('Ctrl Pts',(11.,4.33142426322727,1.77329526969942));
#6985=CARTESIAN_POINT('Ctrl Pts',(11.,4.40035782940769,1.82421550306439));
#6986=CARTESIAN_POINT('Ctrl Pts',(11.,4.46792796306447,1.87412858844431));
#6987=CARTESIAN_POINT('Ctrl Pts',(11.,4.53786533886277,1.92055429834348));
#6988=CARTESIAN_POINT('Ctrl Pts',(11.,4.60994183541066,1.96322520805592));
#6989=CARTESIAN_POINT('Ctrl Pts',(11.,4.68054091417581,2.00502145315738));
#6990=CARTESIAN_POINT('Ctrl Pts',(11.,4.75319300565908,2.04321554640376));
#6991=CARTESIAN_POINT('Ctrl Pts',(11.,4.8276935472168,2.07750853757716));
#6992=CARTESIAN_POINT('Ctrl Pts',(11.,4.84971666822096,2.08764589602336));
#6993=CARTESIAN_POINT('Ctrl Pts',(11.,4.87190134628269,2.09744201703478));
#6994=CARTESIAN_POINT('Ctrl Pts',(11.,4.894242333991,2.10688830013711));
#6995=CARTESIAN_POINT('Ctrl Pts',(11.,4.91136213968559,2.11412694747713));
#6996=CARTESIAN_POINT('Ctrl Pts',(11.,4.92857373206428,2.12116015855725));
#6997=CARTESIAN_POINT('Ctrl Pts',(11.,4.94587474276473,2.12798389426578));
#6998=CARTESIAN_POINT('Ctrl Pts',(11.,4.95784258387274,2.13270416096792));
#6999=CARTESIAN_POINT('Ctrl Pts',(11.,4.96985037892949,2.13732300901462));
#7000=CARTESIAN_POINT('Ctrl Pts',(11.,4.98188766633085,2.14183578609736));
#7001=CARTESIAN_POINT('Ctrl Pts',(11.,5.05807742653212,2.1703993147655));
#7002=CARTESIAN_POINT('Ctrl Pts',(11.,5.13555879779739,2.19476158193379));
#7003=CARTESIAN_POINT('Ctrl Pts',(11.,5.21411802734496,2.21467977829964));
#7004=CARTESIAN_POINT('Ctrl Pts',(11.,5.23291149806021,2.21944474407461));
#7005=CARTESIAN_POINT('Ctrl Pts',(11.,5.25176670167758,2.22395514964206));
#7006=CARTESIAN_POINT('Ctrl Pts',(11.,5.27068078412276,2.22820722848632));
#7007=CARTESIAN_POINT('Ctrl Pts',(11.,5.35116102401766,2.24630000810856));
#7008=CARTESIAN_POINT('Ctrl Pts',(11.,5.43270762797145,2.25971979742273));
#7009=CARTESIAN_POINT('Ctrl Pts',(11.,5.51494305755207,2.26856875626421));
#7010=CARTESIAN_POINT('Ctrl Pts',(11.,5.59661107854833,2.27735665899842));
#7011=CARTESIAN_POINT('Ctrl Pts',(11.,5.67895943723679,2.28163617924203));
#7012=CARTESIAN_POINT('Ctrl Pts',(11.,5.76160564919763,2.28145921133302));
#7013=CARTESIAN_POINT('Ctrl Pts',(11.,5.78186348856166,2.28141583381591));
#7014=CARTESIAN_POINT('Ctrl Pts',(11.,5.80213912408603,2.28110449219973));
#7015=CARTESIAN_POINT('Ctrl Pts',(11.,5.82242670183261,2.28052554761898));
#7016=CARTESIAN_POINT('Ctrl Pts',(11.,5.83510702244445,2.28016369057562));
#7017=CARTESIAN_POINT('Ctrl Pts',(11.,5.84779126773273,2.279697238232));
#7018=CARTESIAN_POINT('Ctrl Pts',(11.,5.86046497453528,2.27912708463001));
#7019=CARTESIAN_POINT('Ctrl Pts',(11.,5.94193573517864,2.27546194953095));
#7020=CARTESIAN_POINT('Ctrl Pts',(11.,6.02311364079001,2.26751240450731));
#7021=CARTESIAN_POINT('Ctrl Pts',(11.,6.10364003765459,2.25539767789523));
#7022=CARTESIAN_POINT('Ctrl Pts',(11.,6.1840010683229,2.24330782966262));
#7023=CARTESIAN_POINT('Ctrl Pts',(11.,6.26371425736774,2.22706947431953));
#7024=CARTESIAN_POINT('Ctrl Pts',(11.,6.3424068145887,2.20675222785943));
#7025=CARTESIAN_POINT('Ctrl Pts',(11.,6.41967103165265,2.1868037575584));
#7026=CARTESIAN_POINT('Ctrl Pts',(11.,6.4959521525711,2.1629226440025));
#7027=CARTESIAN_POINT('Ctrl Pts',(11.,6.57086824905388,2.13513440109465));
#7028=CARTESIAN_POINT('Ctrl Pts',(11.,6.60273655364754,2.12331365454369));
#7029=CARTESIAN_POINT('Ctrl Pts',(11.,6.63435741757429,2.11078543462592));
#7030=CARTESIAN_POINT('Ctrl Pts',(11.,6.66569925751203,2.0975497444889));
#7031=CARTESIAN_POINT('Ctrl Pts',(11.,6.67839502656549,2.09218830860714));
#7032=CARTESIAN_POINT('Ctrl Pts',(11.,6.69104621760511,2.08671013926857));
#7033=CARTESIAN_POINT('Ctrl Pts',(11.,6.70363420806782,2.08112276730685));
#7034=CARTESIAN_POINT('Ctrl Pts',(11.,6.77529401289249,2.04931546768698));
#7035=CARTESIAN_POINT('Ctrl Pts',(11.,6.84503127970776,2.0139218522668));
#7036=CARTESIAN_POINT('Ctrl Pts',(11.,6.91250997861022,1.97501181763712));
#7037=CARTESIAN_POINT('Ctrl Pts',(11.,6.97881475247944,1.93677869978917));
#7038=CARTESIAN_POINT('Ctrl Pts',(11.,7.04293957659776,1.89514998025919));
#7039=CARTESIAN_POINT('Ctrl Pts',(11.,7.10453240739252,1.850155007327));
#7040=CARTESIAN_POINT('Ctrl Pts',(11.,7.16414024895716,1.8066101144695));
#7041=CARTESIAN_POINT('Ctrl Pts',(11.,7.22137713707371,1.75991198779978));
#7042=CARTESIAN_POINT('Ctrl Pts',(11.,7.27588415466789,1.71005912218383));
#7043=CARTESIAN_POINT('Ctrl Pts',(11.,7.29498429594792,1.69258987109458));
#7044=CARTESIAN_POINT('Ctrl Pts',(11.,7.31374883354313,1.67473301722448));
#7045=CARTESIAN_POINT('Ctrl Pts',(11.,7.33216095377102,1.65648779355698));
#7046=CARTESIAN_POINT('Ctrl Pts',(11.,7.34331288097895,1.64543695293058));
#7047=CARTESIAN_POINT('Ctrl Pts',(11.,7.3543355061197,1.63424362832598));
#7048=CARTESIAN_POINT('Ctrl Pts',(11.,7.36522742428746,1.62291062336284));
#7049=CARTESIAN_POINT('Origin',(-1.7667098902285,6.,0.));
#7050=CARTESIAN_POINT('Ctrl Pts',(0.233290109771496,8.56244188004781,0.00169655094858908));
#7051=CARTESIAN_POINT('Ctrl Pts',(0.238897060498093,8.56333297831645,0.114092648848322));
#7052=CARTESIAN_POINT('Ctrl Pts',(0.286660438824881,8.50572313696992,1.07067066579831));
#7053=CARTESIAN_POINT('Ctrl Pts',(0.376580244751861,7.30166397004841,2.72694193252232));
#7054=CARTESIAN_POINT('Ctrl Pts',(0.503049527552434,4.42618944743245,2.57901724514726));
#7055=CARTESIAN_POINT('Ctrl Pts',(0.629518810353006,2.97989373731284,0.0895594277083228));
#7056=CARTESIAN_POINT('Ctrl Pts',(0.755988093153581,4.27624391707079,-2.48150710395807));
#7057=CARTESIAN_POINT('Ctrl Pts',(0.882457375954154,7.13796708616038,-2.79891497944178));
#7058=CARTESIAN_POINT('Ctrl Pts',(0.974891381493459,8.47424725723099,-1.17323432323149));
#7059=CARTESIAN_POINT('Ctrl Pts',(1.02516895943257,8.56249188360061,-0.165257813814287));
#7060=CARTESIAN_POINT('Ctrl Pts',(1.0332901097715,8.5610206941956,-0.00218674593362883));
#7061=CARTESIAN_POINT('Ctrl Pts',(0.166709890228505,8.55738198002468,-0.00304066224802793));
#7062=CARTESIAN_POINT('Ctrl Pts',(0.195452782019385,8.55313914952871,0.576034719477703));
#7063=CARTESIAN_POINT('Ctrl Pts',(0.266352101410457,8.07386839878632,2.0128937423642));
#7064=CARTESIAN_POINT('Ctrl Pts',(0.379407848401719,5.69862372086684,3.00550592532682));
#7065=CARTESIAN_POINT('Ctrl Pts',(0.505877131202292,3.31720488565003,1.38974961778526));
#7066=CARTESIAN_POINT('Ctrl Pts',(0.632346414002866,3.37108102552373,-1.4897402431435));
#7067=CARTESIAN_POINT('Ctrl Pts',(0.758815696803437,5.81286715979806,-3.01549246530217));
#7068=CARTESIAN_POINT('Ctrl Pts',(0.870270188878652,8.11427830150227,-1.94718071880993));
#7069=CARTESIAN_POINT('Ctrl Pts',(0.939568253353674,8.5537603444746,-0.545331335115959));
#7070=CARTESIAN_POINT('Ctrl Pts',(0.966709890228505,8.55722909061475,0.00173622970309435));
#7071=CARTESIAN_POINT('Ctrl Pts',(-2.77555756156289E-16,4.38007430561128,
1.36291222925734));
#7072=CARTESIAN_POINT('Ctrl Pts',(0.0421564276001907,3.92881977966068,0.826561622369841));
#7073=CARTESIAN_POINT('Ctrl Pts',(0.126469282800573,3.60822370236051,-0.720174349784107));
#7074=CARTESIAN_POINT('Ctrl Pts',(0.252938565601145,5.30081920607079,-2.40042716259123));
#7075=CARTESIAN_POINT('Ctrl Pts',(0.37940784840172,7.62787861345926,-1.89456883750813));
#7076=CARTESIAN_POINT('Ctrl Pts',(0.505877131202291,8.47683544733721,0.328672733398138));
#7077=CARTESIAN_POINT('Ctrl Pts',(0.632346414002866,7.07641508773143,2.25505315279287));
#7078=CARTESIAN_POINT('Ctrl Pts',(0.758815696803438,4.69853244539629,2.13272637030342));
#7079=CARTESIAN_POINT('Ctrl Pts',(0.885284979604012,3.50251368823877,0.0740614486166079));
#7080=CARTESIAN_POINT('Ctrl Pts',(1.01175426240458,4.57453452048393,-2.05209005432782));
#7081=CARTESIAN_POINT('Ctrl Pts',(1.13822354520516,6.94104543804747,-2.31457148885869));
#7082=CARTESIAN_POINT('Ctrl Pts',(1.26469282800573,8.45297548944686,-0.4752001569218));
#7083=CARTESIAN_POINT('Ctrl Pts',(1.3911621108063,7.73730008478527,1.79574410473392));
#7084=CARTESIAN_POINT('Ctrl Pts',(1.51763139360688,5.44394372984514,2.43591482501934));
#7085=CARTESIAN_POINT('Ctrl Pts',(1.64410067640745,3.65555424849459,0.863984350743103));
#7086=CARTESIAN_POINT('Ctrl Pts',(1.77056995920802,3.99621004749271,-1.49255480899735));
#7087=CARTESIAN_POINT('Ctrl Pts',(1.8970392420086,6.1565533162993,-2.49366826061349));
#7088=CARTESIAN_POINT('Ctrl Pts',(2.02350852480917,8.17472700992591,-1.23022562847364));
#7089=CARTESIAN_POINT('Ctrl Pts',(2.14997780760974,8.21798116746057,1.15041378883214));
#7090=CARTESIAN_POINT('Ctrl Pts',(2.27644709041031,6.24703576222385,2.48633570206331));
#7091=CARTESIAN_POINT('Ctrl Pts',(2.40291637321089,4.05175150168771,1.56435930211391));
#7092=CARTESIAN_POINT('Ctrl Pts',(2.52938565601146,3.62571640747785,-0.778247766418806));
#7093=CARTESIAN_POINT('Ctrl Pts',(2.65585493881203,5.35582271376271,-2.41411013316777));
#7094=CARTESIAN_POINT('Ctrl Pts',(2.78232422161261,7.67092119477938,-1.8576637268496));
#7095=CARTESIAN_POINT('Ctrl Pts',(2.90879350441318,8.46861780186369,0.385769743907112));
#7096=CARTESIAN_POINT('Ctrl Pts',(3.03526278721376,7.02450594585644,2.27887685238754));
#7097=CARTESIAN_POINT('Ctrl Pts',(3.16173207001433,4.65001673485963,2.1024836104791));
#7098=CARTESIAN_POINT('Ctrl Pts',(3.2882013528149,3.5014782998291,0.0167767625214216));
#7099=CARTESIAN_POINT('Ctrl Pts',(3.41467063561547,4.62190474442643,-2.08416544738097));
#7100=CARTESIAN_POINT('Ctrl Pts',(3.54113991841605,6.9938111083862,-2.29242919788285));
#7101=CARTESIAN_POINT('Ctrl Pts',(3.66760920121662,8.46321480372051,-0.418885398138105));
#7102=CARTESIAN_POINT('Ctrl Pts',(3.7940784840172,7.69571662208578,1.8350578420303));
#7103=CARTESIAN_POINT('Ctrl Pts',(3.92054776681776,5.38829927097786,2.42254295405827));
#7104=CARTESIAN_POINT('Ctrl Pts',(4.04701704961834,3.63638138619269,0.810061228883945));
#7105=CARTESIAN_POINT('Ctrl Pts',(4.17348633241891,4.03091979328168,-1.53805568351414));
#7106=CARTESIAN_POINT('Ctrl Pts',(4.29995561521948,6.21362511284545,-2.48942894199821));
#7107=CARTESIAN_POINT('Ctrl Pts',(4.42642489802006,8.20233256621709,-1.18009466309531));
#7108=CARTESIAN_POINT('Ctrl Pts',(4.55289418082062,8.19105128792784,1.20091065436085));
#7109=CARTESIAN_POINT('Ctrl Pts',(4.67936346362121,6.1900260656191,2.49134145401128));
#7110=CARTESIAN_POINT('Ctrl Pts',(4.80583274642177,4.01643381333958,1.51932792024159));
#7111=CARTESIAN_POINT('Ctrl Pts',(4.93230202922236,3.64416352427244,-0.832422155952186));
#7112=CARTESIAN_POINT('Ctrl Pts',(5.05877131202292,5.41128238894444,-2.42823057400276));
#7113=CARTESIAN_POINT('Ctrl Pts',(5.1852405948235,7.71302922320777,-1.81890709672723));
#7114=CARTESIAN_POINT('Ctrl Pts',(5.31170987762407,8.45913491771966,0.442207646406598));
#7115=CARTESIAN_POINT('Ctrl Pts',(5.43817916042464,6.97204377333561,2.30174348023582));
#7116=CARTESIAN_POINT('Ctrl Pts',(5.56464844322521,4.60221737671311,2.07101325059156));
#7117=CARTESIAN_POINT('Ctrl Pts',(5.6911177260258,3.50174944972781,-0.0404516273254309));
#7118=CARTESIAN_POINT('Ctrl Pts',(5.81758700882635,4.67000016499225,-2.11518145438353));
#7119=CARTESIAN_POINT('Ctrl Pts',(5.94405629162694,7.04605424471208,-2.26906647395101));
#7120=CARTESIAN_POINT('Ctrl Pts',(6.07052557442751,8.47216246510873,-0.362360169163266));
#7121=CARTESIAN_POINT('Ctrl Pts',(6.19699485722808,7.65324323193351,1.87341371889789));
#7122=CARTESIAN_POINT('Ctrl Pts',(6.32346414002865,5.33297588935731,2.40789762695798));
#7123=CARTESIAN_POINT('Ctrl Pts',(6.44993342282923,3.61844844523957,0.755714455403861));
#7124=CARTESIAN_POINT('Ctrl Pts',(6.5764027056298,4.0666626081133,-1.5827503515155));
#7125=CARTESIAN_POINT('Ctrl Pts',(6.70287198843037,6.27058481326315,-2.48388325106456));
#7126=CARTESIAN_POINT('Ctrl Pts',(6.82934127123095,8.22878274143999,-1.1293447824051));
#7127=CARTESIAN_POINT('Ctrl Pts',(6.95581055403152,8.16297192699002,1.25077759379901));
#7128=CARTESIAN_POINT('Ctrl Pts',(7.08227983683209,6.13291668041033,2.49504014038827));
#7129=CARTESIAN_POINT('Ctrl Pts',(7.20874911963267,3.98215674684198,1.47349949160562));
#7130=CARTESIAN_POINT('Ctrl Pts',(7.33521840243324,3.66384656697614,-0.886159852122868));
#7131=CARTESIAN_POINT('Ctrl Pts',(7.46168768523381,5.46705091821445,-2.44107710288693));
#7132=CARTESIAN_POINT('Ctrl Pts',(7.58815696803438,7.75423855804789,-1.77919623074557));
#7133=CARTESIAN_POINT('Ctrl Pts',(7.71462625083496,8.44836191581642,0.498413558841803));
#7134=CARTESIAN_POINT('Ctrl Pts',(7.84109553363553,6.91907164464643,2.32340256036229));
#7135=CARTESIAN_POINT('Ctrl Pts',(7.9675648164361,4.55515132709709,2.03845639109507));
#7136=CARTESIAN_POINT('Ctrl Pts',(8.09403409923669,3.50333123781422,-0.0976587959070175));
#7137=CARTESIAN_POINT('Ctrl Pts',(8.22050338203724,4.71879333438784,-2.14508778874756));
#7138=CARTESIAN_POINT('Ctrl Pts',(8.34697266483783,7.0977485956482,-2.2445133476424));
#7139=CARTESIAN_POINT('Ctrl Pts',(8.47344194763839,8.47981317754976,-0.305644835824586));
#7140=CARTESIAN_POINT('Ctrl Pts',(8.59991123043898,7.60990250675094,1.91078675679009));
#7141=CARTESIAN_POINT('Ctrl Pts',(8.72638051323954,5.27800245571656,2.3919890697293));
#7142=CARTESIAN_POINT('Ctrl Pts',(8.85284979604011,3.60176489689208,0.700971203051395));
#7143=CARTESIAN_POINT('Ctrl Pts',(8.9793190788407,4.10341973960911,-1.62661464614942));
#7144=CARTESIAN_POINT('Ctrl Pts',(9.10578836164126,6.32740247414682,-2.47703451018903));
#7145=CARTESIAN_POINT('Ctrl Pts',(9.23225764444184,8.25406380889129,-1.07800232379207));
#7146=CARTESIAN_POINT('Ctrl Pts',(9.35872692724241,8.13375751216227,1.29998815922553));
#7147=CARTESIAN_POINT('Ctrl Pts',(9.48519621004298,6.0757381573693,2.4974302318881));
#7148=CARTESIAN_POINT('Ctrl Pts',(9.61166549284355,3.94893715107484,1.4268973438337));
#7149=CARTESIAN_POINT('Ctrl Pts',(9.73813477564413,3.68475738146131,-0.93943133204598));
#7150=CARTESIAN_POINT('Ctrl Pts',(9.86460405844469,5.52309488595575,-2.45264550770796));
#7151=CARTESIAN_POINT('Ctrl Pts',(9.99107334124528,7.79453553867095,-1.73854713522886));
#7152=CARTESIAN_POINT('Ctrl Pts',(10.1175426240458,8.43628921595103,0.554348761835227));
#7153=CARTESIAN_POINT('Ctrl Pts',(10.2440119068464,6.86564650173235,2.34386039652572));
#7154=CARTESIAN_POINT('Ctrl Pts',(10.370481189647,4.50878748634398,2.00479630255084));
#7155=CARTESIAN_POINT('Ctrl Pts',(10.4969504724476,3.50632961359115,-0.154750024947643));
#7156=CARTESIAN_POINT('Ctrl Pts',(10.6234197552481,4.76805426261496,-2.1739926088089));
#7157=CARTESIAN_POINT('Ctrl Pts',(10.7498890380487,7.1492585246536,-2.21854556914584));
#7158=CARTESIAN_POINT('Ctrl Pts',(10.8763583208493,8.48541088840014,-0.249223947559238));
#7159=CARTESIAN_POINT('Ctrl Pts',(11.0028276036499,7.56718166314935,1.94803644221398));
#7160=CARTESIAN_POINT('Ctrl Pts',(11.1292968864504,5.22037961200964,2.37306489642968));
#7161=CARTESIAN_POINT('Ctrl Pts',(11.2136097416508,4.13613327342382,1.22433347020397));
#7162=CARTESIAN_POINT('Ctrl Pts',(11.255766169251,3.95494913733603,0.547225702171725));
#7163=CARTESIAN_POINT('Ctrl Pts',(-0.085255389750335,4.26707996100189,1.45797916636347));
#7164=CARTESIAN_POINT('Ctrl Pts',(-0.043098962150144,3.78434917068409,0.884216605633869));
#7165=CARTESIAN_POINT('Ctrl Pts',(0.0412138930502387,3.44139062097895,-0.770408523450359));
#7166=CARTESIAN_POINT('Ctrl Pts',(0.167683175850811,5.25204939159895,-2.56786366598092));
#7167=CARTESIAN_POINT('Ctrl Pts',(0.294152458651385,7.74142769640091,-2.0267203089325));
#7168=CARTESIAN_POINT('Ctrl Pts',(0.420621741451956,8.64960164213652,0.35159857513887));
#7169=CARTESIAN_POINT('Ctrl Pts',(0.547091024252532,7.15149804850376,2.41234941270269));
#7170=CARTESIAN_POINT('Ctrl Pts',(0.673560307053103,4.60775144607501,2.28148999525137));
#7171=CARTESIAN_POINT('Ctrl Pts',(0.800029589853676,3.32830703793013,0.0792274416471788));
#7172=CARTESIAN_POINT('Ctrl Pts',(0.92649887265425,4.47510431934622,-2.19522907087124));
#7173=CARTESIAN_POINT('Ctrl Pts',(1.05296815545482,7.00668598741845,-2.47601931905305));
#7174=CARTESIAN_POINT('Ctrl Pts',(1.1794374382554,8.62407738549864,-0.508346695973345));
#7175=CARTESIAN_POINT('Ctrl Pts',(1.30590672105597,7.85848162116695,1.92100227484841));
#7176=CARTESIAN_POINT('Ctrl Pts',(1.43237600385654,5.40515725091604,2.60582669204557));
#7177=CARTESIAN_POINT('Ctrl Pts',(1.55884528665711,3.49202260498698,0.924249673901536));
#7178=CARTESIAN_POINT('Ctrl Pts',(1.68531456945769,3.8564400980421,-1.59666467837002));
#7179=CARTESIAN_POINT('Ctrl Pts',(1.81178385225826,6.16747334765195,-2.66760859118376));
#7180=CARTESIAN_POINT('Ctrl Pts',(1.93825313505883,8.32642029687239,-1.31603730433789));
#7181=CARTESIAN_POINT('Ctrl Pts',(2.06472241785941,8.37269155278336,1.23065836582043));
#7182=CARTESIAN_POINT('Ctrl Pts',(2.19119170065998,6.26426719706327,2.65976456618141));
#7183=CARTESIAN_POINT('Ctrl Pts',(2.31766098346055,3.91585572389644,1.6734777355632));
#7184=CARTESIAN_POINT('Ctrl Pts',(2.44413026626112,3.46010349116746,-0.832532723200972));
#7185=CARTESIAN_POINT('Ctrl Pts',(2.5705995490617,5.31088954767814,-2.58250106199683));
#7186=CARTESIAN_POINT('Ctrl Pts',(2.69706883186227,7.78747261806504,-1.98724096366182));
#7187=CARTESIAN_POINT('Ctrl Pts',(2.82353811466285,8.64081079292425,0.412678261707595));
#7188=CARTESIAN_POINT('Ctrl Pts',(2.95000739746342,7.09596809890546,2.4378348819274));
#7189=CARTESIAN_POINT('Ctrl Pts',(3.07647668026399,4.555851629135,2.24913771840577));
#7190=CARTESIAN_POINT('Ctrl Pts',(3.20294596306457,3.32719942828513,0.0179469885955816));
#7191=CARTESIAN_POINT('Ctrl Pts',(3.32941524586514,4.52577874880069,-2.22954181223529));
#7192=CARTESIAN_POINT('Ctrl Pts',(3.45588452866571,7.06313221073467,-2.45233254139759));
#7193=CARTESIAN_POINT('Ctrl Pts',(3.58235381146628,8.63503092056008,-0.448103825374002));
#7194=CARTESIAN_POINT('Ctrl Pts',(3.70882309426686,7.81399759572522,1.96305825519663));
#7195=CARTESIAN_POINT('Ctrl Pts',(3.83529237706742,5.34563143552567,2.59152209571278));
#7196=CARTESIAN_POINT('Ctrl Pts',(3.96176165986801,3.47151238195452,0.866565263586447));
#7197=CARTESIAN_POINT('Ctrl Pts',(4.08823094266858,3.89357094560789,-1.64533936605182));
#7198=CARTESIAN_POINT('Ctrl Pts',(4.21470022546915,6.22852606151346,-2.66307356824687));
#7199=CARTESIAN_POINT('Ctrl Pts',(4.34116950826973,8.35595141786789,-1.26240956401662));
#7200=CARTESIAN_POINT('Ctrl Pts',(4.4676387910703,8.34388323888864,1.28467752885019));
#7201=CARTESIAN_POINT('Ctrl Pts',(4.59410807387086,6.20328091478762,2.66511948331801));
#7202=CARTESIAN_POINT('Ctrl Pts',(4.72057735667144,3.87807452807889,1.62530528894999));
#7203=CARTESIAN_POINT('Ctrl Pts',(4.84704663947202,3.47983734591513,-0.890485927812807));
#7204=CARTESIAN_POINT('Ctrl Pts',(4.97351592227259,5.37021769020446,-2.59760644304437));
#7205=CARTESIAN_POINT('Ctrl Pts',(5.09998520507316,7.83251779916133,-1.94578095027001));
#7206=CARTESIAN_POINT('Ctrl Pts',(5.22645448787373,8.63066645110808,0.473052865641068));
#7207=CARTESIAN_POINT('Ctrl Pts',(5.35292377067431,7.03984654322817,2.46229652097656));
#7208=CARTESIAN_POINT('Ctrl Pts',(5.47939305347488,4.50471813216642,2.21547221296159));
#7209=CARTESIAN_POINT('Ctrl Pts',(5.60586233627545,3.32748949164709,-0.0432732413870235));
#7210=CARTESIAN_POINT('Ctrl Pts',(5.73233161907602,4.57722895936978,-2.26272127241091));
#7211=CARTESIAN_POINT('Ctrl Pts',(5.8588009018766,7.11901945183022,-2.42734020217653));
#7212=CARTESIAN_POINT('Ctrl Pts',(5.98527018467717,8.64460270633739,-0.387635803699455));
#7213=CARTESIAN_POINT('Ctrl Pts',(6.11173946747775,7.76856156790366,2.00408956167411));
#7214=CARTESIAN_POINT('Ctrl Pts',(6.23820875027831,5.28644909341736,2.57585521611596));
#7215=CARTESIAN_POINT('Ctrl Pts',(6.3646780330789,3.45232856825029,0.808427650765839));
#7216=CARTESIAN_POINT('Ctrl Pts',(6.49114731587947,3.9318069216693,-1.69315161206052));
#7217=CARTESIAN_POINT('Ctrl Pts',(6.61761659868004,6.2894588602283,-2.65714104987129));
#7218=CARTESIAN_POINT('Ctrl Pts',(6.74408588148061,8.38424656673646,-1.2081197373107));
#7219=CARTESIAN_POINT('Ctrl Pts',(6.87055516428118,8.31384526404822,1.33802282668406));
#7220=CARTESIAN_POINT('Ctrl Pts',(6.99702444708176,6.14218799034921,2.66907616340701));
#7221=CARTESIAN_POINT('Ctrl Pts',(7.12349372988232,3.84140654039433,1.57628019933373));
#7222=CARTESIAN_POINT('Ctrl Pts',(7.24996301268291,3.50089333585828,-0.947971978479414));
#7223=CARTESIAN_POINT('Ctrl Pts',(7.37643229548348,5.42987623025491,-2.61134905322214));
#7224=CARTESIAN_POINT('Ctrl Pts',(7.50290157828404,7.87660160027986,-1.90330014040079));
#7225=CARTESIAN_POINT('Ctrl Pts',(7.62937086108463,8.61914200221331,0.533179297554908));
#7226=CARTESIAN_POINT('Ctrl Pts',(7.75584014388519,6.98317946051453,2.48546638247541));
#7227=CARTESIAN_POINT('Ctrl Pts',(7.88230942668577,4.45436909404781,2.18064442152415));
#7228=CARTESIAN_POINT('Ctrl Pts',(8.00877870948634,3.32918161387337,-0.104470769861797));
#7229=CARTESIAN_POINT('Ctrl Pts',(8.13524799228692,4.62942558869958,-2.29471365718012));
#7230=CARTESIAN_POINT('Ctrl Pts',(8.26171727508748,7.17431962822135,-2.40107442668595));
#7231=CARTESIAN_POINT('Ctrl Pts',(8.38818655788806,8.65278707735367,-0.326964417350377));
#7232=CARTESIAN_POINT('Ctrl Pts',(8.51465584068864,7.72219770600942,2.04406947341078));
#7233=CARTESIAN_POINT('Ctrl Pts',(8.64112512348921,5.22764110913847,2.55883699255878));
#7234=CARTESIAN_POINT('Ctrl Pts',(8.76759440628978,3.43448129577779,0.749865903563404));
#7235=CARTESIAN_POINT('Ctrl Pts',(8.89406368909035,3.97112796581709,-1.74007556383864));
#7236=CARTESIAN_POINT('Ctrl Pts',(9.02053297189094,6.35023971175459,-2.6498145901786));
#7237=CARTESIAN_POINT('Ctrl Pts',(9.14700225469149,8.41129105929893,-1.15319599871568));
#7238=CARTESIAN_POINT('Ctrl Pts',(9.27347153749208,8.28259306213672,1.39066596658451));
#7239=CARTESIAN_POINT('Ctrl Pts',(9.39994082029264,6.08102110552151,2.67163297046886));
#7240=CARTESIAN_POINT('Ctrl Pts',(9.52641010309322,3.80586978497912,1.5264274215094));
#7241=CARTESIAN_POINT('Ctrl Pts',(9.65287938589379,3.52326273809608,-1.00495929301219));
#7242=CARTESIAN_POINT('Ctrl Pts',(9.77934866869437,5.48982942137984,-2.62372438661122));
#7243=CARTESIAN_POINT('Ctrl Pts',(9.90581795149493,7.91970940792481,-1.85981565686425));
#7244=CARTESIAN_POINT('Ctrl Pts',(10.0322872342955,8.60622719779109,0.593016137286807));
#7245=CARTESIAN_POINT('Ctrl Pts',(10.1587565170961,6.92602776456773,2.50735120988754));
#7246=CARTESIAN_POINT('Ctrl Pts',(10.2852257998967,4.40477124582285,2.14463644772956));
#7247=CARTESIAN_POINT('Ctrl Pts',(10.4116950826972,3.33238913474072,-0.165544271688598));
#7248=CARTESIAN_POINT('Ctrl Pts',(10.5381643654978,4.68212260434671,-2.32563466922495));
#7249=CARTESIAN_POINT('Ctrl Pts',(10.6646336482984,7.22942251873667,-2.37329532306358));
#7250=CARTESIAN_POINT('Ctrl Pts',(10.7911029310989,8.65877524418052,-0.266608014441423));
#7251=CARTESIAN_POINT('Ctrl Pts',(10.9175722138995,7.6764969641689,2.08391742849973));
#7252=CARTESIAN_POINT('Ctrl Pts',(11.0440414967001,5.1659989110366,2.53859280528157));
#7253=CARTESIAN_POINT('Ctrl Pts',(11.1283543519005,4.00612336004432,1.30973415156129));
#7254=CARTESIAN_POINT('Ctrl Pts',(11.1705107795007,3.81230112408455,0.585396224303999));
#7255=CARTESIAN_POINT('Ctrl Pts',(-0.17051077950067,4.15408561639251,1.55304610346959));
#7256=CARTESIAN_POINT('Ctrl Pts',(-0.128354351900479,3.6398785617075,0.941871588897895));
#7257=CARTESIAN_POINT('Ctrl Pts',(-0.0440414967000963,3.27455753959738,
-0.820642697116609));
#7258=CARTESIAN_POINT('Ctrl Pts',(0.0824277861004764,5.20327957712712,-2.73530016937061));
#7259=CARTESIAN_POINT('Ctrl Pts',(0.20889706890105,7.85497677934257,-2.15887178035685));
#7260=CARTESIAN_POINT('Ctrl Pts',(0.335366351701623,8.82236783693583,0.374524416879597));
#7261=CARTESIAN_POINT('Ctrl Pts',(0.461835634502195,7.22658100927608,2.56964567261251));
#7262=CARTESIAN_POINT('Ctrl Pts',(0.588304917302769,4.51697044675373,2.43025362019932));
#7263=CARTESIAN_POINT('Ctrl Pts',(0.714774200103341,3.15410038762148,0.0843934346777503));
#7264=CARTESIAN_POINT('Ctrl Pts',(0.841243482903915,4.3756741182085,-2.33836808741465));
#7265=CARTESIAN_POINT('Ctrl Pts',(0.967712765704489,7.07232653678942,-2.63746714924742));
#7266=CARTESIAN_POINT('Ctrl Pts',(1.09418204850506,8.79517928155045,-0.541493235024889));
#7267=CARTESIAN_POINT('Ctrl Pts',(1.22065133130563,7.97966315754858,2.0462604449629));
#7268=CARTESIAN_POINT('Ctrl Pts',(1.34712061410621,5.36637077198697,2.77573855907179));
#7269=CARTESIAN_POINT('Ctrl Pts',(1.47358989690678,3.32849096147935,0.984514997059966));
#7270=CARTESIAN_POINT('Ctrl Pts',(1.60005917970736,3.71667014859151,-1.70077454774269));
#7271=CARTESIAN_POINT('Ctrl Pts',(1.72652846250793,6.17839337900458,-2.84154892175403));
#7272=CARTESIAN_POINT('Ctrl Pts',(1.8529977453085,8.47811358381889,-1.40184898020213));
#7273=CARTESIAN_POINT('Ctrl Pts',(1.97946702810908,8.52740193810615,1.31090294280873));
#7274=CARTESIAN_POINT('Ctrl Pts',(2.10593631090964,6.28149863190269,2.83319343029951));
#7275=CARTESIAN_POINT('Ctrl Pts',(2.23240559371022,3.77995994610518,1.7825961690125));
#7276=CARTESIAN_POINT('Ctrl Pts',(2.35887487651079,3.29449057485706,-0.886817679983138));
#7277=CARTESIAN_POINT('Ctrl Pts',(2.48534415931137,5.26595638159357,-2.75089199082588));
#7278=CARTESIAN_POINT('Ctrl Pts',(2.61181344211193,7.9040240413507,-2.11681820047403));
#7279=CARTESIAN_POINT('Ctrl Pts',(2.73828272491252,8.81300378398482,0.439586779508076));
#7280=CARTESIAN_POINT('Ctrl Pts',(2.86475200771308,7.1674302519545,2.59679291146726));
#7281=CARTESIAN_POINT('Ctrl Pts',(2.99122129051366,4.46168652341036,2.39579182633243));
#7282=CARTESIAN_POINT('Ctrl Pts',(3.11769057331423,3.15292055674116,0.0191172146697414));
#7283=CARTESIAN_POINT('Ctrl Pts',(3.2441598561148,4.42965275317496,-2.37491817708961));
#7284=CARTESIAN_POINT('Ctrl Pts',(3.37062913891538,7.13245331308311,-2.61223588491233));
#7285=CARTESIAN_POINT('Ctrl Pts',(3.49709842171594,8.80684703739969,-0.477322252609899));
#7286=CARTESIAN_POINT('Ctrl Pts',(3.62356770451653,7.93227856936462,2.09105866836297));
#7287=CARTESIAN_POINT('Ctrl Pts',(3.7500369873171,5.30296360007351,2.7605012373673));
#7288=CARTESIAN_POINT('Ctrl Pts',(3.87650627011767,3.30664337771634,0.923069298288947));
#7289=CARTESIAN_POINT('Ctrl Pts',(4.00297555291824,3.75622209793411,-1.75262304858949));
#7290=CARTESIAN_POINT('Ctrl Pts',(4.12944483571881,6.24342701018146,-2.83671819449552));
#7291=CARTESIAN_POINT('Ctrl Pts',(4.2559141185194,8.50957026951867,-1.34472446493793));
#7292=CARTESIAN_POINT('Ctrl Pts',(4.38238340131996,8.49671518984944,1.36844440333954));
#7293=CARTESIAN_POINT('Ctrl Pts',(4.50885268412054,6.21653576395613,2.83889751262473));
#7294=CARTESIAN_POINT('Ctrl Pts',(4.6353219669211,3.73971524281822,1.73128265765839));
#7295=CARTESIAN_POINT('Ctrl Pts',(4.76179124972169,3.31551116755782,-0.948549699673432));
#7296=CARTESIAN_POINT('Ctrl Pts',(4.88826053252225,5.32915299146447,-2.76698231208597));
#7297=CARTESIAN_POINT('Ctrl Pts',(5.01472981532283,7.9520063751149,-2.07265480381278));
#7298=CARTESIAN_POINT('Ctrl Pts',(5.1411990981234,8.80219798449649,0.503898084875541));
#7299=CARTESIAN_POINT('Ctrl Pts',(5.26766838092398,7.10764931312074,2.62284956171731));
#7300=CARTESIAN_POINT('Ctrl Pts',(5.39413766372455,4.40721888761971,2.35993117533163));
#7301=CARTESIAN_POINT('Ctrl Pts',(5.52060694652512,3.15322953356639,-0.0460948554486148));
#7302=CARTESIAN_POINT('Ctrl Pts',(5.6470762293257,4.48445775374728,-2.41026109043829));
#7303=CARTESIAN_POINT('Ctrl Pts',(5.77354551212626,7.1919846589484,-2.58561393040205));
#7304=CARTESIAN_POINT('Ctrl Pts',(5.90001479492684,8.81704294756603,-0.412911438235641));
#7305=CARTESIAN_POINT('Ctrl Pts',(6.02648407772741,7.88387990387384,2.13476540445033));
#7306=CARTESIAN_POINT('Ctrl Pts',(6.15295336052798,5.23992229747739,2.74381280527395));
#7307=CARTESIAN_POINT('Ctrl Pts',(6.27942264332857,3.28620869126101,0.861140846127814));
#7308=CARTESIAN_POINT('Ctrl Pts',(6.40589192612913,3.79695123522531,-1.80355287260552));
#7309=CARTESIAN_POINT('Ctrl Pts',(6.5323612089297,6.30833290719342,-2.83039884867804));
#7310=CARTESIAN_POINT('Ctrl Pts',(6.65883049173028,8.53971039203294,-1.2868946922163));
#7311=CARTESIAN_POINT('Ctrl Pts',(6.78529977453085,8.4647186011064,1.42526805956911));
#7312=CARTESIAN_POINT('Ctrl Pts',(6.91176905733142,6.15145930028808,2.84311218642574));
#7313=CARTESIAN_POINT('Ctrl Pts',(7.038238340132,3.70065633394668,1.67906090706185));
#7314=CARTESIAN_POINT('Ctrl Pts',(7.16470762293257,3.33794010474041,-1.00978410483596));
#7315=CARTESIAN_POINT('Ctrl Pts',(7.29117690573314,5.39270154229538,-2.78162100355734));
#7316=CARTESIAN_POINT('Ctrl Pts',(7.41764618853372,7.99896464251182,-2.02740405005601));
#7317=CARTESIAN_POINT('Ctrl Pts',(7.54411547133428,8.78992208861021,0.567945036268011));
#7318=CARTESIAN_POINT('Ctrl Pts',(7.67058475413486,7.04728727638264,2.64753020458854));
#7319=CARTESIAN_POINT('Ctrl Pts',(7.79705403693543,4.35358686099853,2.32283245195324));
#7320=CARTESIAN_POINT('Ctrl Pts',(7.92352331973601,3.15503198993253,-0.111282743816577));
#7321=CARTESIAN_POINT('Ctrl Pts',(8.04999260253657,4.54005784301132,-2.44433952561267));
#7322=CARTESIAN_POINT('Ctrl Pts',(8.17646188533716,7.25089066079452,-2.5576355057295));
#7323=CARTESIAN_POINT('Ctrl Pts',(8.30293116813772,8.82576097715756,-0.348283998876166));
#7324=CARTESIAN_POINT('Ctrl Pts',(8.42940045093831,7.83449290526792,2.17735219003147));
#7325=CARTESIAN_POINT('Ctrl Pts',(8.55586973373887,5.17727976256035,2.72568491538827));
#7326=CARTESIAN_POINT('Ctrl Pts',(8.68233901653945,3.26719769466351,0.79876060407541));
#7327=CARTESIAN_POINT('Ctrl Pts',(8.80880829934001,3.83883619202506,-1.85353648152785));
#7328=CARTESIAN_POINT('Ctrl Pts',(8.93527758214061,6.37307694936239,-2.82259467016817));
#7329=CARTESIAN_POINT('Ctrl Pts',(9.06174686494116,8.56851830970655,-1.2283896736393));
#7330=CARTESIAN_POINT('Ctrl Pts',(9.18821614774174,8.4314286121112,1.48134377394349));
#7331=CARTESIAN_POINT('Ctrl Pts',(9.31468543054231,6.0863040536737,2.84583570904962));
#7332=CARTESIAN_POINT('Ctrl Pts',(9.44115471334289,3.66280241888341,1.62595749918509));
#7333=CARTESIAN_POINT('Ctrl Pts',(9.56762399614345,3.36176809473084,-1.07048725397839));
#7334=CARTESIAN_POINT('Ctrl Pts',(9.69409327894404,5.45656395680392,-2.79480326551449));
#7335=CARTESIAN_POINT('Ctrl Pts',(9.8205625617446,8.04488327717867,-1.98108417849965));
#7336=CARTESIAN_POINT('Ctrl Pts',(9.94703184454518,8.77616517963117,0.631683512738392));
#7337=CARTESIAN_POINT('Ctrl Pts',(10.0735011273457,6.98640902740309,2.67084202324935));
#7338=CARTESIAN_POINT('Ctrl Pts',(10.1999704101463,4.30075500530173,2.28447659290827));
#7339=CARTESIAN_POINT('Ctrl Pts',(10.3264396929469,3.15844865589028,-0.176338518429553));
#7340=CARTESIAN_POINT('Ctrl Pts',(10.4529089757475,4.59619094607847,-2.47727672964101));
#7341=CARTESIAN_POINT('Ctrl Pts',(10.579378258548,7.30958651281973,-2.52804507698133));
#7342=CARTESIAN_POINT('Ctrl Pts',(10.7058475413486,8.83213959996092,-0.283992081323606));
#7343=CARTESIAN_POINT('Ctrl Pts',(10.8323168241492,7.78581226518845,2.21979841478548));
#7344=CARTESIAN_POINT('Ctrl Pts',(10.9587861069498,5.11161821006357,2.70412071413346));
#7345=CARTESIAN_POINT('Ctrl Pts',(11.0430989621501,3.87611344666481,1.39513483291862));
#7346=CARTESIAN_POINT('Ctrl Pts',(11.0852553897503,3.66965311083307,0.623566746436274));
#7347=CARTESIAN_POINT('Ctrl Pts',(-0.255766169251004,4.04109127178312,1.64811304057572));
#7348=CARTESIAN_POINT('Ctrl Pts',(-0.213609741650813,3.49540795273091,0.999526572161923));
#7349=CARTESIAN_POINT('Ctrl Pts',(-0.129296886450431,3.10772445821582,-0.870876870782859));
#7350=CARTESIAN_POINT('Ctrl Pts',(-0.00282760364985834,5.15450976265528,
-2.9027366727603));
#7351=CARTESIAN_POINT('Ctrl Pts',(0.123641679150715,7.96852586228423,-2.29102325178121));
#7352=CARTESIAN_POINT('Ctrl Pts',(0.250110961951288,8.99513403173513,0.397450258620327));
#7353=CARTESIAN_POINT('Ctrl Pts',(0.376580244751861,7.30166397004841,2.72694193252232));
#7354=CARTESIAN_POINT('Ctrl Pts',(0.503049527552434,4.42618944743245,2.57901724514726));
#7355=CARTESIAN_POINT('Ctrl Pts',(0.629518810353006,2.97989373731284,0.0895594277083228));
#7356=CARTESIAN_POINT('Ctrl Pts',(0.755988093153581,4.27624391707079,-2.48150710395807));
#7357=CARTESIAN_POINT('Ctrl Pts',(0.882457375954154,7.13796708616038,-2.79891497944178));
#7358=CARTESIAN_POINT('Ctrl Pts',(1.00892665875473,8.96628117760225,-0.574639774076433));
#7359=CARTESIAN_POINT('Ctrl Pts',(1.1353959415553,8.10084469393023,2.17151861507739));
#7360=CARTESIAN_POINT('Ctrl Pts',(1.26186522435587,5.32758429305789,2.94565042609802));
#7361=CARTESIAN_POINT('Ctrl Pts',(1.38833450715645,3.16495931797173,1.0447803202184));
#7362=CARTESIAN_POINT('Ctrl Pts',(1.51480378995702,3.57690019914092,-1.80488441711536));
#7363=CARTESIAN_POINT('Ctrl Pts',(1.64127307275759,6.18931341035722,-3.01548925232429));
#7364=CARTESIAN_POINT('Ctrl Pts',(1.76774235555816,8.62980687076538,-1.48766065606638));
#7365=CARTESIAN_POINT('Ctrl Pts',(1.89421163835874,8.68211232342893,1.39114751979702));
#7366=CARTESIAN_POINT('Ctrl Pts',(2.02068092115931,6.29873006674212,3.00662229441761));
#7367=CARTESIAN_POINT('Ctrl Pts',(2.14715020395988,3.6440641683139,1.89171460246179));
#7368=CARTESIAN_POINT('Ctrl Pts',(2.27361948676046,3.12887765854667,-0.941102636765302));
#7369=CARTESIAN_POINT('Ctrl Pts',(2.40008876956103,5.221023215509,-2.91928291965494));
#7370=CARTESIAN_POINT('Ctrl Pts',(2.5265580523616,8.02057546463636,-2.24639543728625));
#7371=CARTESIAN_POINT('Ctrl Pts',(2.65302733516218,8.98519677504537,0.466495297308555));
#7372=CARTESIAN_POINT('Ctrl Pts',(2.77949661796275,7.23889240500353,2.75575094100713));
#7373=CARTESIAN_POINT('Ctrl Pts',(2.90596590076332,4.36752141768572,2.5424459342591));
#7374=CARTESIAN_POINT('Ctrl Pts',(3.0324351835639,2.97864168519721,0.0202874407439004));
#7375=CARTESIAN_POINT('Ctrl Pts',(3.15890446636446,4.33352675754921,-2.52029454194393));
#7376=CARTESIAN_POINT('Ctrl Pts',(3.28537374916504,7.20177441543159,-2.77213922842707));
#7377=CARTESIAN_POINT('Ctrl Pts',(3.41184303196561,8.97866315423926,-0.506540679845794));
#7378=CARTESIAN_POINT('Ctrl Pts',(3.53831231476619,8.05055954300406,2.21905908152931));
#7379=CARTESIAN_POINT('Ctrl Pts',(3.66478159756676,5.26029576462132,2.92948037902181));
#7380=CARTESIAN_POINT('Ctrl Pts',(3.79125088036734,3.14177437347817,0.979573332991449));
#7381=CARTESIAN_POINT('Ctrl Pts',(3.9177201631679,3.61887325026032,-1.85990673112716));
#7382=CARTESIAN_POINT('Ctrl Pts',(4.04418944596849,6.25832795884948,-3.01036282074418));
#7383=CARTESIAN_POINT('Ctrl Pts',(4.17065872876905,8.66318912116946,-1.42703936585924));
#7384=CARTESIAN_POINT('Ctrl Pts',(4.29712801156963,8.64954714081024,1.45221127782889));
#7385=CARTESIAN_POINT('Ctrl Pts',(4.42359729437019,6.22979061312465,3.01267554193145));
#7386=CARTESIAN_POINT('Ctrl Pts',(4.55006657717078,3.60135595755754,1.83726002636678));
#7387=CARTESIAN_POINT('Ctrl Pts',(4.67653585997134,3.1511849892005,-1.00661347153406));
#7388=CARTESIAN_POINT('Ctrl Pts',(4.80300514277192,5.28808829272449,-2.93635818112757));
#7389=CARTESIAN_POINT('Ctrl Pts',(4.92947442557249,8.07149495106845,-2.19952865735556));
#7390=CARTESIAN_POINT('Ctrl Pts',(5.05594370837307,8.9737295178849,0.534743304110009));
#7391=CARTESIAN_POINT('Ctrl Pts',(5.18241299117364,7.17545208301331,2.78340260245806));
#7392=CARTESIAN_POINT('Ctrl Pts',(5.30888227397421,4.30971964307301,2.50439013770165));
#7393=CARTESIAN_POINT('Ctrl Pts',(5.43535155677478,2.97896957548569,-0.0489164695102037));
#7394=CARTESIAN_POINT('Ctrl Pts',(5.56182083957536,4.39168654812479,-2.55780090846567));
#7395=CARTESIAN_POINT('Ctrl Pts',(5.68829012237593,7.26494986606656,-2.74388765862757));
#7396=CARTESIAN_POINT('Ctrl Pts',(5.81475940517651,8.98948318879469,-0.438187072771831));
#7397=CARTESIAN_POINT('Ctrl Pts',(5.94122868797707,7.99919823984401,2.26544124722655));
#7398=CARTESIAN_POINT('Ctrl Pts',(6.06769797077765,5.19339550153742,2.91177039443194));
#7399=CARTESIAN_POINT('Ctrl Pts',(6.19416725357823,3.12008881427174,0.913854041489789));
#7400=CARTESIAN_POINT('Ctrl Pts',(6.32063653637879,3.66209554878131,-1.91395413315054));
#7401=CARTESIAN_POINT('Ctrl Pts',(6.44710581917937,6.32720695415856,-3.00365664748478));
#7402=CARTESIAN_POINT('Ctrl Pts',(6.57357510197995,8.69517421732942,-1.3656696471219));
#7403=CARTESIAN_POINT('Ctrl Pts',(6.70004438478051,8.61559193816459,1.51251329245416));
#7404=CARTESIAN_POINT('Ctrl Pts',(6.8265136675811,6.16073061022695,3.01714820944448));
#7405=CARTESIAN_POINT('Ctrl Pts',(6.95298295038165,3.55990612749904,1.78184161478998));
#7406=CARTESIAN_POINT('Ctrl Pts',(7.07945223318224,3.17498687362254,-1.07159623119251));
#7407=CARTESIAN_POINT('Ctrl Pts',(7.2059215159828,5.35552685433585,-2.95189295389255));
#7408=CARTESIAN_POINT('Ctrl Pts',(7.33239079878339,8.12132768474379,-2.15150795971123));
#7409=CARTESIAN_POINT('Ctrl Pts',(7.45886008158395,8.96070217500711,0.602710774981116));
#7410=CARTESIAN_POINT('Ctrl Pts',(7.58532936438453,7.11139509225075,2.80959402670167));
#7411=CARTESIAN_POINT('Ctrl Pts',(7.71179864718509,4.25280462794925,2.46502048238232));
#7412=CARTESIAN_POINT('Ctrl Pts',(7.83826792998568,2.98088236599169,-0.118094717771357));
#7413=CARTESIAN_POINT('Ctrl Pts',(7.96473721278624,4.45069009732305,-2.59396539404523));
#7414=CARTESIAN_POINT('Ctrl Pts',(8.09120649558682,7.32746169336768,-2.71419658477305));
#7415=CARTESIAN_POINT('Ctrl Pts',(8.2176757783874,8.99873487696146,-0.369603580401957));
#7416=CARTESIAN_POINT('Ctrl Pts',(8.34414506118796,7.9467881045264,2.31063490665217));
#7417=CARTESIAN_POINT('Ctrl Pts',(8.47061434398854,5.12691841598226,2.89253283821776));
#7418=CARTESIAN_POINT('Ctrl Pts',(8.59708362678912,3.09991409354922,0.847655304587422));
#7419=CARTESIAN_POINT('Ctrl Pts',(8.72355290958968,3.70654441823305,-1.96699739921706));
#7420=CARTESIAN_POINT('Ctrl Pts',(8.85002219239026,6.39591418697016,-2.99537475015773));
#7421=CARTESIAN_POINT('Ctrl Pts',(8.97649147519083,8.72574556011418,-1.30358334856292));
#7422=CARTESIAN_POINT('Ctrl Pts',(9.1029607579914,8.58026416208568,1.57202158130248));
#7423=CARTESIAN_POINT('Ctrl Pts',(9.22943004079197,6.09158700182589,3.02003844763038));
#7424=CARTESIAN_POINT('Ctrl Pts',(9.35589932359257,3.51973505278771,1.72548757686079));
#7425=CARTESIAN_POINT('Ctrl Pts',(9.48236860639312,3.20027345136559,-1.1360152149446));
#7426=CARTESIAN_POINT('Ctrl Pts',(9.6088378891937,5.42329849222802,-2.96588214441775));
#7427=CARTESIAN_POINT('Ctrl Pts',(9.73530717199428,8.17005714643252,-2.10235270013504));
#7428=CARTESIAN_POINT('Ctrl Pts',(9.86177645479484,8.94610316147124,0.670350888189973));
#7429=CARTESIAN_POINT('Ctrl Pts',(9.98824573759542,7.04679029023846,2.83433283661117));
#7430=CARTESIAN_POINT('Ctrl Pts',(10.114715020396,4.19673876478062,2.42431673808699));
#7431=CARTESIAN_POINT('Ctrl Pts',(10.2411843031966,2.98450817703985,-0.187132765170506));
#7432=CARTESIAN_POINT('Ctrl Pts',(10.3676535859971,4.51025928781023,-2.62891879005706));
#7433=CARTESIAN_POINT('Ctrl Pts',(10.4941228687977,7.38975050690281,-2.68279483089907));
#7434=CARTESIAN_POINT('Ctrl Pts',(10.6205921515983,9.0055039557413,-0.301376148205788));
#7435=CARTESIAN_POINT('Ctrl Pts',(10.7470614343989,7.895127566208,2.35567940107123));
#7436=CARTESIAN_POINT('Ctrl Pts',(10.8735307171994,5.05723750909054,2.86964862298535));
#7437=CARTESIAN_POINT('Ctrl Pts',(10.9578435723998,3.7461035332853,1.48053551427594));
#7438=CARTESIAN_POINT('Ctrl Pts',(11.,3.52700509758159,0.661737268568548));
#7439=CARTESIAN_POINT('Ctrl Pts',(-2.77555756156289E-16,4.38007430561128,
1.36291222925734));
#7440=CARTESIAN_POINT('Ctrl Pts',(-2.80031029468505E-16,4.32659445095465,
1.31130786139469));
#7441=CARTESIAN_POINT('Ctrl Pts',(1.11194639968977E-16,4.27624355628285,
1.25685426489337));
#7442=CARTESIAN_POINT('Ctrl Pts',(4.68375338513738E-17,4.22901660607647,
1.19991824488684));
#7443=CARTESIAN_POINT('Ctrl Pts',(-1.93070425417206E-17,4.18047796280637,
1.14140086969662));
#7444=CARTESIAN_POINT('Ctrl Pts',(-1.48725298511017E-16,4.13523875300555,
1.08026078916569));
#7445=CARTESIAN_POINT('Ctrl Pts',(-1.66533453693773E-16,4.09332060715764,
1.01684861703025));
#7446=CARTESIAN_POINT('Ctrl Pts',(-1.8377727982304E-16,4.05273082055456,
0.955445936092179));
#7447=CARTESIAN_POINT('Ctrl Pts',(-3.01042658861766E-16,4.01525479286761,
0.891912050008348));
#7448=CARTESIAN_POINT('Ctrl Pts',(-3.33066907387547E-16,3.98094125132206,
0.826531654328836));
#7449=CARTESIAN_POINT('Ctrl Pts',(-3.47077516117576E-16,3.96592907689589,
0.79792773121905));
#7450=CARTESIAN_POINT('Ctrl Pts',(-1.42842800960507E-16,3.95152261862076,
0.768970004663094));
#7451=CARTESIAN_POINT('Ctrl Pts',(-1.45716771982052E-16,3.9377279101113,
0.739680798967653));
#7452=CARTESIAN_POINT('Ctrl Pts',(-1.47637449172231E-16,3.9285088951036,
0.720106798786031));
#7453=CARTESIAN_POINT('Ctrl Pts',(-1.72992178300136E-16,3.91956312859518,
0.700384733783148));
#7454=CARTESIAN_POINT('Ctrl Pts',(-1.73472347597681E-16,3.91089273167378,
0.680521086833724));
#7455=CARTESIAN_POINT('Ctrl Pts',(-1.73770300656856E-16,3.90551260574693,
0.668195362541848));
#7456=CARTESIAN_POINT('Ctrl Pts',(2.06740054808053E-16,3.90024214212162,
0.655823365037683));
#7457=CARTESIAN_POINT('Ctrl Pts',(2.0122792321331E-16,3.89508319856995,
0.643411203636316));
#7458=CARTESIAN_POINT('Ctrl Pts',(1.68366422301827E-16,3.86432728766482,
0.569414012859255));
#7459=CARTESIAN_POINT('Ctrl Pts',(-4.84275148589556E-16,3.83751112678279,
0.493944650744559));
#7460=CARTESIAN_POINT('Ctrl Pts',(-3.60822483003176E-16,3.81465926753848,
0.417382612231489));
#7461=CARTESIAN_POINT('Ctrl Pts',(-2.35429102250813E-16,3.79144816979904,
0.339616994123154));
#7462=CARTESIAN_POINT('Ctrl Pts',(-1.12344122363624E-16,3.77232649682797,
0.260723255358029));
#7463=CARTESIAN_POINT('Ctrl Pts',(-5.55111512312578E-17,3.75736079522538,
0.181064368578248));
#7464=CARTESIAN_POINT('Ctrl Pts',(-4.96349244774822E-18,3.74405019113428,
0.11021517403868));
#7465=CARTESIAN_POINT('Ctrl Pts',(-2.69294374879976E-16,3.73402751903509,
0.0387597845660613));
#7466=CARTESIAN_POINT('Ctrl Pts',(-2.63677968348475E-16,3.72737085088334,
-0.0330606627948158));
#7467=CARTESIAN_POINT('Ctrl Pts',(-2.6150366267442E-16,3.72479382387301,
-0.0608648477899769));
#7468=CARTESIAN_POINT('Ctrl Pts',(8.93900777674783E-17,3.7227216032029,
-0.0887238419963498));
#7469=CARTESIAN_POINT('Ctrl Pts',(1.38777878078145E-16,3.72116002426916,
-0.116623918592605));
#7470=CARTESIAN_POINT('Ctrl Pts',(1.66233930557089E-16,3.72029189908672,
-0.132134347532035));
#7471=CARTESIAN_POINT('Ctrl Pts',(2.59188299389654E-16,3.71958160408319,
-0.147657474843062));
#7472=CARTESIAN_POINT('Ctrl Pts',(2.63677968348475E-16,3.71903024499337,
-0.163190949016707));
#7473=CARTESIAN_POINT('Ctrl Pts',(2.67507061918538E-16,3.71856000864298,
-0.17643894717082));
#7474=CARTESIAN_POINT('Ctrl Pts',(-1.23245947320793E-16,3.71820570920862,
-0.189685934650389));
#7475=CARTESIAN_POINT('Ctrl Pts',(-1.11022302462516E-16,3.71796762862309,
-0.20292615382453));
#7476=CARTESIAN_POINT('Ctrl Pts',(-3.40061438085201E-17,3.71646758077648,
-0.286347329124692));
#7477=CARTESIAN_POINT('Ctrl Pts',(9.27905525951754E-17,3.71957542118597,
-0.369551234359023));
#7478=CARTESIAN_POINT('Ctrl Pts',(0.,3.72735027744889,-0.45215857472717));
#7479=CARTESIAN_POINT('Ctrl Pts',(-8.48558343440982E-17,3.73446028915422,
-0.527701985061926));
#7480=CARTESIAN_POINT('Ctrl Pts',(-2.70767289408761E-16,3.74547354769541,
-0.60274741009298));
#7481=CARTESIAN_POINT('Ctrl Pts',(-2.77555756156289E-16,3.76047169010912,
-0.677016215888271));
#7482=CARTESIAN_POINT('Ctrl Pts',(-2.865998411998E-16,3.77645697580371,
-0.756173223875352));
#7483=CARTESIAN_POINT('Ctrl Pts',(-1.65629045189422E-16,3.79696805372881,
-0.834448848484121));
#7484=CARTESIAN_POINT('Ctrl Pts',(-1.66533453693773E-16,3.82173963045682,
-0.911614883986038));
#7485=CARTESIAN_POINT('Ctrl Pts',(-1.6687918879021E-16,3.83120924891766,
-0.94111372947183));
#7486=CARTESIAN_POINT('Ctrl Pts',(-4.07690256823517E-16,3.84130202564309,
-0.970450366187668));
#7487=CARTESIAN_POINT('Ctrl Pts',(-4.16333634234434E-16,3.85200508769203,
-0.999611703631864));
#7488=CARTESIAN_POINT('Ctrl Pts',(-4.20262745966492E-16,3.8568704921128,
-1.0128678820477));
#7489=CARTESIAN_POINT('Ctrl Pts',(-5.1383979233867E-16,3.86186202208545,
-1.02608783230357));
#7490=CARTESIAN_POINT('Ctrl Pts',(-5.27355936696949E-16,3.86697853716836,
-1.03927030385677));
#7491=CARTESIAN_POINT('Ctrl Pts',(-5.3932641475938E-16,3.87150994271808,
-1.0509452669493));
#7492=CARTESIAN_POINT('Ctrl Pts',(1.87412194500338E-16,3.87613799774593,
-1.06258713958298));
#7493=CARTESIAN_POINT('Ctrl Pts',(1.66533453693773E-16,3.88085844924797,
-1.07418734184327));
#7494=CARTESIAN_POINT('Ctrl Pts',(2.64154277135885E-17,3.91253757934153,
-1.15203674170612));
#7495=CARTESIAN_POINT('Ctrl Pts',(1.31044853828581E-16,3.9484137341162,
-1.22811404869558));
#7496=CARTESIAN_POINT('Ctrl Pts',(-2.77555756156289E-17,3.98814410668546,
-1.3021798603163));
#7497=CARTESIAN_POINT('Ctrl Pts',(-1.88358197049143E-16,4.0283253707254,
-1.37708622893583));
#7498=CARTESIAN_POINT('Ctrl Pts',(-5.21101545420775E-16,4.07244924500996,
-1.44993596567706));
#7499=CARTESIAN_POINT('Ctrl Pts',(-5.55111512312578E-16,4.12021737446078,
-1.5204760132583));
#7500=CARTESIAN_POINT('Ctrl Pts',(-5.89453236598535E-16,4.16845146820379,
-1.59170415860933));
#7501=CARTESIAN_POINT('Ctrl Pts',(-9.73015521435432E-17,4.22040173027164,
-1.66057819124318));
#7502=CARTESIAN_POINT('Ctrl Pts',(0.,4.27581129957554,-1.72681968984969));
#7503=CARTESIAN_POINT('Ctrl Pts',(3.97348772770828E-17,4.29843881566099,
-1.75387062336303));
#7504=CARTESIAN_POINT('Ctrl Pts',(-1.6663043826359E-16,4.32164376063082,
-1.78048226411648));
#7505=CARTESIAN_POINT('Ctrl Pts',(-1.94289029309402E-16,4.34541073537425,
-1.8066342869413));
#7506=CARTESIAN_POINT('Ctrl Pts',(-2.11417038683516E-16,4.36012880129184,
-1.82282933069294));
#7507=CARTESIAN_POINT('Ctrl Pts',(-6.39101957865414E-16,4.37506710170624,
-1.83885279980293));
#7508=CARTESIAN_POINT('Ctrl Pts',(-6.38378239159465E-16,4.39019735919426,
-1.85467428809663));
#7509=CARTESIAN_POINT('Ctrl Pts',(-6.35371199708122E-16,4.45306333295106,
-1.92041231460757));
#7510=CARTESIAN_POINT('Ctrl Pts',(-2.58129078341152E-16,4.51929547534557,
-1.98273176066174));
#7511=CARTESIAN_POINT('Ctrl Pts',(-2.22044604925031E-16,4.58856873157643,
-2.04132864721816));
#7512=CARTESIAN_POINT('Ctrl Pts',(-1.94981249862941E-16,4.64052367374958,
-2.08527631213548));
#7513=CARTESIAN_POINT('Ctrl Pts',(-4.23851232862792E-16,4.69419050378083,
-2.12712976418203));
#7514=CARTESIAN_POINT('Ctrl Pts',(-4.16333634234434E-16,4.74945005246149,
-2.16674908321904));
#7515=CARTESIAN_POINT('Ctrl Pts',(-4.13731776004568E-16,4.7685755097546,
-2.18046142094738));
#7516=CARTESIAN_POINT('Ctrl Pts',(-2.52486346214463E-16,4.78789187530008,
-2.19390603143607));
#7517=CARTESIAN_POINT('Ctrl Pts',(-2.22044604925031E-16,4.80739457519056,
-2.20707674403954));
#7518=CARTESIAN_POINT('Ctrl Pts',(-1.97425656185765E-16,4.82316686509724,
-2.21772820761258));
#7519=CARTESIAN_POINT('Ctrl Pts',(-3.9339803241751E-16,4.83905374993306,
-2.22819555975246));
#7520=CARTESIAN_POINT('Ctrl Pts',(-4.16333634234434E-16,4.85504755554653,
-2.23847288314367));
#7521=CARTESIAN_POINT('Ctrl Pts',(-5.23613684113935E-16,4.92985772524132,
-2.28654451321636));
#7522=CARTESIAN_POINT('Ctrl Pts',(-8.0505927221409E-17,5.00703712827284,
-2.33048359411215));
#7523=CARTESIAN_POINT('Ctrl Pts',(1.66533453693773E-16,5.08631071040055,
-2.36999470778006));
#7524=CARTESIAN_POINT('Ctrl Pts',(3.67447598235833E-16,5.15078295720981,
-2.40212861927662));
#7525=CARTESIAN_POINT('Ctrl Pts',(6.09938800167838E-17,5.21664131547317,
-2.43133339556246));
#7526=CARTESIAN_POINT('Ctrl Pts',(1.11022302462516E-16,5.28375444250491,
-2.45743079686607));
#7527=CARTESIAN_POINT('Ctrl Pts',(1.24376244097105E-16,5.30138663960587,
-2.46428719804956));
#7528=CARTESIAN_POINT('Ctrl Pts',(-7.67588771122088E-18,5.31910551399007,
-2.47092900830453));
#7529=CARTESIAN_POINT('Ctrl Pts',(0.,5.33690753016716,-2.47735729053333));
#7530=CARTESIAN_POINT('Ctrl Pts',(1.2890562790225,8.11784406625472,-0.00180833638339553));
#7531=CARTESIAN_POINT('Ctrl Pts',(1.28093512868358,8.11906067093066,-0.136660465564393));
#7532=CARTESIAN_POINT('Ctrl Pts',(1.27281397834465,8.10727342448819,-0.271300590561459));
#7533=CARTESIAN_POINT('Ctrl Pts',(1.26469282800573,8.0817079134367,-0.403271335301992));
#7534=CARTESIAN_POINT('Ctrl Pts',(1.22253640040554,7.94899880564707,-1.0883239342341));
#7535=CARTESIAN_POINT('Ctrl Pts',(1.18037997280535,7.44502212184727,-1.70144771154639));
#7536=CARTESIAN_POINT('Ctrl Pts',(1.13822354520516,6.79861529368678,-1.9642626944474));
#7537=CARTESIAN_POINT('Ctrl Pts',(1.09606711760497,6.15220846552629,-2.2270776773484));
#7538=CARTESIAN_POINT('Ctrl Pts',(1.05391069000478,5.36337149300511,-2.13958386583811));
#7539=CARTESIAN_POINT('Ctrl Pts',(1.01175426240458,4.790282868037,-1.7414783762589));
#7540=CARTESIAN_POINT('Ctrl Pts',(0.969597834804393,4.21719424306888,-1.34337288667968));
#7541=CARTESIAN_POINT('Ctrl Pts',(0.927441407204202,3.85985396565383,-0.634655719031535));
#7542=CARTESIAN_POINT('Ctrl Pts',(0.885284979604011,3.88052028647255,0.0628136850736727));
#7543=CARTESIAN_POINT('Ctrl Pts',(0.84312855200382,3.90118660729128,0.76028308917888));
#7544=CARTESIAN_POINT('Ctrl Pts',(0.800972124403629,4.29985952634379,1.44650472974115));
#7545=CARTESIAN_POINT('Ctrl Pts',(0.758815696803438,4.89550975959257,1.81000334710386));
#7546=CARTESIAN_POINT('Ctrl Pts',(0.716659269203247,5.49115999284134,2.17350196446658));
#7547=CARTESIAN_POINT('Ctrl Pts',(0.674502841603056,6.28378754028639,2.21427755862973));
#7548=CARTESIAN_POINT('Ctrl Pts',(0.632346414002865,6.91350470727655,1.91360195247884));
#7549=CARTESIAN_POINT('Ctrl Pts',(0.590189986402674,7.5432218742667,1.61292634632796));
#7550=CARTESIAN_POINT('Ctrl Pts',(0.548033558802482,8.01002866080195,0.970799539863048));
#7551=CARTESIAN_POINT('Ctrl Pts',(0.505877131202291,8.10193924842326,0.279195874812881));
#7552=CARTESIAN_POINT('Ctrl Pts',(0.500270180475694,8.11416367457561,0.187210194502225));
#7553=CARTESIAN_POINT('Ctrl Pts',(0.494663229749096,8.11975621683434,0.094349272504648));
#7554=CARTESIAN_POINT('Ctrl Pts',(0.489056279022499,8.11901932033641,0.00140296810865748));
#7555=CARTESIAN_POINT('Ctrl Pts',(0.,6.66173726856851,-2.47299490241842));
#7556=CARTESIAN_POINT('Ctrl Pts',(0.042156427600191,7.4805355142759,-2.25389646671472));
#7557=CARTESIAN_POINT('Ctrl Pts',(0.126469282800573,8.86964786268114,-0.942757917500329));
#7558=CARTESIAN_POINT('Ctrl Pts',(0.252938565601146,8.35568007480496,1.89512494763008));
#7559=CARTESIAN_POINT('Ctrl Pts',(0.379407848401719,5.69862372086684,3.00550592532682));
#7560=CARTESIAN_POINT('Ctrl Pts',(0.505877131202292,3.31720488565003,1.38974961778526));
#7561=CARTESIAN_POINT('Ctrl Pts',(0.632346414002866,3.37108102552373,-1.4897402431435));
#7562=CARTESIAN_POINT('Ctrl Pts',(0.758815696803437,5.81286715979806,-3.01549246530217));
#7563=CARTESIAN_POINT('Ctrl Pts',(0.885284979604013,8.42431700898103,-1.80326119610285));
#7564=CARTESIAN_POINT('Ctrl Pts',(1.01175426240458,8.83433307398675,1.04679026852714));
#7565=CARTESIAN_POINT('Ctrl Pts',(1.13822354520516,6.67035096999308,2.94610350710691));
#7566=CARTESIAN_POINT('Ctrl Pts',(1.26469282800573,3.89764709051462,2.17005731163833));
#7567=CARTESIAN_POINT('Ctrl Pts',(1.39116211080631,3.0341175837159,-0.576701540113256));
#7568=CARTESIAN_POINT('Ctrl Pts',(1.51763139360688,4.8639846740404,-2.79972682418719));
#7569=CARTESIAN_POINT('Ctrl Pts',(1.64410067640745,7.72548774157445,-2.48026517361596));
#7570=CARTESIAN_POINT('Ctrl Pts',(1.77056995920802,9.02003873021916,0.0915870066384873));
#7571=CARTESIAN_POINT('Ctrl Pts',(1.89703924200859,7.57202172994746,2.58026440683785));
#7572=CARTESIAN_POINT('Ctrl Pts',(2.02350852480917,4.69641652838636,2.72574581528328));
#7573=CARTESIAN_POINT('Ctrl Pts',(2.14997780760974,3.00462496841716,0.395914224840739));
#7574=CARTESIAN_POINT('Ctrl Pts',(2.27644709041032,4.03300241565958,-2.29345579779455));
#7575=CARTESIAN_POINT('Ctrl Pts',(2.40291637321088,6.8476553843829,-2.90008617898366));
#7576=CARTESIAN_POINT('Ctrl Pts',(2.52938565601147,8.89253311018671,-0.873081666227454));
#7577=CARTESIAN_POINT('Ctrl Pts',(2.65585493881203,8.31063512397009,1.94678828765999));
#7578=CARTESIAN_POINT('Ctrl Pts',(2.78232422161261,5.63039638482652,2.99873515893208));
#7579=CARTESIAN_POINT('Ctrl Pts',(2.90879350441318,3.28580315999094,1.32746181821946));
#7580=CARTESIAN_POINT('Ctrl Pts',(3.03526278721375,3.4060343620134,-1.54931004838359));
#7581=CARTESIAN_POINT('Ctrl Pts',(3.16173207001433,5.88190527112525,-3.01911791792189));
#7582=CARTESIAN_POINT('Ctrl Pts',(3.2882013528149,8.46502071419216,-1.74719553636016));
#7583=CARTESIAN_POINT('Ctrl Pts',(3.41467063561548,8.80959429091728,1.11139519676803));
#7584=CARTESIAN_POINT('Ctrl Pts',(3.54113991841604,6.60271083165986,2.96070245343145));
#7585=CARTESIAN_POINT('Ctrl Pts',(3.66760920121663,3.84849183796069,2.12132788423443));
#7586=CARTESIAN_POINT('Ctrl Pts',(3.79407848401719,3.0481067685106,-0.644473206270731));
#7587=CARTESIAN_POINT('Ctrl Pts',(3.92054776681777,4.92840366803431,-2.82501339204223));
#7588=CARTESIAN_POINT('Ctrl Pts',(4.04701704961833,7.78184178235469,-2.4400941019681));
#7589=CARTESIAN_POINT('Ctrl Pts',(4.17348633241892,9.01714849317786,0.160730625342051));
#7590=CARTESIAN_POINT('Ctrl Pts',(4.29995561521948,7.51251343469132,2.61559218413545));
#7591=CARTESIAN_POINT('Ctrl Pts',(4.42642489802006,4.63433022445025,2.69517447078429));
#7592=CARTESIAN_POINT('Ctrl Pts',(4.55289418082063,2.99634307005063,0.327206984929225));
#7593=CARTESIAN_POINT('Ctrl Pts',(4.6793634636212,4.08604568686072,-2.33790467107576));
#7594=CARTESIAN_POINT('Ctrl Pts',(4.80583274642178,6.91385412742878,-2.87991145655582));
#7595=CARTESIAN_POINT('Ctrl Pts',(4.93230202922234,8.91177066825553,-0.806604574315915));
#7596=CARTESIAN_POINT('Ctrl Pts',(5.05877131202293,8.26544146026922,1.99919842784905));
#7597=CARTESIAN_POINT('Ctrl Pts',(5.18524059482349,5.56181288602103,2.98948346992642));
#7598=CARTESIAN_POINT('Ctrl Pts',(5.31170987762408,3.2561120833366,1.26494998502281));
#7599=CARTESIAN_POINT('Ctrl Pts',(5.43817916042463,3.44219885099807,-1.60831360312132));
#7600=CARTESIAN_POINT('Ctrl Pts',(5.56464844322522,5.9510835258896,-3.02103070861275));
#7601=CARTESIAN_POINT('Ctrl Pts',(5.69111772602578,8.50439037321506,-1.69028051588142));
#7602=CARTESIAN_POINT('Ctrl Pts',(5.81758700882636,8.78340286420995,1.17545219355302));
#7603=CARTESIAN_POINT('Ctrl Pts',(5.94405629162693,6.53474335439746,2.97372979753514));
#7604=CARTESIAN_POINT('Ctrl Pts',(6.07052557442751,3.80047113580028,2.07149514587238));
#7605=CARTESIAN_POINT('Ctrl Pts',(6.19699485722809,3.06364154273657,-0.711911774223792));
#7606=CARTESIAN_POINT('Ctrl Pts',(6.32346414002865,4.99338643380372,-2.84881527870274));
#7607=CARTESIAN_POINT('Ctrl Pts',(6.44993342282923,7.83726019914311,-2.39864426801156));
#7608=CARTESIAN_POINT('Ctrl Pts',(6.5764027056298,9.01267582524419,0.229790634734156));
#7609=CARTESIAN_POINT('Ctrl Pts',(6.70287198843037,7.45221141439524,2.64954738997428));
#7610=CARTESIAN_POINT('Ctrl Pts',(6.82934127123096,4.57296049994168,2.66318937161644));
#7611=CARTESIAN_POINT('Ctrl Pts',(6.95581055403151,2.9896368961606,0.258327983142764));
#7612=CARTESIAN_POINT('Ctrl Pts',(7.0822798368321,4.14009309396666,-2.38112697366136));
#7613=CARTESIAN_POINT('Ctrl Pts',(7.20874911963266,6.97957342511075,-2.8582258953101));
#7614=CARTESIAN_POINT('Ctrl Pts',(7.33521840243324,8.92948065451071,-0.739704304940699));
#7615=CARTESIAN_POINT('Ctrl Pts',(7.46168768523381,8.21905929021046,2.05055973583909));
#7616=CARTESIAN_POINT('Ctrl Pts',(7.58815696803438,5.49345927251859,2.97866343435355));
#7617=CARTESIAN_POINT('Ctrl Pts',(7.71462625083496,3.22786051088117,1.20177452844665));
#7618=CARTESIAN_POINT('Ctrl Pts',(7.84109553363553,3.47970522104534,-1.66647339916602));
#7619=CARTESIAN_POINT('Ctrl Pts',(7.96756481643612,6.02028744265461,-3.02135859893257));
#7620=CARTESIAN_POINT('Ctrl Pts',(8.09403409923666,8.54244617334588,-1.63247873583206));
#7621=CARTESIAN_POINT('Ctrl Pts',(8.22050338203726,8.75575120016859,1.23889252150743));
#7622=CARTESIAN_POINT('Ctrl Pts',(8.34697266483782,6.46649534115966,2.98519705577739));
#7623=CARTESIAN_POINT('Ctrl Pts',(8.4734419476384,3.75360435149572,2.02057565464541));
#7624=CARTESIAN_POINT('Ctrl Pts',(8.59991123043897,3.08071680575365,-0.778976857734081));
#7625=CARTESIAN_POINT('Ctrl Pts',(8.72638051323954,5.05889727484518,-2.87112261147709));
#7626=CARTESIAN_POINT('Ctrl Pts',(8.85284979604013,7.89171478015486,-2.35593605319605));
#7627=CARTESIAN_POINT('Ctrl Pts',(8.97931907884068,9.00662257753226,0.298730094753956));
#7628=CARTESIAN_POINT('Ctrl Pts',(9.10578836164127,7.39114764994812,2.68211257580753));
#7629=CARTESIAN_POINT('Ctrl Pts',(9.23225764444183,4.51233920524947,2.62980711778656));
#7630=CARTESIAN_POINT('Ctrl Pts',(9.35872692724241,2.98451046190918,0.189313428699894));
#7631=CARTESIAN_POINT('Ctrl Pts',(9.48519621004298,4.19511541707917,-2.42310002974361));
#7632=CARTESIAN_POINT('Ctrl Pts',(9.61166549284355,7.04478041145962,-2.83504094672479));
#7633=CARTESIAN_POINT('Ctrl Pts',(9.73813477564413,8.94565071555854,-0.672415773772391));
#7634=CARTESIAN_POINT('Ctrl Pts',(9.8646040584447,8.17151879730683,2.10084489825768));
#7635=CARTESIAN_POINT('Ctrl Pts',(9.99107334124527,5.42536021041376,2.96628144383517));
#7636=CARTESIAN_POINT('Ctrl Pts',(10.1175426240458,3.20108469038192,1.13796721707783));
#7637=CARTESIAN_POINT('Ctrl Pts',(10.2440119068464,3.51849277787554,-1.72375628994429));
#7638=CARTESIAN_POINT('Ctrl Pts',(10.370481189647,6.08955924048204,-3.02010646233692));
#7639=CARTESIAN_POINT('Ctrl Pts',(10.4969504724476,8.57901781465834,-1.57381085898247));
#7640=CARTESIAN_POINT('Ctrl Pts',(10.6234197552481,8.72694165367111,1.30166438987783));
#7641=CARTESIAN_POINT('Ctrl Pts',(10.7498890380487,6.39745114979413,2.99513375481657));
#7642=CARTESIAN_POINT('Ctrl Pts',(10.8763583208493,3.70897520872018,1.96852709774085));
#7643=CARTESIAN_POINT('Ctrl Pts',(11.0028276036499,3.0972650878174,-0.845492289473616));
#7644=CARTESIAN_POINT('Ctrl Pts',(11.1292968864504,5.12911981582823,-2.89227229900937));
#7645=CARTESIAN_POINT('Ctrl Pts',(11.2136097416508,6.99952657216188,-2.50459204726911));
#7646=CARTESIAN_POINT('Ctrl Pts',(11.255766169251,7.64811304057568,-1.9589087282169));
#7647=CARTESIAN_POINT('Ctrl Pts',(-0.0852553897503347,6.62356674643624,
-2.33034688916694));
#7648=CARTESIAN_POINT('Ctrl Pts',(-0.0430989621501437,7.39513483291858,
-2.12388655333521));
#7649=CARTESIAN_POINT('Ctrl Pts',(0.0412138930502383,8.70411999768534,-0.888377480332016));
#7650=CARTESIAN_POINT('Ctrl Pts',(0.167683175850812,8.2197990496567,1.7858097976561));
#7651=CARTESIAN_POINT('Ctrl Pts',(0.294152458651384,5.71600779530122,2.83214145593622));
#7652=CARTESIAN_POINT('Ctrl Pts',(0.420621741451958,3.47195465591787,1.30958567498853));
#7653=CARTESIAN_POINT('Ctrl Pts',(0.547091024252531,3.52272309657751,-1.40380861193092));
#7654=CARTESIAN_POINT('Ctrl Pts',(0.673560307053103,5.823661410867,-2.84155194939997));
#7655=CARTESIAN_POINT('Ctrl Pts',(0.800029589853677,8.28447684817651,-1.69924495783807));
#7656=CARTESIAN_POINT('Ctrl Pts',(0.926498872654249,8.67084224693258,0.986409006944131));
#7657=CARTESIAN_POINT('Ctrl Pts',(1.05296815545482,6.6316835898229,2.77616550532978));
#7658=CARTESIAN_POINT('Ctrl Pts',(1.1794374382554,4.01891562422582,2.04488343285502));
#7659=CARTESIAN_POINT('Ctrl Pts',(1.30590672105597,3.20519647830103,-0.543436073671827));
#7660=CARTESIAN_POINT('Ctrl Pts',(1.43237600385654,4.92951264141021,-2.63823216492743));
#7661=CARTESIAN_POINT('Ctrl Pts',(1.55884528665712,7.62595765439769,-2.33719779446077));
#7662=CARTESIAN_POINT('Ctrl Pts',(1.68531456945769,8.84583597533803,0.0863040582086905));
#7663=CARTESIAN_POINT('Ctrl Pts',(1.81178385225826,7.4813439140143,2.43142884274551));
#7664=CARTESIAN_POINT('Ctrl Pts',(1.93825313505883,4.77161021040782,2.56851855015692));
#7665=CARTESIAN_POINT('Ctrl Pts',(2.06472241785941,3.17740506463998,0.37307698504849));
#7666=CARTESIAN_POINT('Ctrl Pts',(2.19119170065998,4.14646334402713,-2.16116401154155));
#7667=CARTESIAN_POINT('Ctrl Pts',(2.31766098346055,6.79876067926811,-2.73280256214906));
#7668=CARTESIAN_POINT('Ctrl Pts',(2.44413026626113,8.72568517166943,-0.822720314907301));
#7669=CARTESIAN_POINT('Ctrl Pts',(2.5705995490617,8.17735239481401,1.83449307783794));
#7670=CARTESIAN_POINT('Ctrl Pts',(2.69706883186227,5.65171596835802,2.82576124286347));
#7671=CARTESIAN_POINT('Ctrl Pts',(2.82353811466284,3.44236425375709,1.25089077844456));
#7672=CARTESIAN_POINT('Ctrl Pts',(2.95000739746342,3.55566024451705,-1.45994229429062));
#7673=CARTESIAN_POINT('Ctrl Pts',(3.07647668026399,5.88871724572051,-2.84496827760426));
#7674=CARTESIAN_POINT('Ctrl Pts',(3.20294596306456,8.32283267039175,-1.64641329383313));
#7675=CARTESIAN_POINT('Ctrl Pts',(3.32941524586514,8.6475304535636,1.04728737487113));
#7676=CARTESIAN_POINT('Ctrl Pts',(3.45588452866571,6.56794508967739,2.7899223509744));
#7677=CARTESIAN_POINT('Ctrl Pts',(3.58235381146628,3.97259575928665,1.99896483049539));
#7678=CARTESIAN_POINT('Ctrl Pts',(3.70882309426686,3.21837873485823,-0.607298514815273));
#7679=CARTESIAN_POINT('Ctrl Pts',(3.83529237706743,4.99021580020368,-2.66206014560021));
#7680=CARTESIAN_POINT('Ctrl Pts',(3.96176165986801,7.67906106496106,-2.29934388228426));
#7681=CARTESIAN_POINT('Ctrl Pts',(4.08823094266857,8.84311245379272,0.151459314531306));
#7682=CARTESIAN_POINT('Ctrl Pts',(4.21470022546915,7.42526819360171,2.46471883288909));
#7683=CARTESIAN_POINT('Ctrl Pts',(4.34116950826972,4.71310518676386,2.53971063086796));
#7684=CARTESIAN_POINT('Ctrl Pts',(4.4676387910703,3.16960088515058,0.308332936189166));
#7685=CARTESIAN_POINT('Ctrl Pts',(4.59410807387087,4.19644695778789,-2.2030489719499));
#7686=CARTESIAN_POINT('Ctrl Pts',(4.72057735667144,6.86114092710966,-2.71379156394459));
#7687=CARTESIAN_POINT('Ctrl Pts',(4.84704663947202,8.74381306330275,-0.760077774000557));
#7688=CARTESIAN_POINT('Ctrl Pts',(4.97351592227259,8.13476560520423,1.88388008103432));
#7689=CARTESIAN_POINT('Ctrl Pts',(5.09998520507317,5.58708852293413,2.81704321248145));
#7690=CARTESIAN_POINT('Ctrl Pts',(5.22645448787373,3.41438582644622,1.19198477104298));
#7691=CARTESIAN_POINT('Ctrl Pts',(5.35292377067431,3.58973868290013,-1.51554238877461));
#7692=CARTESIAN_POINT('Ctrl Pts',(5.47939305347488,5.95390514021654,-2.8467707341446));
#7693=CARTESIAN_POINT('Ctrl Pts',(5.60586233627546,8.35993139726009,-1.59278126216586));
#7694=CARTESIAN_POINT('Ctrl Pts',(5.73233161907603,8.62284980837074,1.10764941728427));
#7695=CARTESIAN_POINT('Ctrl Pts',(5.8588009018766,6.50389813226231,2.80219824801587));
#7696=CARTESIAN_POINT('Ctrl Pts',(5.98527018467718,3.92734500127429,1.95200655868209));
#7697=CARTESIAN_POINT('Ctrl Pts',(6.11173946747773,3.23301742770633,-0.670847071622082));
#7698=CARTESIAN_POINT('Ctrl Pts',(6.23820875027833,5.05145021112467,-2.68448908489215));
#7699=CARTESIAN_POINT('Ctrl Pts',(6.36467803307889,7.73128282046858,-2.26028496973954));
#7700=CARTESIAN_POINT('Ctrl Pts',(6.49114731587947,8.83889777959534,0.216535784319152));
#7701=CARTESIAN_POINT('Ctrl Pts',(6.61761659868004,7.36844453202843,2.49671542464112));
#7702=CARTESIAN_POINT('Ctrl Pts',(6.74408588148061,4.6552754086039,2.50957050551929));
#7703=CARTESIAN_POINT('Ctrl Pts',(6.87055516428119,3.16328153873884,0.243427033073461));
#7704=CARTESIAN_POINT('Ctrl Pts',(6.99702444708175,4.24737678659332,-2.24377811307125));
#7705=CARTESIAN_POINT('Ctrl Pts',(7.12349372988233,6.92306938509461,-2.6933568755676));
#7706=CARTESIAN_POINT('Ctrl Pts',(7.2499630126829,8.76050149696535,-0.697036465476021));
#7707=CARTESIAN_POINT('Ctrl Pts',(7.37643229548347,8.09105886500692,1.93227875107649));
#7708=CARTESIAN_POINT('Ctrl Pts',(7.50290157828406,5.52267770250222,2.80684730135633));
#7709=CARTESIAN_POINT('Ctrl Pts',(7.62937086108461,3.38776386943321,1.13245341957922));
#7710=CARTESIAN_POINT('Ctrl Pts',(7.75584014388521,3.62508159957098,-1.57034739450059));
#7711=CARTESIAN_POINT('Ctrl Pts',(7.88230942668576,6.01911721647024,-2.84707971099935));
#7712=CARTESIAN_POINT('Ctrl Pts',(8.00877870948634,8.39579205162815,-1.53831362125216));
#7713=CARTESIAN_POINT('Ctrl Pts',(8.13524799228692,8.5967931556797,1.16743036173818));
#7714=CARTESIAN_POINT('Ctrl Pts',(8.26171727508749,6.43958682082974,2.81300404852356));
#7715=CARTESIAN_POINT('Ctrl Pts',(8.38818655788806,3.88318160049148,1.90402422039959));
#7716=CARTESIAN_POINT('Ctrl Pts',(8.51465584068864,3.24910775042176,-0.734043687424681));
#7717=CARTESIAN_POINT('Ctrl Pts',(8.64112512348919,5.11318223672586,-2.70550967959111));
#7718=CARTESIAN_POINT('Ctrl Pts',(8.7675944062898,7.78259633645583,-2.22004026262758));
#7719=CARTESIAN_POINT('Ctrl Pts',(8.89406368909034,8.83319369708346,0.281498658298747));
#7720=CARTESIAN_POINT('Ctrl Pts',(9.02053297189094,7.31090306545242,2.52740217592696));
#7721=CARTESIAN_POINT('Ctrl Pts',(9.14700225469149,4.59815088911334,2.47811381659131));
#7722=CARTESIAN_POINT('Ctrl Pts',(9.27347153749208,3.15845080896311,0.178393396289211));
#7723=CARTESIAN_POINT('Ctrl Pts',(9.39994082029265,4.29922529601587,-2.28333006709043));
#7724=CARTESIAN_POINT('Ctrl Pts',(9.52641010309322,6.98451508303819,-2.67150928794886));
#7725=CARTESIAN_POINT('Ctrl Pts',(9.6528793858938,8.77573883183555,-0.633629290988387));
#7726=CARTESIAN_POINT('Ctrl Pts',(9.77934866869436,8.04626061668093,1.97966335008995));
#7727=CARTESIAN_POINT('Ctrl Pts',(9.90581795149495,5.45850675035994,2.79517953242645));
#7728=CARTESIAN_POINT('Ctrl Pts',(10.0322872342955,3.36253253962162,1.07232666015524));
#7729=CARTESIAN_POINT('Ctrl Pts',(10.1587565170961,3.66163180123505,-1.62432607686547));
#7730=CARTESIAN_POINT('Ctrl Pts',(10.2852257998967,6.08439325825112,-2.84589980051202));
#7731=CARTESIAN_POINT('Ctrl Pts',(10.4116950826972,8.43025415685968,-1.48302984198647));
#7732=CARTESIAN_POINT('Ctrl Pts',(10.5381643654978,8.56964540984608,1.22658140488878));
#7733=CARTESIAN_POINT('Ctrl Pts',(10.6646336482984,6.37452525664845,2.82236757599056));
#7734=CARTESIAN_POINT('Ctrl Pts',(10.791102931099,3.84112676894634,1.85497794353522));
#7735=CARTESIAN_POINT('Ctrl Pts',(10.9175722138995,3.26470148965294,-0.79672235663028));
#7736=CARTESIAN_POINT('Ctrl Pts',(11.0440414967001,5.17935418061835,-2.72543940467849));
#7737=CARTESIAN_POINT('Ctrl Pts',(11.1283543519005,6.94187158889785,-2.36012143829251));
#7738=CARTESIAN_POINT('Ctrl Pts',(11.1705107795007,7.55304610346956,-1.84591438360752));
#7739=CARTESIAN_POINT('Ctrl Pts',(-0.170510779500669,6.58539622430396,-2.18769887591546));
#7740=CARTESIAN_POINT('Ctrl Pts',(-0.128354351900478,7.30973415156126,-1.9938766399557));
#7741=CARTESIAN_POINT('Ctrl Pts',(-0.0440414967000963,8.53859213268954,
-0.833997043163702));
#7742=CARTESIAN_POINT('Ctrl Pts',(0.0824277861004767,8.08391802450845,1.67649464768213));
#7743=CARTESIAN_POINT('Ctrl Pts',(0.20889706890105,5.73339186973559,2.65877698654563));
#7744=CARTESIAN_POINT('Ctrl Pts',(0.335366351701623,3.62670442618572,1.2294217321918));
#7745=CARTESIAN_POINT('Ctrl Pts',(0.461835634502196,3.67436516763127,-1.31787698071835));
#7746=CARTESIAN_POINT('Ctrl Pts',(0.588304917302769,5.83445566193595,-2.66761143349777));
#7747=CARTESIAN_POINT('Ctrl Pts',(0.714774200103342,8.14463668737201,-1.59522871957328));
#7748=CARTESIAN_POINT('Ctrl Pts',(0.841243482903916,8.50735141987839,0.926027745361123));
#7749=CARTESIAN_POINT('Ctrl Pts',(0.967712765704488,6.59301620965272,2.60622750355264));
#7750=CARTESIAN_POINT('Ctrl Pts',(1.09418204850506,4.14018415793702,1.91970955407172));
#7751=CARTESIAN_POINT('Ctrl Pts',(1.22065133130563,3.37627537288617,-0.5101706072304));
#7752=CARTESIAN_POINT('Ctrl Pts',(1.34712061410621,4.99504060878001,-2.47673750566767));
#7753=CARTESIAN_POINT('Ctrl Pts',(1.47358989690678,7.52642756722094,-2.19413041530558));
#7754=CARTESIAN_POINT('Ctrl Pts',(1.60005917970735,8.6716332204569,0.0810211097788901));
#7755=CARTESIAN_POINT('Ctrl Pts',(1.72652846250793,7.39066609808113,2.28259327865317));
#7756=CARTESIAN_POINT('Ctrl Pts',(1.8529977453085,4.84680389242928,2.41129128503055));
#7757=CARTESIAN_POINT('Ctrl Pts',(1.97946702810908,3.3501851608628,0.350239745256248));
#7758=CARTESIAN_POINT('Ctrl Pts',(2.10593631090965,4.25992427239468,-2.02887222528856));
#7759=CARTESIAN_POINT('Ctrl Pts',(2.23240559371022,6.74986597415332,-2.56551894531445));
#7760=CARTESIAN_POINT('Ctrl Pts',(2.35887487651079,8.55883723315213,-0.772358963587151));
#7761=CARTESIAN_POINT('Ctrl Pts',(2.48534415931136,8.04406966565793,1.72219786801588));
#7762=CARTESIAN_POINT('Ctrl Pts',(2.61181344211194,5.6730355518895,2.65278732679486));
#7763=CARTESIAN_POINT('Ctrl Pts',(2.73828272491251,3.59892534752324,1.17431973866966));
#7764=CARTESIAN_POINT('Ctrl Pts',(2.86475200771308,3.7052861270207,-1.37057454019767));
#7765=CARTESIAN_POINT('Ctrl Pts',(2.99122129051366,5.89552922031577,-2.67081863728663));
#7766=CARTESIAN_POINT('Ctrl Pts',(3.11769057331423,8.18064462659133,-1.54563105130611));
#7767=CARTESIAN_POINT('Ctrl Pts',(3.24415985611481,8.48546661620991,0.983179552974222));
#7768=CARTESIAN_POINT('Ctrl Pts',(3.37062913891538,6.53317934769492,2.61914224851735));
#7769=CARTESIAN_POINT('Ctrl Pts',(3.49709842171595,4.09669968061262,1.87660177675634));
#7770=CARTESIAN_POINT('Ctrl Pts',(3.62356770451652,3.38865070120585,-0.570123823359812));
#7771=CARTESIAN_POINT('Ctrl Pts',(3.7500369873171,5.05202793237307,-2.49910689915819));
#7772=CARTESIAN_POINT('Ctrl Pts',(3.87650627011767,7.57628034756741,-2.15859366260042));
#7773=CARTESIAN_POINT('Ctrl Pts',(4.00297555291824,8.6690764144076,0.14218800372056));
#7774=CARTESIAN_POINT('Ctrl Pts',(4.12944483571882,7.33802295251209,2.31384548164274));
#7775=CARTESIAN_POINT('Ctrl Pts',(4.25591411851938,4.79188014907748,2.38424679095162));
#7776=CARTESIAN_POINT('Ctrl Pts',(4.38238340131997,3.34285870025051,0.289458887449109));
#7777=CARTESIAN_POINT('Ctrl Pts',(4.50885268412053,4.30684822871507,-2.06819327282405));
#7778=CARTESIAN_POINT('Ctrl Pts',(4.63532196692111,6.80842772679051,-2.54767167133336));
#7779=CARTESIAN_POINT('Ctrl Pts',(4.76179124972169,8.57585545835,-0.7135509736852));
#7780=CARTESIAN_POINT('Ctrl Pts',(4.88826053252225,8.00408975013921,1.76856173421959));
#7781=CARTESIAN_POINT('Ctrl Pts',(5.01472981532284,5.61236415984724,2.64460295503647));
#7782=CARTESIAN_POINT('Ctrl Pts',(5.1411990981234,3.57265956955584,1.11901955706315));
#7783=CARTESIAN_POINT('Ctrl Pts',(5.26766838092398,3.7372785148022,-1.4227711744279));
#7784=CARTESIAN_POINT('Ctrl Pts',(5.39413766372454,5.95672675454348,-2.67251075967644));
#7785=CARTESIAN_POINT('Ctrl Pts',(5.52060694652512,8.2154724213051,-1.49528200845031));
#7786=CARTESIAN_POINT('Ctrl Pts',(5.64707622932569,8.46229675253154,1.03984664101552));
#7787=CARTESIAN_POINT('Ctrl Pts',(5.77354551212627,6.47305291012714,2.63066669849658));
#7788=CARTESIAN_POINT('Ctrl Pts',(5.90001479492684,4.05421886674831,1.8325179714918));
#7789=CARTESIAN_POINT('Ctrl Pts',(6.02648407772741,3.40239331267608,-0.629782369020372));
#7790=CARTESIAN_POINT('Ctrl Pts',(6.15295336052798,5.10951398844563,-2.52016289108156));
#7791=CARTESIAN_POINT('Ctrl Pts',(6.27942264332856,7.62530544179405,-2.12192567146752));
#7792=CARTESIAN_POINT('Ctrl Pts',(6.40589192612913,8.66511973394649,0.203280933904147));
#7793=CARTESIAN_POINT('Ctrl Pts',(6.53236120892971,7.28467764966163,2.34388345930797));
#7794=CARTESIAN_POINT('Ctrl Pts',(6.65883049173027,4.73759031726612,2.35595163942215));
#7795=CARTESIAN_POINT('Ctrl Pts',(6.78529977453086,3.33692618131707,0.228526083004159));
#7796=CARTESIAN_POINT('Ctrl Pts',(6.91176905733142,4.35466047921999,-2.10642925248115));
#7797=CARTESIAN_POINT('Ctrl Pts',(7.038238340132,6.86656534507845,-2.52848785582511));
#7798=CARTESIAN_POINT('Ctrl Pts',(7.16470762293257,8.59152233942002,-0.654368626011341));
#7799=CARTESIAN_POINT('Ctrl Pts',(7.29117690573314,7.96305843980337,1.8139977663139));
#7800=CARTESIAN_POINT('Ctrl Pts',(7.41764618853372,5.55189613248584,2.63503116835912));
#7801=CARTESIAN_POINT('Ctrl Pts',(7.54411547133428,3.54766722798525,1.06313231071179));
#7802=CARTESIAN_POINT('Ctrl Pts',(7.67058475413487,3.77045797809661,-1.47422138983515));
#7803=CARTESIAN_POINT('Ctrl Pts',(7.79705403693543,6.01794699028587,-2.67280082306613));
#7804=CARTESIAN_POINT('Ctrl Pts',(7.92352331973602,8.24913792991041,-1.44414850667227));
#7805=CARTESIAN_POINT('Ctrl Pts',(8.04999260253657,8.4378351111908,1.09596820196894));
#7806=CARTESIAN_POINT('Ctrl Pts',(8.17646188533716,6.41267830049983,2.64081104126973));
#7807=CARTESIAN_POINT('Ctrl Pts',(8.30293116813773,4.01275884948723,1.78747278615377));
#7808=CARTESIAN_POINT('Ctrl Pts',(8.4294004509383,3.41749869508988,-0.689110517115282));
#7809=CARTESIAN_POINT('Ctrl Pts',(8.55586973373887,5.16746719860653,-2.53989674770512));
#7810=CARTESIAN_POINT('Ctrl Pts',(8.68233901653946,7.6734778927568,-2.08414447205911));
#7811=CARTESIAN_POINT('Ctrl Pts',(8.80880829934001,8.65976481663465,0.264267221843539));
#7812=CARTESIAN_POINT('Ctrl Pts',(8.93527758214061,7.23065848095672,2.3726917760464));
#7813=CARTESIAN_POINT('Ctrl Pts',(9.06174686494115,4.6839625729772,2.32642051539608));
#7814=CARTESIAN_POINT('Ctrl Pts',(9.18821614774176,3.33239115601705,0.167473363878527));
#7815=CARTESIAN_POINT('Ctrl Pts',(9.31468543054229,4.40333517495259,-2.14356010443725));
#7816=CARTESIAN_POINT('Ctrl Pts',(9.4411547133429,6.92424975461675,-2.50797762917294));
#7817=CARTESIAN_POINT('Ctrl Pts',(9.56762399614345,8.60582694811258,-0.594842808204379));
#7818=CARTESIAN_POINT('Ctrl Pts',(9.69409327894404,7.92100243605504,1.85848180192222));
#7819=CARTESIAN_POINT('Ctrl Pts',(9.8205625617446,5.49165329030611,2.62407762101773));
#7820=CARTESIAN_POINT('Ctrl Pts',(9.94703184454518,3.52398038886132,1.00668610323265));
#7821=CARTESIAN_POINT('Ctrl Pts',(10.0735011273458,3.80477082459457,-1.52489586378665));
#7822=CARTESIAN_POINT('Ctrl Pts',(10.1999704101463,6.0792272760202,-2.67169313868712));
#7823=CARTESIAN_POINT('Ctrl Pts',(10.3264396929469,8.28149049906102,-1.39224882499048));
#7824=CARTESIAN_POINT('Ctrl Pts',(10.4529089757474,8.41234916602104,1.15149841989973));
#7825=CARTESIAN_POINT('Ctrl Pts',(10.5793782585481,6.35159936350278,2.64960139716456));
#7826=CARTESIAN_POINT('Ctrl Pts',(10.7058475413486,3.9732783291725,1.74142878932959));
#7827=CARTESIAN_POINT('Ctrl Pts',(10.8323168241492,3.43213789148847,-0.747952423786943));
#7828=CARTESIAN_POINT('Ctrl Pts',(10.9587861069498,5.22958854540846,-2.55860651034762));
#7829=CARTESIAN_POINT('Ctrl Pts',(11.0430989621501,6.88421660563383,-2.21565082931592));
#7830=CARTESIAN_POINT('Ctrl Pts',(11.0852553897503,7.45797916636344,-1.73292003899813));
#7831=CARTESIAN_POINT('Ctrl Pts',(-0.255766169251004,6.54722570217169,-2.04505086266398));
#7832=CARTESIAN_POINT('Ctrl Pts',(-0.213609741650813,7.22433347020394,-1.8638667265762));
#7833=CARTESIAN_POINT('Ctrl Pts',(-0.129296886450431,8.37306426769373,-0.779616605995389));
#7834=CARTESIAN_POINT('Ctrl Pts',(-0.00282760364985813,7.94803699936021,
1.56717949770815));
#7835=CARTESIAN_POINT('Ctrl Pts',(0.123641679150715,5.75077594416995,2.48541251715503));
#7836=CARTESIAN_POINT('Ctrl Pts',(0.250110961951289,3.78145419645358,1.14925778939507));
#7837=CARTESIAN_POINT('Ctrl Pts',(0.376580244751861,3.82600723868504,-1.23194534950577));
#7838=CARTESIAN_POINT('Ctrl Pts',(0.503049527552435,5.84524991300489,-2.49367091759558));
#7839=CARTESIAN_POINT('Ctrl Pts',(0.629518810353007,8.00479652656751,-1.49121248130849));
#7840=CARTESIAN_POINT('Ctrl Pts',(0.755988093153581,8.3438605928242,0.86564648377811));
#7841=CARTESIAN_POINT('Ctrl Pts',(0.882457375954154,6.55434882948256,2.43628950177551));
#7842=CARTESIAN_POINT('Ctrl Pts',(1.00892665875473,4.26145269164822,1.79453567528841));
#7843=CARTESIAN_POINT('Ctrl Pts',(1.1353959415553,3.54735426747131,-0.476905140788969));
#7844=CARTESIAN_POINT('Ctrl Pts',(1.26186522435587,5.06056857614981,-2.31524284640792));
#7845=CARTESIAN_POINT('Ctrl Pts',(1.38833450715645,7.42689748004418,-2.05106303615039));
#7846=CARTESIAN_POINT('Ctrl Pts',(1.51480378995702,8.49743046557577,0.0757381613490904));
#7847=CARTESIAN_POINT('Ctrl Pts',(1.64127307275759,7.29998828214797,2.13375771456083));
#7848=CARTESIAN_POINT('Ctrl Pts',(1.76774235555816,4.92199757445075,2.25406401990418));
#7849=CARTESIAN_POINT('Ctrl Pts',(1.89421163835874,3.52296525708561,0.327402505464004));
#7850=CARTESIAN_POINT('Ctrl Pts',(2.02068092115931,4.37338520076223,-1.89658043903557));
#7851=CARTESIAN_POINT('Ctrl Pts',(2.14715020395988,6.70097126903852,-2.39823532847985));
#7852=CARTESIAN_POINT('Ctrl Pts',(2.27361948676046,8.39198929463486,-0.721997612266999));
#7853=CARTESIAN_POINT('Ctrl Pts',(2.40008876956103,7.91078693650184,1.60990265819383));
#7854=CARTESIAN_POINT('Ctrl Pts',(2.52655805236161,5.69435513542099,2.47981341072626));
#7855=CARTESIAN_POINT('Ctrl Pts',(2.65302733516217,3.75548644128939,1.09774869889476));
#7856=CARTESIAN_POINT('Ctrl Pts',(2.77949661796276,3.85491200952435,-1.28120678610471));
#7857=CARTESIAN_POINT('Ctrl Pts',(2.90596590076332,5.90234119491101,-2.496668996969));
#7858=CARTESIAN_POINT('Ctrl Pts',(3.0324351835639,8.03845658279093,-1.44484880877908));
#7859=CARTESIAN_POINT('Ctrl Pts',(3.15890446636447,8.32340277885622,0.919071731077316));
#7860=CARTESIAN_POINT('Ctrl Pts',(3.28537374916504,6.49841360571246,2.44836214606031));
#7861=CARTESIAN_POINT('Ctrl Pts',(3.41184303196562,4.22080360193859,1.7542387230173));
#7862=CARTESIAN_POINT('Ctrl Pts',(3.53831231476619,3.55892266755349,-0.532949131904351));
#7863=CARTESIAN_POINT('Ctrl Pts',(3.66478159756676,5.11384006454244,-2.33615365271617));
#7864=CARTESIAN_POINT('Ctrl Pts',(3.79125088036733,7.47349963017379,-2.01784344291659));
#7865=CARTESIAN_POINT('Ctrl Pts',(3.91772016316791,8.49504037502246,0.132916692909814));
#7866=CARTESIAN_POINT('Ctrl Pts',(4.04418944596848,7.25077771142249,2.16297213039638));
#7867=CARTESIAN_POINT('Ctrl Pts',(4.17065872876906,4.87065511139108,2.22878295103529));
#7868=CARTESIAN_POINT('Ctrl Pts',(4.29712801156962,3.51611651535046,0.27058483870905));
#7869=CARTESIAN_POINT('Ctrl Pts',(4.42359729437021,4.41724949964224,-1.93333757369819));
#7870=CARTESIAN_POINT('Ctrl Pts',(4.55006657717077,6.75571452647139,-2.38155177872214));
#7871=CARTESIAN_POINT('Ctrl Pts',(4.67653585997135,8.40789785339724,-0.667024173369842));
#7872=CARTESIAN_POINT('Ctrl Pts',(4.80300514277192,7.8734138950742,1.65324338740486));
#7873=CARTESIAN_POINT('Ctrl Pts',(4.92947442557249,5.63763979676036,2.4721626975915));
#7874=CARTESIAN_POINT('Ctrl Pts',(5.05594370837307,3.73093331266546,1.04605434308332));
#7875=CARTESIAN_POINT('Ctrl Pts',(5.18241299117363,3.88481834670426,-1.32999996008119));
#7876=CARTESIAN_POINT('Ctrl Pts',(5.30888227397422,5.95954836887043,-2.49825078520828));
#7877=CARTESIAN_POINT('Ctrl Pts',(5.43535155677478,8.07101344535011,-1.39778275473475));
#7878=CARTESIAN_POINT('Ctrl Pts',(5.56182083957536,8.30174369669236,0.972043864746774));
#7879=CARTESIAN_POINT('Ctrl Pts',(5.68829012237593,6.44220768799198,2.45913514897731));
#7880=CARTESIAN_POINT('Ctrl Pts',(5.8147594051765,4.18109273222233,1.7130293843015));
#7881=CARTESIAN_POINT('Ctrl Pts',(5.94122868797708,3.57176919764584,-0.588717666418658));
#7882=CARTESIAN_POINT('Ctrl Pts',(6.06769797077765,5.16757776576658,-2.35583669727097));
#7883=CARTESIAN_POINT('Ctrl Pts',(6.19416725357822,7.51932806311952,-1.9835663731955));
#7884=CARTESIAN_POINT('Ctrl Pts',(6.32063653637881,8.49134168829764,0.190026083489143));
#7885=CARTESIAN_POINT('Ctrl Pts',(6.44710581917936,7.20091076729482,2.19105149397482));
#7886=CARTESIAN_POINT('Ctrl Pts',(6.57357510197996,4.81990522592834,2.202332773325));
#7887=CARTESIAN_POINT('Ctrl Pts',(6.70004438478051,3.51057082389531,0.213625132934857));
#7888=CARTESIAN_POINT('Ctrl Pts',(6.82651366758109,4.46194417184665,-1.96908039189105));
#7889=CARTESIAN_POINT('Ctrl Pts',(6.95298295038166,6.81006130506229,-2.36361883608261));
#7890=CARTESIAN_POINT('Ctrl Pts',(7.07945223318223,8.42254318187467,-0.611700786546665));
#7891=CARTESIAN_POINT('Ctrl Pts',(7.20592151598281,7.83505801459984,1.69571678155131));
#7892=CARTESIAN_POINT('Ctrl Pts',(7.33239079878338,5.58111456246946,2.4632150353619));
#7893=CARTESIAN_POINT('Ctrl Pts',(7.45886008158396,3.70757058653729,0.993811201844362));
#7894=CARTESIAN_POINT('Ctrl Pts',(7.58532936438453,3.91583435662225,-1.37809538516971));
#7895=CARTESIAN_POINT('Ctrl Pts',(7.71179864718509,6.0167767641015,-2.49852193513291));
#7896=CARTESIAN_POINT('Ctrl Pts',(7.83826792998569,8.10248380819267,-1.34998339209237));
#7897=CARTESIAN_POINT('Ctrl Pts',(7.96473721278623,8.27887706670191,1.0245060421997));
#7898=CARTESIAN_POINT('Ctrl Pts',(8.09120649558683,6.38576978016992,2.46861803401591));
#7899=CARTESIAN_POINT('Ctrl Pts',(8.21767577838739,4.14233609848298,1.67092135190795));
#7900=CARTESIAN_POINT('Ctrl Pts',(8.34414506118797,3.58588963975799,-0.64417734680588));
#7901=CARTESIAN_POINT('Ctrl Pts',(8.47061434398853,5.22175216048721,-2.37428381581914));
#7902=CARTESIAN_POINT('Ctrl Pts',(8.59708362678913,7.56435944905776,-1.94824868149064));
#7903=CARTESIAN_POINT('Ctrl Pts',(8.72355290958967,8.48633593618585,0.247035785388331));
#7904=CARTESIAN_POINT('Ctrl Pts',(8.85002219239027,7.15041389646101,2.21798137616584));
#7905=CARTESIAN_POINT('Ctrl Pts',(8.97649147519083,4.76977425684107,2.17472721420083));
#7906=CARTESIAN_POINT('Ctrl Pts',(9.10296075799141,3.50633150307099,0.156553331467843));
#7907=CARTESIAN_POINT('Ctrl Pts',(9.22943004079197,4.5074450538893,-2.00379014178407));
#7908=CARTESIAN_POINT('Ctrl Pts',(9.35589932359255,6.86398442619531,-2.34444597039702));
#7909=CARTESIAN_POINT('Ctrl Pts',(9.48236860639313,8.43591506438961,-0.556056325420373));
#7910=CARTESIAN_POINT('Ctrl Pts',(9.60883788919369,7.79574425542913,1.7373002537545));
#7911=CARTESIAN_POINT('Ctrl Pts',(9.73530717199428,5.52479983025231,2.45297570960901));
#7912=CARTESIAN_POINT('Ctrl Pts',(9.86177645479484,3.68542823810099,0.941045546310063));
#7913=CARTESIAN_POINT('Ctrl Pts',(9.98824573759541,3.94790984795411,-1.42546565070784));
#7914=CARTESIAN_POINT('Ctrl Pts',(10.114715020396,6.07406129378925,-2.49748647686222));
#7915=CARTESIAN_POINT('Ctrl Pts',(10.2411843031966,8.13272684126239,-1.30146780799449));
#7916=CARTESIAN_POINT('Ctrl Pts',(10.3676535859971,8.25505292219599,1.07641543491069));
#7917=CARTESIAN_POINT('Ctrl Pts',(10.4941228687977,6.32867347035711,2.47683521833855));
#7918=CARTESIAN_POINT('Ctrl Pts',(10.6205921515983,4.10542988939866,1.62787963512397));
#7919=CARTESIAN_POINT('Ctrl Pts',(10.7470614343988,3.59957429332401,-0.69918249094361));
#7920=CARTESIAN_POINT('Ctrl Pts',(10.8735307171994,5.27982291019858,-2.39177361601674));
#7921=CARTESIAN_POINT('Ctrl Pts',(10.9578435723998,6.8265616223698,-2.07118022033933));
#7922=CARTESIAN_POINT('Ctrl Pts',(11.,7.36291222925732,-1.61992569438875));
#7923=CARTESIAN_POINT('Ctrl Pts',(0.710943720977492,8.11470858782477,0.00143578057856379));
#7924=CARTESIAN_POINT('Ctrl Pts',(0.725958511702855,8.11629544067967,0.251703656050626));
#7925=CARTESIAN_POINT('Ctrl Pts',(0.740973302428217,8.07519857973553,0.501468424247686));
#7926=CARTESIAN_POINT('Ctrl Pts',(0.75598809315358,7.98909795455781,0.734610492596574));
#7927=CARTESIAN_POINT('Ctrl Pts',(0.798144520753771,7.74735667171032,1.38919415644391));
#7928=CARTESIAN_POINT('Ctrl Pts',(0.840300948353963,7.15085275059643,1.91274182910972));
#7929=CARTESIAN_POINT('Ctrl Pts',(0.882457375954154,6.47045143373377,2.06755669436143));
#7930=CARTESIAN_POINT('Ctrl Pts',(0.924613803554345,5.7900501168711,2.22237155961314));
#7931=CARTESIAN_POINT('Ctrl Pts',(0.966770231154535,5.02575140425966,2.00845361745078));
#7932=CARTESIAN_POINT('Ctrl Pts',(1.00892665875473,4.52458564392446,1.52292117702337));
#7933=CARTESIAN_POINT('Ctrl Pts',(1.05108308635492,4.02341988358925,1.03738873659595));
#7934=CARTESIAN_POINT('Ctrl Pts',(1.09323951395511,3.78538707553028,0.28024179790349));
#7935=CARTESIAN_POINT('Ctrl Pts',(1.1353959415553,3.91857305628055,-0.4047212890459));
#7936=CARTESIAN_POINT('Ctrl Pts',(1.17755236915549,4.05175903703082,-1.08968437599529));
#7937=CARTESIAN_POINT('Ctrl Pts',(1.21970879675568,4.55616380659031,-1.7024636112016));
#7938=CARTESIAN_POINT('Ctrl Pts',(1.26186522435587,5.20275434201912,-1.96482326042851));
#7939=CARTESIAN_POINT('Ctrl Pts',(1.30402165195606,5.84934487744794,-2.22718290965541));
#7940=CARTESIAN_POINT('Ctrl Pts',(1.34617807955625,6.63812117874606,-2.1391229729029));
#7941=CARTESIAN_POINT('Ctrl Pts',(1.38833450715645,7.21093149365039,-1.74062613827673));
#7942=CARTESIAN_POINT('Ctrl Pts',(1.4292042450968,7.76625861201282,-1.35429214063134));
#7943=CARTESIAN_POINT('Ctrl Pts',(1.47007398303714,8.11860189172077,-0.676182228442241));
#7944=CARTESIAN_POINT('Ctrl Pts',(1.51094372097749,8.12031955932164,0.000387557394038608));
#7945=CARTESIAN_POINT('Ctrl Pts',(0.,6.66173726856851,-2.47299490241842));
#7946=CARTESIAN_POINT('Ctrl Pts',(-2.92724575880526E-17,6.74302007470053,
-2.4435642830524));
#7947=CARTESIAN_POINT('Ctrl Pts',(-8.31564143722506E-17,6.82243058251537,
-2.40977680229731));
#7948=CARTESIAN_POINT('Ctrl Pts',(-7.97972798949331E-17,6.89976867880956,
-2.37194498173918));
#7949=CARTESIAN_POINT('Ctrl Pts',(-7.62437812158347E-17,6.98158166512527,
-2.33192415932525));
#7950=CARTESIAN_POINT('Ctrl Pts',(1.83719249610399E-16,7.06107643989013,
-2.2873769918661));
#7951=CARTESIAN_POINT('Ctrl Pts',(2.32452945780892E-16,7.13798362917082,
-2.23862239524585));
#7952=CARTESIAN_POINT('Ctrl Pts',(2.75094929930074E-16,7.20527741979142,
-2.19596212320313));
#7953=CARTESIAN_POINT('Ctrl Pts',(-3.13354561198216E-16,7.27058988911543,
-2.15007935982338));
#7954=CARTESIAN_POINT('Ctrl Pts',(-3.40005801291454E-16,7.33371319645899,
-2.10116340617892));
#7955=CARTESIAN_POINT('Ctrl Pts',(-3.52840359175394E-16,7.36411177225105,
-2.07760672978032));
#7956=CARTESIAN_POINT('Ctrl Pts',(1.0360295682957E-16,7.39400223353409,
-2.05334632697955));
#7957=CARTESIAN_POINT('Ctrl Pts',(1.31838984174237E-16,7.42335885067487,
-2.02840199034912));
#7958=CARTESIAN_POINT('Ctrl Pts',(1.49593456598285E-16,7.44181793640698,
-2.01271729322671));
#7959=CARTESIAN_POINT('Ctrl Pts',(-5.01310080724556E-17,7.46006591992173,
-1.99676217065983));
#7960=CARTESIAN_POINT('Ctrl Pts',(-5.55111512312578E-17,7.47809603849993,
-1.98054141094945));
#7961=CARTESIAN_POINT('Ctrl Pts',(-5.89928980535388E-17,7.48976418676514,
-1.97004418496315));
#7962=CARTESIAN_POINT('Ctrl Pts',(-3.27549090266268E-17,7.50134210697178,
-1.9594346195351));
#7963=CARTESIAN_POINT('Ctrl Pts',(-4.16333634234434E-17,7.51281285098918,
-1.94872845073444));
#7964=CARTESIAN_POINT('Ctrl Pts',(-9.07143297655421E-17,7.57622424849985,
-1.88954369998029));
#7965=CARTESIAN_POINT('Ctrl Pts',(-1.47034643718728E-16,7.63647286263829,
-1.82731287118978));
#7966=CARTESIAN_POINT('Ctrl Pts',(-1.2490009027033E-16,7.69332727300807,
-1.76231279717448));
#7967=CARTESIAN_POINT('Ctrl Pts',(-1.02897662229704E-16,7.74984230846473,
-1.69770072110568));
#7968=CARTESIAN_POINT('Ctrl Pts',(-4.18758661845513E-16,7.80300405366629,
-1.63035153777999));
#7969=CARTESIAN_POINT('Ctrl Pts',(-4.85722573273506E-16,7.85254163516931,
-1.56051042864998));
#7970=CARTESIAN_POINT('Ctrl Pts',(-5.45725005239589E-16,7.89692935536835,
-1.49792990864085));
#7971=CARTESIAN_POINT('Ctrl Pts',(1.03285777158662E-17,7.93840696580168,
-1.43334792061814));
#7972=CARTESIAN_POINT('Ctrl Pts',(-6.93889390390723E-17,7.97674451927385,
-1.3669303939457));
#7973=CARTESIAN_POINT('Ctrl Pts',(-1.05037396214999E-16,7.99388848823845,
-1.33722948940558));
#7974=CARTESIAN_POINT('Ctrl Pts',(1.79461103361955E-17,8.01040405398028,
-1.30716143593201));
#7975=CARTESIAN_POINT('Ctrl Pts',(5.55111512312578E-17,8.02626824247406,
-1.27674080217197));
#7976=CARTESIAN_POINT('Ctrl Pts',(7.37723601010594E-17,8.03398018029529,
-1.26195264984184));
#7977=CARTESIAN_POINT('Ctrl Pts',(-5.37222981174814E-16,8.04153816448487,
-1.24708117637209));
#7978=CARTESIAN_POINT('Ctrl Pts',(-5.55111512312578E-16,8.04893941986435,
-1.23212805327155));
#7979=CARTESIAN_POINT('Ctrl Pts',(-5.69642358968991E-16,8.05495145663562,
-1.21998163738446));
#7980=CARTESIAN_POINT('Ctrl Pts',(2.79116992920913E-16,8.06086026851682,
-1.20778075528828));
#7981=CARTESIAN_POINT('Ctrl Pts',(2.63677968348475E-16,8.06665780144445,
-1.19554063643636));
#7982=CARTESIAN_POINT('Ctrl Pts',(1.6930174401095E-16,8.10209716910752,
-1.12071879796678));
#7983=CARTESIAN_POINT('Ctrl Pts',(-3.46947901332591E-16,8.13344607811337,
-1.04430567332096));
#7984=CARTESIAN_POINT('Ctrl Pts',(-3.05311331771918E-16,8.16046085298837,
-0.96652813442685));
#7985=CARTESIAN_POINT('Ctrl Pts',(-2.63674762211246E-16,8.18747562786337,
-0.888750595532739));
#7986=CARTESIAN_POINT('Ctrl Pts',(-8.32710016965256E-17,8.21015673786416,
-0.809607920476006));
#7987=CARTESIAN_POINT('Ctrl Pts',(-2.77555756156289E-17,8.22820692560612,
-0.729317175418125));
#7988=CARTESIAN_POINT('Ctrl Pts',(2.8467517448409E-17,8.2464872029431,-0.648002947099096));
#7989=CARTESIAN_POINT('Ctrl Pts',(-1.24010162979355E-16,8.26001706827931,
-0.565509980237511));
#7990=CARTESIAN_POINT('Ctrl Pts',(-1.94289029309402E-16,8.26887071011419,
-0.48222934860738));
#7991=CARTESIAN_POINT('Ctrl Pts',(-2.1762897265876E-16,8.27181104637248,
-0.454571457610426));
#7992=CARTESIAN_POINT('Ctrl Pts',(-3.6803890847137E-16,8.27423521289526,
-0.426826800529392));
#7993=CARTESIAN_POINT('Ctrl Pts',(-3.88578058618805E-16,8.27614473190817,
-0.399010127625446));
#7994=CARTESIAN_POINT('Ctrl Pts',(-3.9982746972E-16,8.27719058649453,-0.383774775299874));
#7995=CARTESIAN_POINT('Ctrl Pts',(-7.62784563143259E-17,8.27808204622248,
-0.368517824314681));
#7996=CARTESIAN_POINT('Ctrl Pts',(-8.32667268468867E-17,8.27881928950886,
-0.353241737063793));
#7997=CARTESIAN_POINT('Ctrl Pts',(-8.92262223760452E-17,8.27944799986697,
-0.340214511908367));
#7998=CARTESIAN_POINT('Ctrl Pts',(1.13306245230702E-17,8.27996424640881,
-0.327178880475876));
#7999=CARTESIAN_POINT('Ctrl Pts',(2.77555756156289E-17,8.28036828922386,
-0.314144138808217));
#8000=CARTESIAN_POINT('Ctrl Pts',(1.30673503817005E-16,8.28290000144603,
-0.232469094571197));
#8001=CARTESIAN_POINT('Ctrl Pts',(8.32667268468867E-17,8.28103543097395,
-0.150734510285442));
#8002=CARTESIAN_POINT('Ctrl Pts',(8.32667268468867E-17,8.27490228926521,
-0.0693021198429901));
#8003=CARTESIAN_POINT('Ctrl Pts',(8.32667268468867E-17,8.26876142391814,
0.0122328207055393));
#8004=CARTESIAN_POINT('Ctrl Pts',(1.8500451461589E-16,8.25834084135165,
0.0934658284870283));
#8005=CARTESIAN_POINT('Ctrl Pts',(5.55111512312578E-17,8.24371805826975,
0.17402142364346));
#8006=CARTESIAN_POINT('Ctrl Pts',(-7.19074938173633E-17,8.22932955867074,
0.253286372190899));
#8007=CARTESIAN_POINT('Ctrl Pts',(6.41784410555287E-17,8.21087195899808,
0.331896311753077));
#8008=CARTESIAN_POINT('Ctrl Pts',(1.94289029309402E-16,8.18837667526648,
0.409467604336036));
#8009=CARTESIAN_POINT('Ctrl Pts',(2.4652271985269E-16,8.17934580618128,
0.440609073652239));
#8010=CARTESIAN_POINT('Ctrl Pts',(1.7445856536241E-16,8.16966375078697,
0.471582780693396));
#8011=CARTESIAN_POINT('Ctrl Pts',(1.66533453693773E-16,8.15933082804816,
0.502362225180225));
#8012=CARTESIAN_POINT('Ctrl Pts',(1.62901681143594E-16,8.15459564869234,
0.516467255654357));
#8013=CARTESIAN_POINT('Ctrl Pts',(6.62171881083989E-16,8.14972350969714,
0.530531944514346));
#8014=CARTESIAN_POINT('Ctrl Pts',(6.66133814775094E-16,8.14471983929536,
0.544539167387205));
#8015=CARTESIAN_POINT('Ctrl Pts',(6.87161873422234E-16,8.11816273792442,
0.618882840708986));
#8016=CARTESIAN_POINT('Ctrl Pts',(-1.24134177748354E-16,8.08787072716445,
0.691710604375033));
#8017=CARTESIAN_POINT('Ctrl Pts',(-2.77555756156289E-17,8.05389882723943,
0.762666289558938));
#8018=CARTESIAN_POINT('Ctrl Pts',(4.37166554604183E-17,8.02870602066407,
0.815285449988755));
#8019=CARTESIAN_POINT('Ctrl Pts',(5.91214766369708E-16,8.00148860185591,
0.866874658240732));
#8020=CARTESIAN_POINT('Ctrl Pts',(4.9960036108132E-16,7.97225570207189,
0.917275970722266));
#8021=CARTESIAN_POINT('Ctrl Pts',(4.67062548093405E-16,7.96187333236407,
0.935176523312302));
#8022=CARTESIAN_POINT('Ctrl Pts',(5.93084551578718E-16,7.95123663480896,
0.952927120175963));
#8023=CARTESIAN_POINT('Ctrl Pts',(6.10622663543836E-16,7.9403457074372,
0.970520278191213));
#8024=CARTESIAN_POINT('Ctrl Pts',(6.2283322446657E-16,7.93276311630981,
0.982769163829288));
#8025=CARTESIAN_POINT('Ctrl Pts',(5.89454364215472E-16,7.92505825553759,
0.994940049303588));
#8026=CARTESIAN_POINT('Ctrl Pts',(5.82867087928207E-16,7.91723622740492,
1.00702299437693));
#8027=CARTESIAN_POINT('Ctrl Pts',(5.48320440966256E-16,7.87621398503319,
1.07039140637391));
#8028=CARTESIAN_POINT('Ctrl Pts',(6.74760874961288E-16,7.83193489245364,
1.13140409419983));
#8029=CARTESIAN_POINT('Ctrl Pts',(5.55111512312578E-16,7.78442983090767,
1.18972080081364));
#8030=CARTESIAN_POINT('Ctrl Pts',(4.53551463141926E-16,7.74410687155662,
1.23922083541523));
#8031=CARTESIAN_POINT('Ctrl Pts',(2.26389524579989E-16,7.70145896228683,
1.28677814743062));
#8032=CARTESIAN_POINT('Ctrl Pts',(4.9960036108132E-16,7.65648804272845,
1.3321604106817));
#8033=CARTESIAN_POINT('Ctrl Pts',(5.66398646151588E-16,7.64543507438408,
1.34331447922279));
#8034=CARTESIAN_POINT('Ctrl Pts',(7.18591525774023E-17,7.63424170833627,
1.35433703657155));
#8035=CARTESIAN_POINT('Ctrl Pts',(5.55111512312578E-17,7.62291087731919,
1.3652268607858));
#8036=CARTESIAN_POINT('Origin',(6.,6.,0.));
#8037=CARTESIAN_POINT('Origin',(11.,-6.,0.));
#8038=CARTESIAN_POINT('Ctrl Pts',(11.,-4.63708777074269,-1.61992569438875));
#8039=CARTESIAN_POINT('Ctrl Pts',(11.,-4.68916071039273,-1.67389115040286));
#8040=CARTESIAN_POINT('Ctrl Pts',(11.,-4.74418227950824,-1.7247197028367));
#8041=CARTESIAN_POINT('Ctrl Pts',(11.,-4.80179350695765,-1.77240163479619));
#8042=CARTESIAN_POINT('Ctrl Pts',(11.,-4.86093069393025,-1.8213465271434));
#8043=CARTESIAN_POINT('Ctrl Pts',(11.,-4.92279707407985,-1.86697639170717));
#8044=CARTESIAN_POINT('Ctrl Pts',(11.,-4.98704961307706,-1.9092500417527));
#8045=CARTESIAN_POINT('Ctrl Pts',(11.,-5.0009412869431,-1.91838978578032));
#8046=CARTESIAN_POINT('Ctrl Pts',(11.,-5.01494649271969,-1.92737366922165));
#8047=CARTESIAN_POINT('Ctrl Pts',(11.,-5.02905605736331,-1.93619735983612));
#8048=CARTESIAN_POINT('Ctrl Pts',(11.,-5.095826994682,-1.97795386386861));
#8049=CARTESIAN_POINT('Ctrl Pts',(11.,-5.16480894835441,-2.01605026992946));
#8050=CARTESIAN_POINT('Ctrl Pts',(11.,-5.23562552815997,-2.05045819483435));
#8051=CARTESIAN_POINT('Ctrl Pts',(11.,-5.29121456335243,-2.07746745387636));
#8052=CARTESIAN_POINT('Ctrl Pts',(11.,-5.34793515199878,-2.10220338751318));
#8053=CARTESIAN_POINT('Ctrl Pts',(11.,-5.40562122838672,-2.12463650733759));
#8054=CARTESIAN_POINT('Ctrl Pts',(11.,-5.42503819593862,-2.13218743100917));
#8055=CARTESIAN_POINT('Ctrl Pts',(11.,-5.44456464967012,-2.13947732652672));
#8056=CARTESIAN_POINT('Ctrl Pts',(11.,-5.46419453130331,-2.14650467737314));
#8057=CARTESIAN_POINT('Ctrl Pts',(11.,-5.48077911786492,-2.15244183535448));
#8058=CARTESIAN_POINT('Ctrl Pts',(11.,-5.49743964788631,-2.15819215670317));
#8059=CARTESIAN_POINT('Ctrl Pts',(11.,-5.5141504139477,-2.16374765702697));
#8060=CARTESIAN_POINT('Ctrl Pts',(11.,-5.59091180623393,-2.18926701012754));
#8061=CARTESIAN_POINT('Ctrl Pts',(11.,-5.66882884756264,-2.21071518477414));
#8062=CARTESIAN_POINT('Ctrl Pts',(11.,-5.74752223865727,-2.22806242052001));
#8063=CARTESIAN_POINT('Ctrl Pts',(11.,-5.82735436949371,-2.24566068098954));
#8064=CARTESIAN_POINT('Ctrl Pts',(11.,-5.90798634098841,-2.25903895400364));
#8065=CARTESIAN_POINT('Ctrl Pts',(11.,-5.98905364152142,-2.26812340437189));
#8066=CARTESIAN_POINT('Ctrl Pts',(11.,-6.06934098436991,-2.27712045221375));
#8067=CARTESIAN_POINT('Ctrl Pts',(11.,-6.15005628953376,-2.28190623150704));
#8068=CARTESIAN_POINT('Ctrl Pts',(11.,-6.2308622507703,-2.28236146501133));
#8069=CARTESIAN_POINT('Ctrl Pts',(11.,-6.26376631466807,-2.28254683539842));
#8070=CARTESIAN_POINT('Ctrl Pts',(11.,-6.29668552386031,-2.28201357588125));
#8071=CARTESIAN_POINT('Ctrl Pts',(11.,-6.32959734487964,-2.28075114470524));
#8072=CARTESIAN_POINT('Ctrl Pts',(11.,-6.34313630322685,-2.28023181752799));
#8073=CARTESIAN_POINT('Ctrl Pts',(11.,-6.3566759153337,-2.27958889854899));
#8074=CARTESIAN_POINT('Ctrl Pts',(11.,-6.37019720730564,-2.27882277952366));
#8075=CARTESIAN_POINT('Ctrl Pts',(11.,-6.45384130154684,-2.27408348892273));
#8076=CARTESIAN_POINT('Ctrl Pts',(11.,-6.53692139016417,-2.2646296568094));
#8077=CARTESIAN_POINT('Ctrl Pts',(11.,-6.61905941956099,-2.25039732976414));
#8078=CARTESIAN_POINT('Ctrl Pts',(11.,-6.63843261915327,-2.24704047162504));
#8079=CARTESIAN_POINT('Ctrl Pts',(11.,-6.65775349179807,-2.24341756918389));
#8080=CARTESIAN_POINT('Ctrl Pts',(11.,-6.67701720133506,-2.2395273783889));
#8081=CARTESIAN_POINT('Ctrl Pts',(11.,-6.75568871853955,-2.22364013655372));
#8082=CARTESIAN_POINT('Ctrl Pts',(11.,-6.83340685342578,-2.20329917928858));
#8083=CARTESIAN_POINT('Ctrl Pts',(11.,-6.90995038418047,-2.17879339655753));
#8084=CARTESIAN_POINT('Ctrl Pts',(11.,-6.98825812324156,-2.15372279397793));
#8085=CARTESIAN_POINT('Ctrl Pts',(11.,-7.06533723375411,-2.12429291956538));
#8086=CARTESIAN_POINT('Ctrl Pts',(11.,-7.14094474113465,-2.09075923730983));
#8087=CARTESIAN_POINT('Ctrl Pts',(11.,-7.15790725065089,-2.0832359711147));
#8088=CARTESIAN_POINT('Ctrl Pts',(11.,-7.17479564031027,-2.07550594796968));
#8089=CARTESIAN_POINT('Ctrl Pts',(11.,-7.19160706411186,-2.06757171297803));
#8090=CARTESIAN_POINT('Ctrl Pts',(11.,-7.20870424201776,-2.05950261491706));
#8091=CARTESIAN_POINT('Ctrl Pts',(11.,-7.2257270756284,-2.05121953031441));
#8092=CARTESIAN_POINT('Ctrl Pts',(11.,-7.24264281162302,-2.04274031453622));
#8093=CARTESIAN_POINT('Ctrl Pts',(11.,-7.31794347071332,-2.00499495501592));
#8094=CARTESIAN_POINT('Ctrl Pts',(11.,-7.39121475588854,-1.96332675494362));
#8095=CARTESIAN_POINT('Ctrl Pts',(11.,-7.46222053368768,-1.91806519793764));
#8096=CARTESIAN_POINT('Ctrl Pts',(11.,-7.53467721725653,-1.8718787830364));
#8097=CARTESIAN_POINT('Ctrl Pts',(11.,-7.60477566895564,-1.82195030921268));
#8098=CARTESIAN_POINT('Ctrl Pts',(11.,-7.67225632822043,-1.76857519958011));
#8099=CARTESIAN_POINT('Ctrl Pts',(11.,-7.7402204116953,-1.71481771638312));
#8100=CARTESIAN_POINT('Ctrl Pts',(11.,-7.80552992851377,-1.65756352815942));
#8101=CARTESIAN_POINT('Ctrl Pts',(11.,-7.86789832115903,-1.597066268732));
#8102=CARTESIAN_POINT('Ctrl Pts',(11.,-7.88758899419526,-1.57796634159826));
#8103=CARTESIAN_POINT('Ctrl Pts',(11.,-7.90698629455484,-1.55854283015653));
#8104=CARTESIAN_POINT('Ctrl Pts',(11.,-7.92608054802242,-1.53880285675951));
#8105=CARTESIAN_POINT('Ctrl Pts',(11.,-7.93886127755718,-1.52558991489516));
#8106=CARTESIAN_POINT('Ctrl Pts',(11.,-7.95150622626967,-1.51223518086157));
#8107=CARTESIAN_POINT('Ctrl Pts',(11.,-7.96401239792668,-1.49874069798903));
#8108=CARTESIAN_POINT('Ctrl Pts',(11.,-7.97296243208598,-1.48908337950791));
#8109=CARTESIAN_POINT('Ctrl Pts',(11.,-7.98184040084489,-1.47935546066086));
#8110=CARTESIAN_POINT('Ctrl Pts',(11.,-7.99063713711847,-1.46956699588278));
#8111=CARTESIAN_POINT('Ctrl Pts',(11.,-8.05020603751975,-1.40328240290278));
#8112=CARTESIAN_POINT('Ctrl Pts',(11.,-8.10615530524682,-1.33411428433584));
#8113=CARTESIAN_POINT('Ctrl Pts',(11.,-8.15821728462088,-1.26237772980875));
#8114=CARTESIAN_POINT('Ctrl Pts',(11.,-8.21030973545835,-1.19059918844553));
#8115=CARTESIAN_POINT('Ctrl Pts',(11.,-8.25851120867521,-1.11624858408148));
#8116=CARTESIAN_POINT('Ctrl Pts',(11.,-8.30252641897689,-1.03959725091855));
#8117=CARTESIAN_POINT('Ctrl Pts',(11.,-8.34556791606098,-0.964641613760129));
#8118=CARTESIAN_POINT('Ctrl Pts',(11.,-8.38460699954129,-0.88748521250845));
#8119=CARTESIAN_POINT('Ctrl Pts',(11.,-8.41933041215152,-0.808349409023425));
#8120=CARTESIAN_POINT('Ctrl Pts',(11.,-8.43267483371714,-0.777937031804278));
#8121=CARTESIAN_POINT('Ctrl Pts',(11.,-8.4453814194259,-0.74723202383003));
#8122=CARTESIAN_POINT('Ctrl Pts',(11.,-8.45743055670488,-0.716245966456263));
#8123=CARTESIAN_POINT('Ctrl Pts',(11.,-8.46428526209977,-0.69861812392042));
#8124=CARTESIAN_POINT('Ctrl Pts',(11.,-8.47092716798352,-0.680899312562034));
#8125=CARTESIAN_POINT('Ctrl Pts',(11.,-8.47735703821271,-0.663092892961399));
#8126=CARTESIAN_POINT('Ctrl Pts',(11.,-8.47299490241841,0.661737268568549));
#8127=CARTESIAN_POINT('Ctrl Pts',(11.,-8.44299217193241,0.744600156882087));
#8128=CARTESIAN_POINT('Ctrl Pts',(11.,-8.40842658662345,0.825613049231886));
#8129=CARTESIAN_POINT('Ctrl Pts',(11.,-8.36960246891694,0.904544308645214));
#8130=CARTESIAN_POINT('Ctrl Pts',(11.,-8.32947621078867,0.986122880850064));
#8131=CARTESIAN_POINT('Ctrl Pts',(11.,-8.28480032785149,1.06547870562738));
#8132=CARTESIAN_POINT('Ctrl Pts',(11.,-8.23586758286413,1.14231964012019));
#8133=CARTESIAN_POINT('Ctrl Pts',(11.,-8.22619772360642,1.15750458472054));
#8134=CARTESIAN_POINT('Ctrl Pts',(11.,-8.21636151332297,1.17259118394073));
#8135=CARTESIAN_POINT('Ctrl Pts',(11.,-8.20636105572507,1.18757697609823));
#8136=CARTESIAN_POINT('Ctrl Pts',(11.,-8.19636269232515,1.20255963007776));
#8137=CARTESIAN_POINT('Ctrl Pts',(11.,-8.18620566899149,1.21743322439163));
#8138=CARTESIAN_POINT('Ctrl Pts',(11.,-8.17589375376841,1.23219396468862));
#8139=CARTESIAN_POINT('Ctrl Pts',(11.,-8.12540468254945,1.30446531797046));
#8140=CARTESIAN_POINT('Ctrl Pts',(11.,-8.07119588129312,1.37404838032795));
#8141=CARTESIAN_POINT('Ctrl Pts',(11.,-8.0135480096579,1.44068419309266));
#8142=CARTESIAN_POINT('Ctrl Pts',(11.,-7.97155389150282,1.48922565898246));
#8143=CARTESIAN_POINT('Ctrl Pts',(11.,-7.92773394870726,1.53620245880582));
#8144=CARTESIAN_POINT('Ctrl Pts',(11.,-7.88218714794513,1.58149989349267));
#8145=CARTESIAN_POINT('Ctrl Pts',(11.,-7.86583399269375,1.5977635161737));
#8146=CARTESIAN_POINT('Ctrl Pts',(11.,-7.84925816751652,1.61381052543022));
#8147=CARTESIAN_POINT('Ctrl Pts',(11.,-7.83246407288259,1.62963517198371));
#8148=CARTESIAN_POINT('Ctrl Pts',(11.,-7.82132717922489,1.64012918250814));
#8149=CARTESIAN_POINT('Ctrl Pts',(11.,-7.81010043989387,1.65051957759726));
#8150=CARTESIAN_POINT('Ctrl Pts',(11.,-7.79878879465207,1.66080200414467));
#8151=CARTESIAN_POINT('Ctrl Pts',(11.,-7.73504595251212,1.71874504233381));
#8152=CARTESIAN_POINT('Ctrl Pts',(11.,-7.66857522386929,1.77329518611919));
#8153=CARTESIAN_POINT('Ctrl Pts',(11.,-7.59964161110829,1.82421541577063));
#8154=CARTESIAN_POINT('Ctrl Pts',(11.,-7.53207142409031,1.87412850319976));
#8155=CARTESIAN_POINT('Ctrl Pts',(11.,-7.46213399626932,1.92055421440432));
#8156=CARTESIAN_POINT('Ctrl Pts',(11.,-7.39005745111888,1.96322512488115));
#8157=CARTESIAN_POINT('Ctrl Pts',(11.,-7.31945832744952,2.00502136913163));
#8158=CARTESIAN_POINT('Ctrl Pts',(11.,-7.2468061944969,2.04321546128308));
#8159=CARTESIAN_POINT('Ctrl Pts',(11.,-7.17230561691982,2.07750845132568));
#8160=CARTESIAN_POINT('Ctrl Pts',(11.,-7.15028246724394,2.08764581773415));
#8161=CARTESIAN_POINT('Ctrl Pts',(11.,-7.12809776072295,2.09744194614622));
#8162=CARTESIAN_POINT('Ctrl Pts',(11.,-7.10575674483513,2.10688823607142));
#8163=CARTESIAN_POINT('Ctrl Pts',(11.,-7.08863683070083,2.11412692536018));
#8164=CARTESIAN_POINT('Ctrl Pts',(11.,-7.0714251291155,2.12116017596557));
#8165=CARTESIAN_POINT('Ctrl Pts',(11.,-7.05412400850806,2.12798394870633));
#8166=CARTESIAN_POINT('Ctrl Pts',(11.,-7.0421560960086,2.1327042391968));
#8167=CARTESIAN_POINT('Ctrl Pts',(11.,-7.0301482296559,2.13732310976275));
#8168=CARTESIAN_POINT('Ctrl Pts',(11.,-7.01811087072427,2.14183590822721));
#8169=CARTESIAN_POINT('Ctrl Pts',(11.,-6.94192107660596,2.17039941521055));
#8170=CARTESIAN_POINT('Ctrl Pts',(11.,-6.86443967890492,2.19476166022804));
#8171=CARTESIAN_POINT('Ctrl Pts',(11.,-6.78588043231568,2.21467983405259));
#8172=CARTESIAN_POINT('Ctrl Pts',(11.,-6.76708719688578,2.2194447337464));
#8173=CARTESIAN_POINT('Ctrl Pts',(11.,-6.74823223066446,2.22395507969414));
#8174=CARTESIAN_POINT('Ctrl Pts',(11.,-6.72931838764412,2.22820710552603));
#8175=CARTESIAN_POINT('Ctrl Pts',(11.,-6.64883815143219,2.24629988777883));
#8176=CARTESIAN_POINT('Ctrl Pts',(11.,-6.56729156100039,2.25971968137586));
#8177=CARTESIAN_POINT('Ctrl Pts',(11.,-6.48505615285959,2.26856864579746));
#8178=CARTESIAN_POINT('Ctrl Pts',(11.,-6.40338815460454,2.27735655391734));
#8179=CARTESIAN_POINT('Ctrl Pts',(11.,-6.32103982649442,2.28163608098665));
#8180=CARTESIAN_POINT('Ctrl Pts',(11.,-6.23839365107816,2.28145912099538));
#8181=CARTESIAN_POINT('Ctrl Pts',(11.,-6.21813581056131,2.28141574539739));
#8182=CARTESIAN_POINT('Ctrl Pts',(11.,-6.19786017422479,2.28110440549847));
#8183=CARTESIAN_POINT('Ctrl Pts',(11.,-6.17757259598781,2.28052546242847));
#8184=CARTESIAN_POINT('Ctrl Pts',(11.,-6.16489228263999,2.28016360654541));
#8185=CARTESIAN_POINT('Ctrl Pts',(11.,-6.15220804476619,2.27969715540688));
#8186=CARTESIAN_POINT('Ctrl Pts',(11.,-6.13953434549051,2.27912700305166));
#8187=CARTESIAN_POINT('Ctrl Pts',(11.,-6.05806362624421,2.27546187565287));
#8188=CARTESIAN_POINT('Ctrl Pts',(11.,-5.976885766891,2.26751233932642));
#8189=CARTESIAN_POINT('Ctrl Pts',(11.,-5.89635941922123,2.25539762204348));
#8190=CARTESIAN_POINT('Ctrl Pts',(11.,-5.81599843329012,2.24330778246543));
#8191=CARTESIAN_POINT('Ctrl Pts',(11.,-5.73628529198131,2.22706943595767));
#8192=CARTESIAN_POINT('Ctrl Pts',(11.,-5.65759278366309,2.20675219816744));
#8193=CARTESIAN_POINT('Ctrl Pts',(11.,-5.58032860266213,2.18680373329304));
#8194=CARTESIAN_POINT('Ctrl Pts',(11.,-5.50404751923812,2.16292262378908));
#8195=CARTESIAN_POINT('Ctrl Pts',(11.,-5.42913146009419,2.13513438322616));
#8196=CARTESIAN_POINT('Ctrl Pts',(11.,-5.39726310244459,2.12331361210136));
#8197=CARTESIAN_POINT('Ctrl Pts',(11.,-5.36564218650334,2.11078536423984));
#8198=CARTESIAN_POINT('Ctrl Pts',(11.,-5.3343002956742,2.09754964276009));
#8199=CARTESIAN_POINT('Ctrl Pts',(11.,-5.32160465228749,2.09218825595708));
#8200=CARTESIAN_POINT('Ctrl Pts',(11.,-5.30895358614716,2.08671013786179));
#8201=CARTESIAN_POINT('Ctrl Pts',(11.,-5.2963657193717,2.08112281913911));
#8202=CARTESIAN_POINT('Ctrl Pts',(11.,-5.22470595288081,2.0493155270761));
#8203=CARTESIAN_POINT('Ctrl Pts',(11.,-5.1549687226797,2.0139219178475));
#8204=CARTESIAN_POINT('Ctrl Pts',(11.,-5.08749005705245,1.97501188775492));
#8205=CARTESIAN_POINT('Ctrl Pts',(11.,-5.02118530622618,1.93677876879874));
#8206=CARTESIAN_POINT('Ctrl Pts',(11.,-4.95706050256354,1.8951500455755));
#8207=CARTESIAN_POINT('Ctrl Pts',(11.,-4.89546768821356,1.85015506607012));
#8208=CARTESIAN_POINT('Ctrl Pts',(11.,-4.8358598511882,1.80661015854118));
#8209=CARTESIAN_POINT('Ctrl Pts',(11.,-4.77862296475962,1.75991201329989));
#8210=CARTESIAN_POINT('Ctrl Pts',(11.,-4.72411594487011,1.7100591248934));
#8211=CARTESIAN_POINT('Ctrl Pts',(11.,-4.70501584604852,1.6925899053867));
#8212=CARTESIAN_POINT('Ctrl Pts',(11.,-4.68625134890234,1.67473308433625));
#8213=CARTESIAN_POINT('Ctrl Pts',(11.,-4.66783926694922,1.65648789471542));
#8214=CARTESIAN_POINT('Ctrl Pts',(11.,-4.6566873428301,1.64543705479909));
#8215=CARTESIAN_POINT('Ctrl Pts',(11.,-4.64566472044625,1.63424373084128));
#8216=CARTESIAN_POINT('Ctrl Pts',(11.,-4.63477280471478,1.62291072646336));
#8217=CARTESIAN_POINT('Origin',(-1.7667098902285,-6.,0.));
#8218=CARTESIAN_POINT('Ctrl Pts',(0.233290109771496,-3.4375580541705,0.00169662369046201));
#8219=CARTESIAN_POINT('Ctrl Pts',(0.238897060498093,-3.43666696742173,0.114092740073729));
#8220=CARTESIAN_POINT('Ctrl Pts',(0.286660438824881,-3.49427689386692,1.07067089040277));
#8221=CARTESIAN_POINT('Ctrl Pts',(0.376580244751861,-4.69833585942183,2.72694181908363));
#8222=CARTESIAN_POINT('Ctrl Pts',(0.503049527552434,-7.57381067700105,2.57901747640416));
#8223=CARTESIAN_POINT('Ctrl Pts',(0.629518810353007,-9.02010634361806,0.0895593516203334));
#8224=CARTESIAN_POINT('Ctrl Pts',(0.755988093153582,-7.72375616695671,-2.48150715181869));
#8225=CARTESIAN_POINT('Ctrl Pts',(0.882457375954152,-4.86203286070258,-2.79891511344676));
#8226=CARTESIAN_POINT('Ctrl Pts',(0.97489138149346,-3.52575264953356,-1.17323436387186));
#8227=CARTESIAN_POINT('Ctrl Pts',(1.02516895943257,-3.43750802030871,-0.165257814947204));
#8228=CARTESIAN_POINT('Ctrl Pts',(1.0332901097715,-3.438979209753,-0.00218674096624601));
#8229=CARTESIAN_POINT('Ctrl Pts',(0.166709890228505,-3.44261795854501,-0.00304121041534603));
#8230=CARTESIAN_POINT('Ctrl Pts',(0.195452782019385,-3.44686084504951,0.576034429433346));
#8231=CARTESIAN_POINT('Ctrl Pts',(0.266352101410457,-3.92613180196041,2.01289446940098));
#8232=CARTESIAN_POINT('Ctrl Pts',(0.379407848401719,-6.30137623450992,3.00550525361278));
#8233=CARTESIAN_POINT('Ctrl Pts',(0.505877131202293,-8.68279501755112,1.3897499208415));
#8234=CARTESIAN_POINT('Ctrl Pts',(0.632346414002865,-8.62891891149828,-1.48974040295355));
#8235=CARTESIAN_POINT('Ctrl Pts',(0.758815696803439,-6.18713281460021,-3.01549224619728));
#8236=CARTESIAN_POINT('Ctrl Pts',(0.870270188878651,-3.8857217769571,-1.94718070444853));
#8237=CARTESIAN_POINT('Ctrl Pts',(0.939568253353674,-3.44623974036578,-0.545331334169339));
#8238=CARTESIAN_POINT('Ctrl Pts',(0.966709890228505,-3.4427709916825,0.00173622513077922));
#8239=CARTESIAN_POINT('Ctrl Pts',(-2.77555756156289E-16,-7.61992569438872,
1.36291222925734));
#8240=CARTESIAN_POINT('Ctrl Pts',(0.0421564276001907,-8.07118022033932,
0.826561622369841));
#8241=CARTESIAN_POINT('Ctrl Pts',(0.126469282800573,-8.39177520902806,-0.720175462073977));
#8242=CARTESIAN_POINT('Ctrl Pts',(0.252938565601146,-6.69918148311235,-2.40042657120791));
#8243=CARTESIAN_POINT('Ctrl Pts',(0.379407848401718,-4.37212097158592,-1.89456935454149));
#8244=CARTESIAN_POINT('Ctrl Pts',(0.505877131202293,-3.52316464584869,0.328673032761782));
#8245=CARTESIAN_POINT('Ctrl Pts',(0.632346414002864,-4.92358477124844,2.25505305898439));
#8246=CARTESIAN_POINT('Ctrl Pts',(0.758815696803439,-7.30146765750439,2.13272656154203));
#8247=CARTESIAN_POINT('Ctrl Pts',(0.88528497960401,-8.49748637868727,0.074061385695407));
#8248=CARTESIAN_POINT('Ctrl Pts',(1.01175426240459,-7.42546554900288,-2.05209009390631));
#8249=CARTESIAN_POINT('Ctrl Pts',(1.13822354520516,-5.05895451801068,-2.31457159967453));
#8250=CARTESIAN_POINT('Ctrl Pts',(1.26469282800573,-3.54702442124209,-0.475200162100537));
#8251=CARTESIAN_POINT('Ctrl Pts',(1.3911621108063,-4.26269984665637,1.79574416585738));
#8252=CARTESIAN_POINT('Ctrl Pts',(1.51763139360688,-6.55605629257995,2.43591492214283));
#8253=CARTESIAN_POINT('Ctrl Pts',(1.64410067640745,-8.34444584030976,0.863984381349539));
#8254=CARTESIAN_POINT('Ctrl Pts',(1.77056995920802,-8.00379002929963,-1.49255486462238));
#8255=CARTESIAN_POINT('Ctrl Pts',(1.8970392420086,-5.84344667754611,-2.49366835649056));
#8256=CARTESIAN_POINT('Ctrl Pts',(2.02350852480917,-3.82527290719829,-1.23022567500147));
#8257=CARTESIAN_POINT('Ctrl Pts',(2.14997780760974,-3.78201874786567,1.15041383249752));
#8258=CARTESIAN_POINT('Ctrl Pts',(2.27644709041031,-5.75296422837819,2.48633579704923));
#8259=CARTESIAN_POINT('Ctrl Pts',(2.40291637321089,-7.9482485726293,1.56435936173015));
#8260=CARTESIAN_POINT('Ctrl Pts',(2.52938565601146,-8.37428368311575,-0.778247796073561));
#8261=CARTESIAN_POINT('Ctrl Pts',(2.65585493881204,-6.6441773108105,-2.41411022529385));
#8262=CARTESIAN_POINT('Ctrl Pts',(2.78232422161261,-4.3290787414722,-1.85766379771369));
#8263=CARTESIAN_POINT('Ctrl Pts',(2.90879350441318,-3.53138210395009,0.38576975861922));
#8264=CARTESIAN_POINT('Ctrl Pts',(3.03526278721376,-4.97549401505624,2.27887693933677));
#8265=CARTESIAN_POINT('Ctrl Pts',(3.16173207001432,-7.3499833166459,2.10248369069325));
#8266=CARTESIAN_POINT('Ctrl Pts',(3.2882013528149,-8.49852179549707,0.0167767631624936));
#8267=CARTESIAN_POINT('Ctrl Pts',(3.41467063561548,-7.37809530815189,-2.08416552689859));
#8268=CARTESIAN_POINT('Ctrl Pts',(3.54113991841604,-5.00618885369701,-2.29242928534551));
#8269=CARTESIAN_POINT('Ctrl Pts',(3.66760920121662,-3.53678510230054,-0.418885414119979));
#8270=CARTESIAN_POINT('Ctrl Pts',(3.79407848401719,-4.30428331321763,1.83505791204326));
#8271=CARTESIAN_POINT('Ctrl Pts',(3.92054776681776,-6.61170075236032,2.4225430464854));
#8272=CARTESIAN_POINT('Ctrl Pts',(4.04701704961834,-8.36361870398636,0.810061259790201));
#8273=CARTESIAN_POINT('Ctrl Pts',(4.1734863324189,-7.96908028184454,-1.53805574219553));
#8274=CARTESIAN_POINT('Ctrl Pts',(4.29995561521949,-5.78637487900414,-2.48942903697728));
#8275=CARTESIAN_POINT('Ctrl Pts',(4.42642489802005,-3.7976673497574,-1.18009470811942));
#8276=CARTESIAN_POINT('Ctrl Pts',(4.55289418082064,-3.80894862847708,1.20091070017914));
#8277=CARTESIAN_POINT('Ctrl Pts',(4.6793634636212,-5.80997392713084,2.49134154906332));
#8278=CARTESIAN_POINT('Ctrl Pts',(4.80583274642178,-7.98356626233935,1.51932797820845));
#8279=CARTESIAN_POINT('Ctrl Pts',(4.93230202922234,-8.35583656560968,-0.832422187711553));
#8280=CARTESIAN_POINT('Ctrl Pts',(5.05877131202293,-6.58871763351688,-2.42823066664694));
#8281=CARTESIAN_POINT('Ctrl Pts',(5.18524059482349,-4.28697071143509,-1.81890716612392));
#8282=CARTESIAN_POINT('Ctrl Pts',(5.31170987762408,-3.54086498845706,0.442207663278129));
#8283=CARTESIAN_POINT('Ctrl Pts',(5.43817916042463,-5.02795618957805,2.30174356805414));
#8284=CARTESIAN_POINT('Ctrl Pts',(5.56464844322522,-7.39778267661641,2.07101332960685));
#8285=CARTESIAN_POINT('Ctrl Pts',(5.69111772602579,-8.49825064558784,-0.0404516288687811));
#8286=CARTESIAN_POINT('Ctrl Pts',(5.81758700882636,-7.32999988575116,-2.11518153508395));
#8287=CARTESIAN_POINT('Ctrl Pts',(5.94405629162693,-4.95394571537787,-2.2690665605226));
#8288=CARTESIAN_POINT('Ctrl Pts',(6.07052557442751,-3.52783744057095,-0.362360182988378));
#8289=CARTESIAN_POINT('Ctrl Pts',(6.19699485722807,-4.34675670499038,1.87341379037416));
#8290=CARTESIAN_POINT('Ctrl Pts',(6.32346414002865,-6.66702413609162,2.40789771882639));
#8291=CARTESIAN_POINT('Ctrl Pts',(6.44993342282923,-8.38155164562368,0.7557144842366));
#8292=CARTESIAN_POINT('Ctrl Pts',(6.57640270562979,-7.93333746564924,-1.58275041190211));
#8293=CARTESIAN_POINT('Ctrl Pts',(6.70287198843038,-5.72941517641325,-2.48388334583205));
#8294=CARTESIAN_POINT('Ctrl Pts',(6.82934127123094,-3.77121717352535,-1.12934482549294));
#8295=CARTESIAN_POINT('Ctrl Pts',(6.95581055403152,-3.83702799048622,1.25077764151987));
#8296=CARTESIAN_POINT('Ctrl Pts',(7.08227983683208,-5.86708331451848,2.49504023558143));
#8297=CARTESIAN_POINT('Ctrl Pts',(7.20874911963267,-8.01784333014474,1.47349954782397));
#8298=CARTESIAN_POINT('Ctrl Pts',(7.33521840243323,-8.33615352215498,-0.886159885932465));
#8299=CARTESIAN_POINT('Ctrl Pts',(7.46168768523382,-6.53294910211921,-2.44107719602128));
#8300=CARTESIAN_POINT('Ctrl Pts',(7.58815696803438,-4.24576137502258,-1.7791962986271));
#8301=CARTESIAN_POINT('Ctrl Pts',(7.71462625083496,-3.55163799077159,0.49841357785763));
#8302=CARTESIAN_POINT('Ctrl Pts',(7.84109553363553,-5.08092832028779,2.32340264900719));
#8303=CARTESIAN_POINT('Ctrl Pts',(7.9675648164361,-7.44484872802906,2.03845646886778));
#8304=CARTESIAN_POINT('Ctrl Pts',(8.09403409923668,-8.4966688574394,-0.0976587996322113));
#8305=CARTESIAN_POINT('Ctrl Pts',(8.22050338203724,-7.28120671449707,-2.14508787059042));
#8306=CARTESIAN_POINT('Ctrl Pts',(8.34697266483783,-4.90225136246375,-2.24451343327464));
#8307=CARTESIAN_POINT('Ctrl Pts',(8.47344194763839,-3.5201867278485,-0.305644847490535));
#8308=CARTESIAN_POINT('Ctrl Pts',(8.59991123043897,-4.39009743180727,1.91078682970075));
#8309=CARTESIAN_POINT('Ctrl Pts',(8.72638051323955,-6.72199757186506,2.39198916097544));
#8310=CARTESIAN_POINT('Ctrl Pts',(8.85284979604012,-8.39823519454311,0.700971229823036));
#8311=CARTESIAN_POINT('Ctrl Pts',(8.97931907884069,-7.89658033286896,-1.62661470825881));
#8312=CARTESIAN_POINT('Ctrl Pts',(9.10578836164127,-5.67259751314697,-2.47703460460759));
#8313=CARTESIAN_POINT('Ctrl Pts',(9.23225764444182,-3.74593610549994,-1.07800236507619));
#8314=CARTESIAN_POINT('Ctrl Pts',(9.35872692724242,-3.86624240572105,1.29998820909676));
#8315=CARTESIAN_POINT('Ctrl Pts',(9.48519621004297,-5.92426184101915,2.49743032669638));
#8316=CARTESIAN_POINT('Ctrl Pts',(9.61166549284356,-8.05106292487872,1.42689739909694));
#8317=CARTESIAN_POINT('Ctrl Pts',(9.73813477564412,-8.31524271099646,-0.939431369294025));
#8318=CARTESIAN_POINT('Ctrl Pts',(9.8646040584447,-6.47690512487916,-2.45264559891613));
#8319=CARTESIAN_POINT('Ctrl Pts',(9.99107334124527,-4.20546440592863,-1.73854720547185));
#8320=CARTESIAN_POINT('Ctrl Pts',(10.1175426240458,-3.56371066804312,0.554348789288414));
#8321=CARTESIAN_POINT('Ctrl Pts',(10.2440119068464,-5.1343535056252,2.34386047615449));
#8322=CARTESIAN_POINT('Ctrl Pts',(10.370481189647,-7.49121250041255,2.0047963934507));
#8323=CARTESIAN_POINT('Ctrl Pts',(10.4969504724476,-8.49367060210842,-0.154750050135963));
#8324=CARTESIAN_POINT('Ctrl Pts',(10.6234197552481,-7.23194557971607,-2.17399267067328));
#8325=CARTESIAN_POINT('Ctrl Pts',(10.7498890380487,-4.85074177411285,-2.21854566422902));
#8326=CARTESIAN_POINT('Ctrl Pts',(10.8763583208493,-3.51458845010521,-0.249223991557292));
#8327=CARTESIAN_POINT('Ctrl Pts',(11.0028276036499,-4.43281921636254,1.94803666841403));
#8328=CARTESIAN_POINT('Ctrl Pts',(11.1292968864504,-6.77961885270218,2.37306464117732));
#8329=CARTESIAN_POINT('Ctrl Pts',(11.2136097416508,-7.86386672657618,1.22433347020397));
#8330=CARTESIAN_POINT('Ctrl Pts',(11.255766169251,-8.04505086266397,0.547225702171725));
#8331=CARTESIAN_POINT('Ctrl Pts',(-0.085255389750335,-7.73292003899811,
1.45797916636347));
#8332=CARTESIAN_POINT('Ctrl Pts',(-0.043098962150144,-8.21565082931591,
0.884216605633869));
#8333=CARTESIAN_POINT('Ctrl Pts',(0.0412138930502382,-8.55860821447594,
-0.770409713325555));
#8334=CARTESIAN_POINT('Ctrl Pts',(0.167683175850811,-6.74795134565662,-2.56786303334696));
#8335=CARTESIAN_POINT('Ctrl Pts',(0.294152458651384,-4.25857185970001,-2.02672086203038));
#8336=CARTESIAN_POINT('Ctrl Pts',(0.420621741451957,-3.35039845754936,0.351598895383963));
#8337=CARTESIAN_POINT('Ctrl Pts',(0.547091024252531,-4.84850180063956,2.4123493123508));
#8338=CARTESIAN_POINT('Ctrl Pts',(0.673560307053103,-7.39224866400329,2.28149019982941));
#8339=CARTESIAN_POINT('Ctrl Pts',(0.800029589853677,-8.67169303366418,0.079227374337048));
#8340=CARTESIAN_POINT('Ctrl Pts',(0.926498872654249,-7.52489575498751,-2.19522911321044));
#8341=CARTESIAN_POINT('Ctrl Pts',(1.05296815545482,-4.99331396557464,-2.47601943759861));
#8342=CARTESIAN_POINT('Ctrl Pts',(1.1794374382554,-3.3759225189606,-0.508346701513314));
#8343=CARTESIAN_POINT('Ctrl Pts',(1.30590672105597,-4.14151830549257,1.92100234023541));
#8344=CARTESIAN_POINT('Ctrl Pts',(1.43237600385654,-6.59484277307325,2.60582679594369));
#8345=CARTESIAN_POINT('Ctrl Pts',(1.55884528665711,-8.50797749001172,0.924249706642856));
#8346=CARTESIAN_POINT('Ctrl Pts',(1.68531456945769,-8.14355998410671,-1.59666473787506));
#8347=CARTESIAN_POINT('Ctrl Pts',(1.81178385225826,-5.83252664576418,-2.66760869374852));
#8348=CARTESIAN_POINT('Ctrl Pts',(1.93825313505883,-3.67357961447098,-1.31603735411116));
#8349=CARTESIAN_POINT('Ctrl Pts',(2.06472241785941,-3.62730835663665,1.23065841253159));
#8350=CARTESIAN_POINT('Ctrl Pts',(2.19119170065998,-5.73573279288324,2.65976466779286));
#8351=CARTESIAN_POINT('Ctrl Pts',(2.31766098346055,-8.08414435560439,1.67347779933784));
#8352=CARTESIAN_POINT('Ctrl Pts',(2.44413026626113,-8.53989660574529,-0.832532754924229));
#8353=CARTESIAN_POINT('Ctrl Pts',(2.5705995490617,-6.68911047860912,-2.58250116054896));
#8354=CARTESIAN_POINT('Ctrl Pts',(2.69706883186227,-4.2125273137399,-1.98724103946888));
#8355=CARTESIAN_POINT('Ctrl Pts',(2.82353811466284,-3.35918910631978,0.412678277445913));
#8356=CARTESIAN_POINT('Ctrl Pts',(2.95000739746342,-4.90403185928076,2.43783497494159));
#8357=CARTESIAN_POINT('Ctrl Pts',(3.07647668026399,-7.44414842596318,2.24913780421508));
#8358=CARTESIAN_POINT('Ctrl Pts',(3.20294596306457,-8.6728006736903,0.0179469892813684));
#8359=CARTESIAN_POINT('Ctrl Pts',(3.32941524586514,-7.4742213074451,-2.22954189729948));
#8360=CARTESIAN_POINT('Ctrl Pts',(3.45588452866571,-4.93686774870375,-2.45233263496102));
#8361=CARTESIAN_POINT('Ctrl Pts',(3.58235381146628,-3.36496897890566,-0.448103842470657));
#8362=CARTESIAN_POINT('Ctrl Pts',(3.70882309426686,-4.18600233506543,1.9630583300932));
#8363=CARTESIAN_POINT('Ctrl Pts',(3.83529237706743,-6.65436858944041,2.59152219458696));
#8364=CARTESIAN_POINT('Ctrl Pts',(3.961761659868,-8.52848771451476,0.8665652966485));
#8365=CARTESIAN_POINT('Ctrl Pts',(4.08823094266857,-8.1064291347586,-1.64533942882639));
#8366=CARTESIAN_POINT('Ctrl Pts',(4.21470022546916,-5.7714739297676,-2.66307366985099));
#8367=CARTESIAN_POINT('Ctrl Pts',(4.34116950826972,-3.64404849224561,-1.26240961218128));
#8368=CARTESIAN_POINT('Ctrl Pts',(4.4676387910703,-3.65611667168528,1.28467757786444));
#8369=CARTESIAN_POINT('Ctrl Pts',(4.59410807387086,-5.79671907745662,2.66511958500019));
#8370=CARTESIAN_POINT('Ctrl Pts',(4.72057735667144,-8.12192555287883,1.6253053509602));
#8371=CARTESIAN_POINT('Ctrl Pts',(4.84704663947201,-8.52016275023653,-0.890485961787482));
#8372=CARTESIAN_POINT('Ctrl Pts',(4.97351592227259,-6.6297823338236,-2.59760654215074));
#8373=CARTESIAN_POINT('Ctrl Pts',(5.09998520507316,-4.16748213092269,-1.94578102450731));
#8374=CARTESIAN_POINT('Ctrl Pts',(5.22645448787373,-3.36933344852421,0.473052883689435));
#8375=CARTESIAN_POINT('Ctrl Pts',(5.35292377067431,-4.96015341709861,2.46229661492046));
#8376=CARTESIAN_POINT('Ctrl Pts',(5.47939305347488,-7.49528192488301,2.21547229748841));
#8377=CARTESIAN_POINT('Ctrl Pts',(5.60586233627545,-8.67251061031707,-0.043273243038023));
#8378=CARTESIAN_POINT('Ctrl Pts',(5.73233161907603,-7.42277109491315,-2.26272135874042));
#8379=CARTESIAN_POINT('Ctrl Pts',(5.8588009018766,-4.88098050547587,-2.42734029478673));
#8380=CARTESIAN_POINT('Ctrl Pts',(5.98527018467717,-3.3553971927632,-0.387635818488908));
#8381=CARTESIAN_POINT('Ctrl Pts',(6.11173946747774,-4.23143836462047,2.00408963813605));
#8382=CARTESIAN_POINT('Ctrl Pts',(6.23820875027832,-6.71355093380672,2.57585531439246));
#8383=CARTESIAN_POINT('Ctrl Pts',(6.36467803307889,-8.54767152895091,0.808427681609743));
#8384=CARTESIAN_POINT('Ctrl Pts',(6.49114731587946,-8.06819315723838,-1.69315167665925));
#8385=CARTESIAN_POINT('Ctrl Pts',(6.61761659868005,-5.71054112872801,-2.65714115124909));
#8386=CARTESIAN_POINT('Ctrl Pts',(6.74408588148061,-3.61575334229747,-1.20811978340404));
#8387=CARTESIAN_POINT('Ctrl Pts',(6.87055516428119,-3.68615464767176,1.33802287773358));
#8388=CARTESIAN_POINT('Ctrl Pts',(6.99702444708175,-5.85781200422589,2.66907626524016));
#8389=CARTESIAN_POINT('Ctrl Pts',(7.12349372988232,-8.15859354196241,1.57628025947347));
#8390=CARTESIAN_POINT('Ctrl Pts',(7.24996301268291,-8.49910675948999,-0.947972014647327));
#8391=CARTESIAN_POINT('Ctrl Pts',(7.37643229548347,-6.57012379149707,-2.61134915285286));
#8392=CARTESIAN_POINT('Ctrl Pts',(7.50290157828406,-4.12339832812209,-1.90330021301725));
#8393=CARTESIAN_POINT('Ctrl Pts',(7.62937086108461,-3.38085789785896,0.53317931789714));
#8394=CARTESIAN_POINT('Ctrl Pts',(7.7558401438852,-5.01682050197373,2.48546647730356));
#8395=CARTESIAN_POINT('Ctrl Pts',(7.88230942668576,-7.54563096492355,2.18064450472173));
#8396=CARTESIAN_POINT('Ctrl Pts',(8.00877870948635,-8.67081848802445,-0.104470773846832));
#8397=CARTESIAN_POINT('Ctrl Pts',(8.13524799228691,-7.3705744635952,-2.29471374473175));
#8398=CARTESIAN_POINT('Ctrl Pts',(8.26171727508749,-4.82568032696878,-2.40107451829127));
#8399=CARTESIAN_POINT('Ctrl Pts',(8.38818655788806,-3.34721282144588,-0.326964429830057));
#8400=CARTESIAN_POINT('Ctrl Pts',(8.51465584068863,-4.27780222826304,2.04406955140716));
#8401=CARTESIAN_POINT('Ctrl Pts',(8.64112512348922,-6.77235892036706,2.5588370901696));
#8402=CARTESIAN_POINT('Ctrl Pts',(8.76759440628977,-8.56551880203525,0.749865932202442));
#8403=CARTESIAN_POINT('Ctrl Pts',(8.89406368909036,-8.02887211171653,-1.74007563028033));
#8404=CARTESIAN_POINT('Ctrl Pts',(9.02053297189093,-5.64976027465288,-2.64981469118311));
#8405=CARTESIAN_POINT('Ctrl Pts',(9.1470022546915,-3.58870884912087,-1.15319604287949));
#8406=CARTESIAN_POINT('Ctrl Pts',(9.27347153749207,-3.71740685001871,1.3906660199344));
#8407=CARTESIAN_POINT('Ctrl Pts',(9.39994082029265,-5.91897889275454,2.67163307189029));
#8408=CARTESIAN_POINT('Ctrl Pts',(9.52641010309321,-8.19413029627241,1.52642748062739));
#8409=CARTESIAN_POINT('Ctrl Pts',(9.6528793858938,-8.47673736081089,-1.00495933285839));
#8410=CARTESIAN_POINT('Ctrl Pts',(9.77934866869435,-6.51017059021083,-2.62372448418141));
#8411=CARTESIAN_POINT('Ctrl Pts',(9.90581795149495,-4.08029053281044,-1.85981573200689));
#8412=CARTESIAN_POINT('Ctrl Pts',(10.0322872342955,-3.39377267811131,0.593016166654935));
#8413=CARTESIAN_POINT('Ctrl Pts',(10.1587565170961,-5.07397224330304,2.50735129507063));
#8414=CARTESIAN_POINT('Ctrl Pts',(10.2852257998967,-7.59522874000989,2.14463654496994));
#8415=CARTESIAN_POINT('Ctrl Pts',(10.4116950826972,-8.6676110960045,-0.165544298633874));
#8416=CARTESIAN_POINT('Ctrl Pts',(10.5381643654978,-7.31787722698646,-2.32563473540455));
#8417=CARTESIAN_POINT('Ctrl Pts',(10.6646336482984,-4.77057780086958,-2.37329542477909));
#8418=CARTESIAN_POINT('Ctrl Pts',(10.791102931099,-3.34122404818372,-0.266608061508461));
#8419=CARTESIAN_POINT('Ctrl Pts',(10.9175722138995,-4.3235039766914,2.08391767047786));
#8420=CARTESIAN_POINT('Ctrl Pts',(11.0440414967001,-6.83399944658457,2.53859253222465));
#8421=CARTESIAN_POINT('Ctrl Pts',(11.1283543519005,-7.99387663995568,1.30973415156129));
#8422=CARTESIAN_POINT('Ctrl Pts',(11.1705107795007,-8.18769887591545,0.585396224303999));
#8423=CARTESIAN_POINT('Ctrl Pts',(-0.17051077950067,-7.84591438360749,1.55304610346959));
#8424=CARTESIAN_POINT('Ctrl Pts',(-0.128354351900479,-8.3601214382925,0.941871588897895));
#8425=CARTESIAN_POINT('Ctrl Pts',(-0.0440414967000962,-8.7254412199238,
-0.820643964577131));
#8426=CARTESIAN_POINT('Ctrl Pts',(0.0824277861004762,-6.79672120820092,
-2.73529949548601));
#8427=CARTESIAN_POINT('Ctrl Pts',(0.20889706890105,-4.14502274781409,-2.15887236951926));
#8428=CARTESIAN_POINT('Ctrl Pts',(0.335366351701622,-3.17763226925003,0.374524758006143));
#8429=CARTESIAN_POINT('Ctrl Pts',(0.461835634502197,-4.77341883003069,2.56964556571722));
#8430=CARTESIAN_POINT('Ctrl Pts',(0.588304917302768,-7.48302967050217,2.43025383811678));
#8431=CARTESIAN_POINT('Ctrl Pts',(0.714774200103343,-8.84589968864111,0.0843933629786898));
#8432=CARTESIAN_POINT('Ctrl Pts',(0.841243482903914,-7.62432596097212,-2.33836813251456));
#8433=CARTESIAN_POINT('Ctrl Pts',(0.967712765704489,-4.9276734131386,-2.63746727552268));
#8434=CARTESIAN_POINT('Ctrl Pts',(1.09418204850506,-3.20482061667911,-0.541493240926087));
#8435=CARTESIAN_POINT('Ctrl Pts',(1.22065133130563,-4.02033676432878,2.04626051461342));
#8436=CARTESIAN_POINT('Ctrl Pts',(1.34712061410621,-6.63362925356655,2.77573866974455));
#8437=CARTESIAN_POINT('Ctrl Pts',(1.47358989690678,-8.67150913971368,0.98451503193617));
#8438=CARTESIAN_POINT('Ctrl Pts',(1.60005917970735,-8.2833299389138,-1.70077461112773));
#8439=CARTESIAN_POINT('Ctrl Pts',(1.72652846250792,-5.82160661398222,-2.84154903100648));
#8440=CARTESIAN_POINT('Ctrl Pts',(1.8529977453085,-3.52188632174367,-1.40184903322085));
#8441=CARTESIAN_POINT('Ctrl Pts',(1.97946702810907,-3.47259796540763,1.31090299256566));
#8442=CARTESIAN_POINT('Ctrl Pts',(2.10593631090964,-5.71850135738828,2.8331935385365));
#8443=CARTESIAN_POINT('Ctrl Pts',(2.23240559371022,-8.22004013857948,1.78259623694553));
#8444=CARTESIAN_POINT('Ctrl Pts',(2.35887487651079,-8.70550952837483,-0.886817713774895));
#8445=CARTESIAN_POINT('Ctrl Pts',(2.48534415931136,-6.73404364640775,-2.75089209580407));
#8446=CARTESIAN_POINT('Ctrl Pts',(2.61181344211194,-4.0959758860076,-2.11681828122406));
#8447=CARTESIAN_POINT('Ctrl Pts',(2.73828272491251,-3.18699610868948,0.439586796272604));
#8448=CARTESIAN_POINT('Ctrl Pts',(2.86475200771309,-4.83256970350528,2.5967930105464));
#8449=CARTESIAN_POINT('Ctrl Pts',(2.99122129051365,-7.53831353528048,2.3957919177369));
#8450=CARTESIAN_POINT('Ctrl Pts',(3.11769057331423,-8.84707955188353,0.0191172154002425));
#8451=CARTESIAN_POINT('Ctrl Pts',(3.2441598561148,-7.57034730673834,-2.37491826770037));
#8452=CARTESIAN_POINT('Ctrl Pts',(3.37062913891538,-4.86754664371048,-2.61223598457652));
#8453=CARTESIAN_POINT('Ctrl Pts',(3.49709842171595,-3.19315285551078,-0.477322270821332));
#8454=CARTESIAN_POINT('Ctrl Pts',(3.62356770451652,-4.06772135691324,2.09105874814314));
#8455=CARTESIAN_POINT('Ctrl Pts',(3.7500369873171,-6.69703642652049,2.76050134268853));
#8456=CARTESIAN_POINT('Ctrl Pts',(3.87650627011767,-8.69335672504318,0.923069333506797));
#8457=CARTESIAN_POINT('Ctrl Pts',(4.00297555291824,-8.24377798767264,-1.75262311545725));
#8458=CARTESIAN_POINT('Ctrl Pts',(4.12944483571881,-5.75657298053108,-2.83671830272471));
#8459=CARTESIAN_POINT('Ctrl Pts',(4.25591411851939,-3.4904296347338,-1.34472451624315));
#8460=CARTESIAN_POINT('Ctrl Pts',(4.38238340131996,-3.50328471489348,1.36844445554975));
#8461=CARTESIAN_POINT('Ctrl Pts',(4.50885268412054,-5.78346422778239,2.83889762093706));
#8462=CARTESIAN_POINT('Ctrl Pts',(4.63532196692111,-8.26028484341833,1.73128272371194));
#8463=CARTESIAN_POINT('Ctrl Pts',(4.76179124972168,-8.68448893486336,-0.94854973586341));
#8464=CARTESIAN_POINT('Ctrl Pts',(4.88826053252225,-6.67084703413032,-2.76698241765453));
#8465=CARTESIAN_POINT('Ctrl Pts',(5.01472981532283,-4.04799355041029,-2.07265488289069));
#8466=CARTESIAN_POINT('Ctrl Pts',(5.1411990981234,-3.19780190859137,0.503898104100741));
#8467=CARTESIAN_POINT('Ctrl Pts',(5.26766838092397,-4.89235064461916,2.62284966178678));
#8468=CARTESIAN_POINT('Ctrl Pts',(5.39413766372455,-7.59278117314959,2.35993126536998));
#8469=CARTESIAN_POINT('Ctrl Pts',(5.52060694652512,-8.84677057504632,-0.0460948572072665));
#8470=CARTESIAN_POINT('Ctrl Pts',(5.64707622932569,-7.51554230407514,-2.41026118239688));
#8471=CARTESIAN_POINT('Ctrl Pts',(5.77354551212627,-4.80801529557386,-2.58561402905087));
#8472=CARTESIAN_POINT('Ctrl Pts',(5.90001479492683,-3.18295694495545,-0.412911453989435));
#8473=CARTESIAN_POINT('Ctrl Pts',(6.02648407772741,-4.11612002425056,2.13476548589794));
#8474=CARTESIAN_POINT('Ctrl Pts',(6.15295336052799,-6.76007773152183,2.74381290995853));
#8475=CARTESIAN_POINT('Ctrl Pts',(6.27942264332856,-8.71379141227815,0.861140878982882));
#8476=CARTESIAN_POINT('Ctrl Pts',(6.40589192612912,-8.20304884882752,-1.8035529414164));
#8477=CARTESIAN_POINT('Ctrl Pts',(6.53236120892971,-5.69166708104277,-2.83039895666613));
#8478=CARTESIAN_POINT('Ctrl Pts',(6.65883049173027,-3.46028951106959,-1.28689474131513));
#8479=CARTESIAN_POINT('Ctrl Pts',(6.78529977453086,-3.5352813048573,1.42526811394729));
#8480=CARTESIAN_POINT('Ctrl Pts',(6.91176905733142,-5.84854069393329,2.84311229489889));
#8481=CARTESIAN_POINT('Ctrl Pts',(7.03823834013199,-8.2993437537801,1.67906097112298));
#8482=CARTESIAN_POINT('Ctrl Pts',(7.16470762293257,-8.662059996825,-1.00978414336219));
#8483=CARTESIAN_POINT('Ctrl Pts',(7.29117690573314,-6.60729848087495,-2.78162110968445));
#8484=CARTESIAN_POINT('Ctrl Pts',(7.41764618853372,-4.00103528122159,-2.02740412740739));
#8485=CARTESIAN_POINT('Ctrl Pts',(7.54411547133428,-3.21007780494632,0.567945057936651));
#8486=CARTESIAN_POINT('Ctrl Pts',(7.67058475413486,-4.95271268365969,2.64753030559991));
#8487=CARTESIAN_POINT('Ctrl Pts',(7.79705403693543,-7.64641320181803,2.32283254057568));
#8488=CARTESIAN_POINT('Ctrl Pts',(7.92352331973601,-8.8449681186095,-0.111282748061457));
#8489=CARTESIAN_POINT('Ctrl Pts',(8.04999260253658,-7.45994221269332,-2.44433961887307));
#8490=CARTESIAN_POINT('Ctrl Pts',(8.17646188533714,-4.7491092914738,-2.55763560330791));
#8491=CARTESIAN_POINT('Ctrl Pts',(8.30293116813774,-3.17423891504325,-0.34828401216958));
#8492=CARTESIAN_POINT('Ctrl Pts',(8.42940045093828,-4.16550702471881,2.17735227311358));
#8493=CARTESIAN_POINT('Ctrl Pts',(8.55586973373889,-6.82272026886908,2.72568501936376));
#8494=CARTESIAN_POINT('Ctrl Pts',(8.68233901653944,-8.73280240952739,0.798760634581848));
#8495=CARTESIAN_POINT('Ctrl Pts',(8.80880829934001,-8.16116389056411,-1.85353655230184));
#8496=CARTESIAN_POINT('Ctrl Pts',(8.93527758214061,-5.62692303615881,-2.82259477775864));
#8497=CARTESIAN_POINT('Ctrl Pts',(9.06174686494115,-3.43148159274178,-1.22838972068279));
#8498=CARTESIAN_POINT('Ctrl Pts',(9.18821614774175,-3.56857129431638,1.48134383077204));
#8499=CARTESIAN_POINT('Ctrl Pts',(9.3146854305423,-5.91369594448993,2.84583581708419));
#8500=CARTESIAN_POINT('Ctrl Pts',(9.44115471334289,-8.33719766766608,1.62595756215785));
#8501=CARTESIAN_POINT('Ctrl Pts',(9.56762399614346,-8.63823201062531,-1.07048729642275));
#8502=CARTESIAN_POINT('Ctrl Pts',(9.69409327894403,-6.54343605554251,-2.7948033694467));
#8503=CARTESIAN_POINT('Ctrl Pts',(9.8205625617446,-3.95511665969225,-1.98108425854193));
#8504=CARTESIAN_POINT('Ctrl Pts',(9.94703184454517,-3.22383468817951,0.631683544021454));
#8505=CARTESIAN_POINT('Ctrl Pts',(10.0735011273458,-5.01359098098088,2.67084211398678));
#8506=CARTESIAN_POINT('Ctrl Pts',(10.1999704101463,-7.69924497960724,2.28447669648917));
#8507=CARTESIAN_POINT('Ctrl Pts',(10.3264396929469,-8.84155158990058,-0.176338547131783));
#8508=CARTESIAN_POINT('Ctrl Pts',(10.4529089757475,-7.40380887425685,-2.47727680013581));
#8509=CARTESIAN_POINT('Ctrl Pts',(10.579378258548,-4.69041382762631,-2.52804518532915));
#8510=CARTESIAN_POINT('Ctrl Pts',(10.7058475413486,-3.16785964626223,-0.283992131459634));
#8511=CARTESIAN_POINT('Ctrl Pts',(10.8323168241492,-4.21418873702027,2.2197986725417));
#8512=CARTESIAN_POINT('Ctrl Pts',(10.9587861069498,-6.88838004046696,2.70412042327197));
#8513=CARTESIAN_POINT('Ctrl Pts',(11.0430989621501,-8.12388655333519,1.39513483291862));
#8514=CARTESIAN_POINT('Ctrl Pts',(11.0852553897503,-8.33034688916693,0.623566746436274));
#8515=CARTESIAN_POINT('Ctrl Pts',(-0.255766169251004,-7.95890872821688,
1.64811304057572));
#8516=CARTESIAN_POINT('Ctrl Pts',(-0.213609741650813,-8.50459204726909,
0.999526572161923));
#8517=CARTESIAN_POINT('Ctrl Pts',(-0.129296886450431,-8.89227422537169,
-0.87087821582871));
#8518=CARTESIAN_POINT('Ctrl Pts',(-0.00282760364985846,-6.84549107074519,
-2.90273595762506));
#8519=CARTESIAN_POINT('Ctrl Pts',(0.123641679150715,-4.03147363592819,-2.29102387700814));
#8520=CARTESIAN_POINT('Ctrl Pts',(0.250110961951288,-3.0048660809507,0.397450620628325));
#8521=CARTESIAN_POINT('Ctrl Pts',(0.376580244751861,-4.69833585942183,2.72694181908363));
#8522=CARTESIAN_POINT('Ctrl Pts',(0.503049527552434,-7.57381067700105,2.57901747640416));
#8523=CARTESIAN_POINT('Ctrl Pts',(0.629518810353007,-9.02010634361806,0.0895593516203334));
#8524=CARTESIAN_POINT('Ctrl Pts',(0.755988093153582,-7.72375616695671,-2.48150715181869));
#8525=CARTESIAN_POINT('Ctrl Pts',(0.882457375954152,-4.86203286070258,-2.79891511344676));
#8526=CARTESIAN_POINT('Ctrl Pts',(1.00892665875473,-3.03371871439761,-0.574639780338865));
#8527=CARTESIAN_POINT('Ctrl Pts',(1.1353959415553,-3.899155223165,2.17151868899145));
#8528=CARTESIAN_POINT('Ctrl Pts',(1.26186522435587,-6.67241573405984,2.94565054354541));
#8529=CARTESIAN_POINT('Ctrl Pts',(1.38833450715645,-8.83504078941567,1.04478035722949));
#8530=CARTESIAN_POINT('Ctrl Pts',(1.51480378995702,-8.42309989372086,-1.8048844843804));
#8531=CARTESIAN_POINT('Ctrl Pts',(1.64127307275759,-5.81068658220031,-3.01548936826444));
#8532=CARTESIAN_POINT('Ctrl Pts',(1.76774235555817,-3.37019302901635,-1.48766071233055));
#8533=CARTESIAN_POINT('Ctrl Pts',(1.89421163835874,-3.31788757417861,1.39114757259974));
#8534=CARTESIAN_POINT('Ctrl Pts',(2.02068092115931,-5.70126992189332,3.00662240928013));
#8535=CARTESIAN_POINT('Ctrl Pts',(2.14715020395988,-8.35593592155457,1.89171467455323));
#8536=CARTESIAN_POINT('Ctrl Pts',(2.27361948676046,-8.87112245100439,-0.941102672625564));
#8537=CARTESIAN_POINT('Ctrl Pts',(2.40008876956103,-6.77897681420636,-2.91928303105917));
#8538=CARTESIAN_POINT('Ctrl Pts',(2.5265580523616,-3.9794244582753,-2.24639552297924));
#8539=CARTESIAN_POINT('Ctrl Pts',(2.65302733516218,-3.01480311105916,0.466495315099294));
#8540=CARTESIAN_POINT('Ctrl Pts',(2.77949661796275,-4.7611075477298,2.75575104615122));
#8541=CARTESIAN_POINT('Ctrl Pts',(2.90596590076332,-7.63247864459777,2.54244603125873));
#8542=CARTESIAN_POINT('Ctrl Pts',(3.03243518356389,-9.02135843007676,0.0202874415191203));
#8543=CARTESIAN_POINT('Ctrl Pts',(3.15890446636447,-7.66647330603156,-2.52029463810126));
#8544=CARTESIAN_POINT('Ctrl Pts',(3.28537374916504,-4.79822553871722,-2.77213933419203));
#8545=CARTESIAN_POINT('Ctrl Pts',(3.41184303196562,-3.02133673211591,-0.506540699172009));
#8546=CARTESIAN_POINT('Ctrl Pts',(3.53831231476618,-3.94944037876103,2.21905916619308));
#8547=CARTESIAN_POINT('Ctrl Pts',(3.66478159756677,-6.73970426360059,2.92948049079009));
#8548=CARTESIAN_POINT('Ctrl Pts',(3.79125088036733,-8.85822573557158,0.979573370365098));
#8549=CARTESIAN_POINT('Ctrl Pts',(3.91772016316791,-8.3811268405867,-1.85990680208812));
#8550=CARTESIAN_POINT('Ctrl Pts',(4.04418944596848,-5.74167203129455,-3.01036293559842));
#8551=CARTESIAN_POINT('Ctrl Pts',(4.17065872876906,-3.336810777222,-1.42703942030501));
#8552=CARTESIAN_POINT('Ctrl Pts',(4.29712801156963,-3.3504527581017,1.45221133323505));
#8553=CARTESIAN_POINT('Ctrl Pts',(4.4235972943702,-5.77020937810816,3.01267565687393));
#8554=CARTESIAN_POINT('Ctrl Pts',(4.55006657717077,-8.39864413395782,1.83726009646369));
#8555=CARTESIAN_POINT('Ctrl Pts',(4.67653585997135,-8.84881511949022,-1.00661350993934));
#8556=CARTESIAN_POINT('Ctrl Pts',(4.80300514277192,-6.71191173443704,-2.93635829315832));
#8557=CARTESIAN_POINT('Ctrl Pts',(4.92947442557249,-3.92850496989789,-2.19952874127408));
#8558=CARTESIAN_POINT('Ctrl Pts',(5.05594370837306,-3.02627036865852,0.534743324512047));
#8559=CARTESIAN_POINT('Ctrl Pts',(5.18241299117364,-4.82454787213973,2.7834027086531));
#8560=CARTESIAN_POINT('Ctrl Pts',(5.3088822739742,-7.69028042141618,2.50439023325154));
#8561=CARTESIAN_POINT('Ctrl Pts',(5.43535155677479,-9.02103053977556,-0.0489164713765121));
#8562=CARTESIAN_POINT('Ctrl Pts',(5.56182083957535,-7.60831351323712,-2.55780100605334));
#8563=CARTESIAN_POINT('Ctrl Pts',(5.68829012237593,-4.73505008567186,-2.743887763315));
#8564=CARTESIAN_POINT('Ctrl Pts',(5.81475940517651,-3.01051669714769,-0.438187089489962));
#8565=CARTESIAN_POINT('Ctrl Pts',(5.94122868797708,-4.00080168388066,2.26544133365983));
#8566=CARTESIAN_POINT('Ctrl Pts',(6.06769797077765,-6.80660452923693,2.9117705055246));
#8567=CARTESIAN_POINT('Ctrl Pts',(6.19416725357822,-8.87991129560537,0.913854076356023));
#8568=CARTESIAN_POINT('Ctrl Pts',(6.32063653637879,-8.33790454041667,-1.91395420617355));
#8569=CARTESIAN_POINT('Ctrl Pts',(6.44710581917937,-5.67279303335752,-3.00365676208316));
#8570=CARTESIAN_POINT('Ctrl Pts',(6.57357510197994,-3.30482567984171,-1.36566969922623));
#8571=CARTESIAN_POINT('Ctrl Pts',(6.70004438478051,-3.38440796204285,1.51251335016101));
#8572=CARTESIAN_POINT('Ctrl Pts',(6.8265136675811,-5.83926938364069,3.01714832455762));
#8573=CARTESIAN_POINT('Ctrl Pts',(6.95298295038165,-8.44009396559778,1.78184168277249));
#8574=CARTESIAN_POINT('Ctrl Pts',(7.07945223318224,-8.82501323416001,-1.07159627207705));
#8575=CARTESIAN_POINT('Ctrl Pts',(7.2059215159828,-6.6444731702528,-2.95189306651605));
#8576=CARTESIAN_POINT('Ctrl Pts',(7.33239079878339,-3.87867223432111,-2.15150804179754));
#8577=CARTESIAN_POINT('Ctrl Pts',(7.45886008158394,-3.03929771203367,0.602710797976159));
#8578=CARTESIAN_POINT('Ctrl Pts',(7.58532936438453,-4.88860486534565,2.80959413389628));
#8579=CARTESIAN_POINT('Ctrl Pts',(7.7117986471851,-7.74719543871252,2.46502057642963));
#8580=CARTESIAN_POINT('Ctrl Pts',(7.83826792998567,-9.01911774919456,-0.118094722276079));
#8581=CARTESIAN_POINT('Ctrl Pts',(7.96473721278625,-7.54930996179144,-2.5939654930144));
#8582=CARTESIAN_POINT('Ctrl Pts',(8.09120649558682,-4.67253825597884,-2.71419668832455));
#8583=CARTESIAN_POINT('Ctrl Pts',(8.21767577838739,-3.00126500864061,-0.369603594509102));
#8584=CARTESIAN_POINT('Ctrl Pts',(8.34414506118797,-4.05321182117459,2.31063499481999));
#8585=CARTESIAN_POINT('Ctrl Pts',(8.47061434398855,-6.87308161737107,2.89253294855792));
#8586=CARTESIAN_POINT('Ctrl Pts',(8.59708362678911,-8.90008601701954,0.847655336961254));
#8587=CARTESIAN_POINT('Ctrl Pts',(8.72355290958969,-8.29345566941167,-1.96699747432336));
#8588=CARTESIAN_POINT('Ctrl Pts',(8.85002219239025,-5.60408579766473,-2.99537486433416));
#8589=CARTESIAN_POINT('Ctrl Pts',(8.97649147519084,-3.27425433636271,-1.30358339848609));
#8590=CARTESIAN_POINT('Ctrl Pts',(9.1029607579914,-3.41973573861403,1.57202164160968));
#8591=CARTESIAN_POINT('Ctrl Pts',(9.22943004079198,-5.90841299622533,3.0200385622781));
#8592=CARTESIAN_POINT('Ctrl Pts',(9.35589932359255,-8.48026503905977,1.72548764368831));
#8593=CARTESIAN_POINT('Ctrl Pts',(9.48236860639313,-8.79972666043973,-1.1360152599871));
#8594=CARTESIAN_POINT('Ctrl Pts',(9.60883788919369,-6.57670152087419,-2.96588225471199));
#8595=CARTESIAN_POINT('Ctrl Pts',(9.73530717199427,-3.82994278657406,-2.10235278507697));
#8596=CARTESIAN_POINT('Ctrl Pts',(9.86177645479484,-3.0538966982477,0.670350921387973));
#8597=CARTESIAN_POINT('Ctrl Pts',(9.98824573759542,-4.95320971865872,2.83433293290292));
#8598=CARTESIAN_POINT('Ctrl Pts',(10.114715020396,-7.80326121920459,2.4243168480084));
#8599=CARTESIAN_POINT('Ctrl Pts',(10.2411843031966,-9.01549208379667,-0.187132795629694));
#8600=CARTESIAN_POINT('Ctrl Pts',(10.3676535859971,-7.48974052152724,-2.62891886486708));
#8601=CARTESIAN_POINT('Ctrl Pts',(10.4941228687977,-4.61024985438304,-2.68279494587922));
#8602=CARTESIAN_POINT('Ctrl Pts',(10.6205921515983,-2.99449524434074,-0.301376201410799));
#8603=CARTESIAN_POINT('Ctrl Pts',(10.7470614343989,-4.10487349734913,2.35567967460553));
#8604=CARTESIAN_POINT('Ctrl Pts',(10.8735307171994,-6.94276063434935,2.8696483143193));
#8605=CARTESIAN_POINT('Ctrl Pts',(10.9578435723998,-8.2538964667147,1.48053551427594));
#8606=CARTESIAN_POINT('Ctrl Pts',(11.,-8.47299490241841,0.661737268568548));
#8607=CARTESIAN_POINT('Ctrl Pts',(-2.77555756156289E-16,-7.61992569438872,
1.36291222925734));
#8608=CARTESIAN_POINT('Ctrl Pts',(-2.8415648060146E-16,-7.67340551349811,
1.31130789569533));
#8609=CARTESIAN_POINT('Ctrl Pts',(-2.12884066448237E-16,-7.72375637073556,
1.25685433110144));
#8610=CARTESIAN_POINT('Ctrl Pts',(-2.20309881449055E-16,-7.77098328294997,
1.19991834123266));
#8611=CARTESIAN_POINT('Ctrl Pts',(-2.2794194360023E-16,-7.81952189173417,
1.14140099151826));
#8612=CARTESIAN_POINT('Ctrl Pts',(-5.34217411271648E-16,-7.86476106583717,
1.08026093410145));
#8613=CARTESIAN_POINT('Ctrl Pts',(-5.30825383648903E-16,-7.90667917618666,
1.01684878351049));
#8614=CARTESIAN_POINT('Ctrl Pts',(-5.27540844822369E-16,-7.94726895796044,
0.955446078740799));
#8615=CARTESIAN_POINT('Ctrl Pts',(-1.29049571234523E-16,-7.98474497647301,
0.891912164254134));
#8616=CARTESIAN_POINT('Ctrl Pts',(-1.87350135405495E-16,-8.01905850567605,
0.826531736936219));
#8617=CARTESIAN_POINT('Ctrl Pts',(-2.12856632230295E-16,-8.03407067470238,
0.797927799984632));
#8618=CARTESIAN_POINT('Ctrl Pts',(-1.8986486044456E-16,-8.04847712697053,
0.76897005896662));
#8619=CARTESIAN_POINT('Ctrl Pts',(-1.87350135405495E-16,-8.06227182896166,
0.739680838297154));
#8620=CARTESIAN_POINT('Ctrl Pts',(-1.85669547491645E-16,-8.07149081277949,
0.720106885082177));
#8621=CARTESIAN_POINT('Ctrl Pts',(-1.91431563196273E-16,-8.08043654946019,
0.70038486767912));
#8622=CARTESIAN_POINT('Ctrl Pts',(-1.87350135405495E-16,-8.08910691796322,
0.680521268938271));
#8623=CARTESIAN_POINT('Ctrl Pts',(-1.84817515006514E-16,-8.09448708227411,
0.668195446224487));
#8624=CARTESIAN_POINT('Ctrl Pts',(-5.32249335375699E-16,-8.09975758272891,
0.65582334914044));
#8625=CARTESIAN_POINT('Ctrl Pts',(-5.13478148889135E-16,-8.1049165612927,
0.643411087671161));
#8626=CARTESIAN_POINT('Ctrl Pts',(-4.01571461942795E-16,-8.13567243277232,
0.569413897374587));
#8627=CARTESIAN_POINT('Ctrl Pts',(7.11652356572681E-17,-8.16248855621688,
0.493944535414431));
#8628=CARTESIAN_POINT('Ctrl Pts',(6.93889390390723E-17,-8.1853403815105,
0.417382497740407));
#8629=CARTESIAN_POINT('Ctrl Pts',(6.75847180162072E-17,-8.20855145064346,
0.33961686079112));
#8630=CARTESIAN_POINT('Ctrl Pts',(-3.39859180694956E-18,-8.22767309653215,
0.260723103319841));
#8631=CARTESIAN_POINT('Ctrl Pts',(-2.77555756156289E-17,-8.24263877411456,
0.181064199295853));
#8632=CARTESIAN_POINT('Ctrl Pts',(-4.9418863841957E-17,-8.25594936254853,
0.110214959044269));
#8633=CARTESIAN_POINT('Ctrl Pts',(-2.34406229728529E-16,-8.26597201859407,
0.0387595244952337));
#8634=CARTESIAN_POINT('Ctrl Pts',(-1.94289029309402E-16,-8.27262867129198,
-0.033060966067791));
#8635=CARTESIAN_POINT('Ctrl Pts',(-1.78758283697696E-16,-8.27520569009181,
-0.0608651437518981));
#8636=CARTESIAN_POINT('Ctrl Pts',(1.70471564310096E-16,-8.27727790351381,
-0.0887241302716296));
#8637=CARTESIAN_POINT('Ctrl Pts',(1.80411241501588E-16,-8.27883947623463,
-0.116624198769123));
#8638=CARTESIAN_POINT('Ctrl Pts',(1.85936496667142E-16,-8.27970752130047,
-0.132133253501507));
#8639=CARTESIAN_POINT('Ctrl Pts',(-2.39785655553094E-16,-8.28041776438053,
-0.147655004235494));
#8640=CARTESIAN_POINT('Ctrl Pts',(-2.4980018054066E-16,-8.28096910004911,
-0.163187100078598));
#8641=CARTESIAN_POINT('Ctrl Pts',(-2.58342787073613E-16,-8.28143940130555,
-0.176436313953894));
#8642=CARTESIAN_POINT('Ctrl Pts',(-9.71445146547012E-17,-8.28179374468433,
-0.189684521305536));
#8643=CARTESIAN_POINT('Ctrl Pts',(-9.71445146547012E-17,-8.28203184796289,
-0.202925957134301));
#8644=CARTESIAN_POINT('Ctrl Pts',(-9.71445146547012E-17,-8.2835319015313,
-0.286347164882211));
#8645=CARTESIAN_POINT('Ctrl Pts',(3.42590742071393E-16,-8.28042407041806,
-0.369551099405944));
#8646=CARTESIAN_POINT('Ctrl Pts',(2.4980018054066E-16,-8.27264922864484,
-0.452158464222489));
#8647=CARTESIAN_POINT('Ctrl Pts',(1.64944085125772E-16,-8.26553920899994,
-0.527702122060185));
#8648=CARTESIAN_POINT('Ctrl Pts',(-1.23009909160896E-16,-8.25452592361271,
-0.602747787578086));
#8649=CARTESIAN_POINT('Ctrl Pts',(-1.94289029309402E-16,-8.23952773590921,
-0.677016823098132));
#8650=CARTESIAN_POINT('Ctrl Pts',(-2.70259366732582E-16,-8.22354244627324,
-0.756173856417238));
#8651=CARTESIAN_POINT('Ctrl Pts',(-1.27582757010408E-16,-8.20303136853968,
-0.834449499034265));
#8652=CARTESIAN_POINT('Ctrl Pts',(-8.32667268468867E-17,-8.17825979510907,
-0.911615546253567));
#8653=CARTESIAN_POINT('Ctrl Pts',(-6.63256748201779E-17,-8.16879016272722,
-0.941114443510699));
#8654=CARTESIAN_POINT('Ctrl Pts',(1.29856532866623E-17,-8.15869737053701,
-0.970451130557648));
#8655=CARTESIAN_POINT('Ctrl Pts',(5.55111512312578E-17,-8.14799429148353,
-0.999612516884173));
#8656=CARTESIAN_POINT('Ctrl Pts',(7.48427287796255E-17,-8.1431288010665,
-1.01286893076376));
#8657=CARTESIAN_POINT('Ctrl Pts',(-2.0843408605211E-16,-8.1381371807216,
-1.02608911501842));
#8658=CARTESIAN_POINT('Ctrl Pts',(-1.94289029309402E-16,-8.1330205709451,
-1.03927181904394));
#8659=CARTESIAN_POINT('Ctrl Pts',(-1.81761449722105E-16,-8.12848904184923,
-1.05094709026127));
#8660=CARTESIAN_POINT('Ctrl Pts',(-3.0517213644317E-16,-8.12386085858254,
-1.062589268253));
#8661=CARTESIAN_POINT('Ctrl Pts',(-3.05311331771918E-16,-8.11914027396792,
-1.07418977377208));
#8662=CARTESIAN_POINT('Ctrl Pts',(-3.06245451009502E-16,-8.08746112969757,
-1.15203904837463));
#8663=CARTESIAN_POINT('Ctrl Pts',(1.46916949704505E-16,-8.05158497707301,
-1.22811622682948));
#8664=CARTESIAN_POINT('Ctrl Pts',(1.66533453693773E-16,-8.011854620096,
-1.30218190876206));
#8665=CARTESIAN_POINT('Ctrl Pts',(1.8637260655645E-16,-7.97167332042167,
-1.37708824204871));
#8666=CARTESIAN_POINT('Ctrl Pts',(3.72027912645227E-17,-7.92754941417975,
-1.44993793701178));
#8667=CARTESIAN_POINT('Ctrl Pts',(2.77555756156289E-17,-7.87978125494087,
-1.52047793744191));
#8668=CARTESIAN_POINT('Ctrl Pts',(1.82162073883537E-17,-7.83154714264218,
-1.59170601816577));
#8669=CARTESIAN_POINT('Ctrl Pts',(-2.18320265390652E-16,-7.77959686600608,
-1.66057998181683));
#8670=CARTESIAN_POINT('Ctrl Pts',(-2.4980018054066E-16,-7.72418728444125,
-1.72682140823545));
#8671=CARTESIAN_POINT('Ctrl Pts',(-2.62655382569273E-16,-7.70156011527822,
-1.75387189154257));
#8672=CARTESIAN_POINT('Ctrl Pts',(-7.7813004774142E-17,-7.67835553557515,
-1.78048309521614));
#8673=CARTESIAN_POINT('Ctrl Pts',(-8.32667268468867E-17,-7.65458894362178,
-1.80663469511614));
#8674=CARTESIAN_POINT('Ctrl Pts',(-8.66440684510765E-17,-7.63987094026128,
-1.82282966896707));
#8675=CARTESIAN_POINT('Ctrl Pts',(-2.43913607355091E-17,-7.62493270407027,
-1.8388530693696));
#8676=CARTESIAN_POINT('Ctrl Pts',(-5.55111512312578E-17,-7.60980251222269,
-1.85467449041822));
#8677=CARTESIAN_POINT('Ctrl Pts',(-1.84813850145164E-16,-7.54693657997148,
-1.92041247932014));
#8678=CARTESIAN_POINT('Ctrl Pts',(-7.96394343888385E-17,-7.48070447872273,
-1.98273188781124));
#8679=CARTESIAN_POINT('Ctrl Pts',(-1.38777878078145E-16,-7.41143126172467,
-2.04132873838597));
#8680=CARTESIAN_POINT('Ctrl Pts',(-1.83131710845124E-16,-7.35947634897613,
-2.08527637631701));
#8681=CARTESIAN_POINT('Ctrl Pts',(-3.08318371281544E-16,-7.30580954729488,
-2.12712980226528));
#8682=CARTESIAN_POINT('Ctrl Pts',(-3.05311331771918E-16,-7.25055002523813,
-2.1667490967338));
#8683=CARTESIAN_POINT('Ctrl Pts',(-3.04270587907503E-16,-7.2314245670102,
-2.18046143323572));
#8684=CARTESIAN_POINT('Ctrl Pts',(-5.15303059498705E-16,-7.21210820012051,
-2.19390604239713));
#8685=CARTESIAN_POINT('Ctrl Pts',(-5.55111512312578E-16,-7.19260549845642,
-2.20707675358934));
#8686=CARTESIAN_POINT('Ctrl Pts',(-5.87305517585258E-16,-7.17683321805303,
-2.21772820863456));
#8687=CARTESIAN_POINT('Ctrl Pts',(-8.35843188115225E-16,-7.16094634262041,
-2.22819555243348));
#8688=CARTESIAN_POINT('Ctrl Pts',(-8.04911692853238E-16,-7.14495254626684,
-2.23847286770512));
#8689=CARTESIAN_POINT('Ctrl Pts',(-6.6023125743896E-16,-7.07014240854922,
-2.28654446708293));
#8690=CARTESIAN_POINT('Ctrl Pts',(6.61429474879476E-17,-6.99296303382602,
-2.33048352074413));
#8691=CARTESIAN_POINT('Ctrl Pts',(1.66533453693773E-16,-6.91368947490656,
-2.36999461204078));
#8692=CARTESIAN_POINT('Ctrl Pts',(2.48179831249947E-16,-6.84921725371376,
-2.40212850198302));
#8693=CARTESIAN_POINT('Ctrl Pts',(-6.79181988010686E-17,-6.78335891798408,
-2.43133326054258));
#8694=CARTESIAN_POINT('Ctrl Pts',(-5.55111512312578E-17,-6.71624580957888,
-2.4574306487719));
#8695=CARTESIAN_POINT('Ctrl Pts',(3.78536928224624E-18,-6.69861361567082,
-2.4642870471818));
#8696=CARTESIAN_POINT('Ctrl Pts',(-6.28715915022922E-17,-6.68089474419301,
-2.47092885494305));
#8697=CARTESIAN_POINT('Ctrl Pts',(-5.55111512312578E-17,-6.66309273064558,
-2.4773571349477));
#8698=CARTESIAN_POINT('Ctrl Pts',(1.2890562790225,-3.88215585431528,-0.00180833227560233));
#8699=CARTESIAN_POINT('Ctrl Pts',(1.28093512868358,-3.88093924960685,-0.136660466501262));
#8700=CARTESIAN_POINT('Ctrl Pts',(1.27281397834465,-3.89272649643071,-0.271300596775523));
#8701=CARTESIAN_POINT('Ctrl Pts',(1.26469282800573,-3.91829200827257,-0.403271347036546));
#8702=CARTESIAN_POINT('Ctrl Pts',(1.22253640040554,-4.05100112016495,-1.0883239746252));
#8703=CARTESIAN_POINT('Ctrl Pts',(1.18037997280535,-4.55497781908782,-1.70144778714986));
#8704=CARTESIAN_POINT('Ctrl Pts',(1.13822354520516,-5.20138467371462,-1.96426277578416));
#8705=CARTESIAN_POINT('Ctrl Pts',(1.09606711760497,-5.84779152834142,-2.22707776441846));
#8706=CARTESIAN_POINT('Ctrl Pts',(1.05391069000478,-6.63662853867215,-2.13958392916239));
#8707=CARTESIAN_POINT('Ctrl Pts',(1.01175426240459,-7.20971718211825,-1.74147843160073));
#8708=CARTESIAN_POINT('Ctrl Pts',(0.969597834804394,-7.78280582556434,-1.34337293403907));
#8709=CARTESIAN_POINT('Ctrl Pts',(0.927441407204202,-8.14014610212581,-0.634655774171833));
#8710=CARTESIAN_POINT('Ctrl Pts',(0.885284979604011,-8.11947978687606,0.0628136684028912));
#8711=CARTESIAN_POINT('Ctrl Pts',(0.843128552003819,-8.09881347162631,0.760283110977616));
#8712=CARTESIAN_POINT('Ctrl Pts',(0.800972124403629,-7.70014056456535,1.44650483625982));
#8713=CARTESIAN_POINT('Ctrl Pts',(0.758815696803438,-7.10449029665888,1.81000344847466));
#8714=CARTESIAN_POINT('Ctrl Pts',(0.716659269203247,-6.50884002875241,2.17350206068949));
#8715=CARTESIAN_POINT('Ctrl Pts',(0.674502841603055,-5.71621240000042,2.21427755983694));
#8716=CARTESIAN_POINT('Ctrl Pts',(0.632346414002864,-5.08649523139113,1.91360197170689));
#8717=CARTESIAN_POINT('Ctrl Pts',(0.590189986402673,-4.45677806278185,1.61292638357685));
#8718=CARTESIAN_POINT('Ctrl Pts',(0.548033558802483,-3.98997135431527,0.970799708169316));
#8719=CARTESIAN_POINT('Ctrl Pts',(0.505877131202292,-3.89806072103819,0.27919597258167));
#8720=CARTESIAN_POINT('Ctrl Pts',(0.500270180475695,-3.88583628881346,0.187210282889286));
#8721=CARTESIAN_POINT('Ctrl Pts',(0.494663229749097,-3.88024373829367,0.0943493479437828));
#8722=CARTESIAN_POINT('Ctrl Pts',(0.4890562790225,-3.88098062526521,0.00140302826277638));
#8723=CARTESIAN_POINT('Ctrl Pts',(0.,-5.33826273143149,-2.47299490241842));
#8724=CARTESIAN_POINT('Ctrl Pts',(0.042156427600191,-4.51946448572409,-2.25389646671472));
#8725=CARTESIAN_POINT('Ctrl Pts',(0.126469282800573,-3.13035187791014,-0.942759478034699));
#8726=CARTESIAN_POINT('Ctrl Pts',(0.252938565601146,-3.64432015505377,1.8951258406221));
#8727=CARTESIAN_POINT('Ctrl Pts',(0.379407848401719,-6.30137623450992,3.00550525361278));
#8728=CARTESIAN_POINT('Ctrl Pts',(0.505877131202293,-8.68279501755112,1.3897499208415));
#8729=CARTESIAN_POINT('Ctrl Pts',(0.632346414002865,-8.62891891149828,-1.48974040295355));
#8730=CARTESIAN_POINT('Ctrl Pts',(0.758815696803439,-6.18713281460021,-3.01549224619728));
#8731=CARTESIAN_POINT('Ctrl Pts',(0.88528497960401,-3.57568308349712,-1.80326120932383));
#8732=CARTESIAN_POINT('Ctrl Pts',(1.01175426240459,-3.16566700707563,1.04679027585758));
#8733=CARTESIAN_POINT('Ctrl Pts',(1.13822354520516,-5.32964905792872,2.94610338914275));
#8734=CARTESIAN_POINT('Ctrl Pts',(1.26469282800573,-8.10235283801081,2.17005725520049));
#8735=CARTESIAN_POINT('Ctrl Pts',(1.3911621108063,-8.96588232345381,-0.576701529052951));
#8736=CARTESIAN_POINT('Ctrl Pts',(1.51763139360688,-7.13601528805713,-2.7997267301126));
#8737=CARTESIAN_POINT('Ctrl Pts',(1.64410067640745,-4.27451231466393,-2.48026509630649));
#8738=CARTESIAN_POINT('Ctrl Pts',(1.77056995920802,-2.97996136626914,0.0915870049917526));
#8739=CARTESIAN_POINT('Ctrl Pts',(1.8970392420086,-4.42797832080538,2.58026432327149));
#8740=CARTESIAN_POINT('Ctrl Pts',(2.02350852480917,-7.30358342959944,2.725745728157));
#8741=CARTESIAN_POINT('Ctrl Pts',(2.14997780760974,-8.99537493549262,0.395914211910863));
#8742=CARTESIAN_POINT('Ctrl Pts',(2.27644709041031,-7.9669975211319,-2.29345572403429));
#8743=CARTESIAN_POINT('Ctrl Pts',(2.40291637321089,-5.15234464286247,-2.90008608592962));
#8744=CARTESIAN_POINT('Ctrl Pts',(2.52938565601146,-3.10746698267462,-0.873081638157841));
#8745=CARTESIAN_POINT('Ctrl Pts',(2.65585493881204,-3.68936495023107,1.94678822513078));
#8746=CARTESIAN_POINT('Ctrl Pts',(2.7823242216126,-6.36960360330106,2.99873506265578));
#8747=CARTESIAN_POINT('Ctrl Pts',(2.90879350441318,-8.71419675286107,1.32746177559001));
#8748=CARTESIAN_POINT('Ctrl Pts',(3.03526278721375,-8.59396555469508,-1.5493099986334));
#8749=CARTESIAN_POINT('Ctrl Pts',(3.16173207001433,-6.1180947250836,-3.01911782098221));
#8750=CARTESIAN_POINT('Ctrl Pts',(3.2882013528149,-3.53497936495718,-1.74719548025824));
#8751=CARTESIAN_POINT('Ctrl Pts',(3.41467063561547,-3.19040579929669,1.11139516108156));
#8752=CARTESIAN_POINT('Ctrl Pts',(3.54113991841605,-5.39728918769256,2.96070235836602));
#8753=CARTESIAN_POINT('Ctrl Pts',(3.66760920121662,-8.15150809295624,2.12132781612021));
#8754=CARTESIAN_POINT('Ctrl Pts',(3.79407848401719,-8.95189313670652,-0.644473185577155));
#8755=CARTESIAN_POINT('Ctrl Pts',(3.92054776681777,-7.07159629755764,-2.82501330133343));
#8756=CARTESIAN_POINT('Ctrl Pts',(4.04701704961834,-4.21815827485875,-2.44009402361868));
#8757=CARTESIAN_POINT('Ctrl Pts',(4.17348633241891,-2.98285160370029,0.160730620181111));
#8758=CARTESIAN_POINT('Ctrl Pts',(4.29995561521949,-4.48748661387422,2.61559210015096));
#8759=CARTESIAN_POINT('Ctrl Pts',(4.42642489802005,-7.36566973169923,2.69517438424447));
#8760=CARTESIAN_POINT('Ctrl Pts',(4.55289418082063,-9.00365683350444,0.327206974422883));
#8761=CARTESIAN_POINT('Ctrl Pts',(4.67936346362121,-7.9139542516838,-2.33790459600758));
#8762=CARTESIAN_POINT('Ctrl Pts',(4.80583274642177,-5.08614590191431,-2.87991136408426));
#8763=CARTESIAN_POINT('Ctrl Pts',(4.93230202922235,-3.08822942523902,-0.806604548416513));
#8764=CARTESIAN_POINT('Ctrl Pts',(5.05877131202292,-3.73455861247221,1.99919836365645));
#8765=CARTESIAN_POINT('Ctrl Pts',(5.1852405948235,-6.43818709990916,2.98948337393659));
#8766=CARTESIAN_POINT('Ctrl Pts',(5.31170987762407,-8.74388782855944,1.26494994440632));
#8767=CARTESIAN_POINT('Ctrl Pts',(5.43817916042464,-8.55780106687306,-1.60831355147971));
#8768=CARTESIAN_POINT('Ctrl Pts',(5.56464844322523,-6.04891647253973,-3.02103061160996));
#8769=CARTESIAN_POINT('Ctrl Pts',(5.69111772602578,-3.49560970719883,-1.69028046160792));
#8770=CARTESIAN_POINT('Ctrl Pts',(5.81758700882637,-3.21659722516281,1.17545215581023));
#8771=CARTESIAN_POINT('Ctrl Pts',(5.94405629162693,-5.4652566627727,2.97372970205115));
#8772=CARTESIAN_POINT('Ctrl Pts',(6.07052557442751,-8.19952879357467,2.0714950793584));
#8773=CARTESIAN_POINT('Ctrl Pts',(6.19699485722808,-8.9363583629794,-0.711911751364896));
#8774=CARTESIAN_POINT('Ctrl Pts',(6.32346414002865,-7.00661353387476,-2.84881518722965));
#8775=CARTESIAN_POINT('Ctrl Pts',(6.44993342282923,-4.16273985984979,-2.39864419099309));
#8776=CARTESIAN_POINT('Ctrl Pts',(6.5764027056298,-2.98732427149032,0.22979062735577));
#8777=CARTESIAN_POINT('Ctrl Pts',(6.70287198843037,-4.54778863223406,2.64954730489951));
#8778=CARTESIAN_POINT('Ctrl Pts',(6.82934127123096,-7.42703945423727,2.66318928610364));
#8779=CARTESIAN_POINT('Ctrl Pts',(6.95581055403151,-9.01036300717914,0.25832797484807));
#8780=CARTESIAN_POINT('Ctrl Pts',(7.0822798368321,-7.85990684631327,-2.38112689720535));
#8781=CARTESIAN_POINT('Ctrl Pts',(7.20874911963266,-5.02042660634255,-2.85822580353484));
#8782=CARTESIAN_POINT('Ctrl Pts',(7.33521840243325,-3.07051943955244,-0.739704281189414));
#8783=CARTESIAN_POINT('Ctrl Pts',(7.4616876852338,-3.78094078104177,2.05055966999733));
#8784=CARTESIAN_POINT('Ctrl Pts',(7.58815696803439,-6.50654071121665,2.97866333871112));
#8785=CARTESIAN_POINT('Ctrl Pts',(7.71462625083495,-8.77213940010801,1.20177448985872));
#8786=CARTESIAN_POINT('Ctrl Pts',(7.84109553363553,-8.52029469802955,-1.66647334565703));
#8787=CARTESIAN_POINT('Ctrl Pts',(7.96756481643611,-5.9797125579978,-3.02135850191909));
#8788=CARTESIAN_POINT('Ctrl Pts',(8.09403409923667,-3.4575539082881,-1.63247868341485));
#8789=CARTESIAN_POINT('Ctrl Pts',(8.22050338203725,-3.24424888831968,1.23889248172823));
#8790=CARTESIAN_POINT('Ctrl Pts',(8.34697266483782,-5.5335046738129,2.98519695992403));
#8791=CARTESIAN_POINT('Ctrl Pts',(8.47344194763839,-8.24639557638579,2.02057558976858));
#8792=CARTESIAN_POINT('Ctrl Pts',(8.59991123043898,-8.91928310048972,-0.77897683272588));
#8793=CARTESIAN_POINT('Ctrl Pts',(8.72638051323954,-6.94110269497493,-2.87112251928));
#8794=CARTESIAN_POINT('Ctrl Pts',(8.85284979604013,-4.10828528051702,-2.35593597756347));
#8795=CARTESIAN_POINT('Ctrl Pts',(8.97931907884068,-2.99337751913424,0.298730085189438));
#8796=CARTESIAN_POINT('Ctrl Pts',(9.10578836164126,-4.60885239449141,2.68211248963539));
#8797=CARTESIAN_POINT('Ctrl Pts',(9.23225764444184,-7.48766074739694,2.6298070334431));
#8798=CARTESIAN_POINT('Ctrl Pts',(9.3587269272424,-9.01548944052047,0.189313422437645));
#8799=CARTESIAN_POINT('Ctrl Pts',(9.48519621004299,-7.80488452630467,-2.42309995159429));
#8800=CARTESIAN_POINT('Ctrl Pts',(9.61166549284354,-4.95521961969974,-2.83504085634446));
#8801=CARTESIAN_POINT('Ctrl Pts',(9.73813477564413,-3.05434938326512,-0.672415750957662));
#8802=CARTESIAN_POINT('Ctrl Pts',(9.86460405844471,-3.82848126493051,2.10084482849876));
#8803=CARTESIAN_POINT('Ctrl Pts',(9.99107334124527,-6.57463978426254,2.96628135292037));
#8804=CARTESIAN_POINT('Ctrl Pts',(10.1175426240459,-8.79891519692859,1.13796717239844));
#8805=CARTESIAN_POINT('Ctrl Pts',(10.2440119068464,-8.4815071817026,-1.72375621929785));
#8806=CARTESIAN_POINT('Ctrl Pts',(10.370481189647,-5.91044069571119,-3.02010639410425));
#8807=CARTESIAN_POINT('Ctrl Pts',(10.4969504724476,-3.42098237960844,-1.57381075447018));
#8808=CARTESIAN_POINT('Ctrl Pts',(10.6234197552481,-3.27305825140319,1.30166424671849));
#8809=CARTESIAN_POINT('Ctrl Pts',(10.7498890380487,-5.60254915406858,2.99513384905324));
#8810=CARTESIAN_POINT('Ctrl Pts',(10.8763583208493,-8.29102426622762,1.96852667642011));
#8811=CARTESIAN_POINT('Ctrl Pts',(11.0028276036498,-8.90273551252011,-0.8454915895703));
#8812=CARTESIAN_POINT('Ctrl Pts',(11.1292968864504,-6.870879053568,-2.89227340548826));
#8813=CARTESIAN_POINT('Ctrl Pts',(11.2136097416508,-5.00047342783812,-2.50459204726911));
#8814=CARTESIAN_POINT('Ctrl Pts',(11.255766169251,-4.35188695942431,-1.9589087282169));
#8815=CARTESIAN_POINT('Ctrl Pts',(-0.0852553897503347,-5.37643325356376,
-2.33034688916694));
#8816=CARTESIAN_POINT('Ctrl Pts',(-0.0430989621501437,-4.60486516708142,
-2.12388655333521));
#8817=CARTESIAN_POINT('Ctrl Pts',(0.0412138930502385,-3.29587975786923,
-0.888378950851187));
#8818=CARTESIAN_POINT('Ctrl Pts',(0.167683175850811,-3.78020116694325,1.7858106391383));
#8819=CARTESIAN_POINT('Ctrl Pts',(0.294152458651385,-6.28399216264951,2.83214082296819));
#8820=CARTESIAN_POINT('Ctrl Pts',(0.420621741451957,-8.52804525286687,1.30958596056379));
#8821=CARTESIAN_POINT('Ctrl Pts',(0.547091024252532,-8.47727684407722,-1.40380876252277));
#8822=CARTESIAN_POINT('Ctrl Pts',(0.673560307053103,-6.17633856500803,-2.84155174293356));
#8823=CARTESIAN_POINT('Ctrl Pts',(0.800029589853677,-3.71552323896728,-1.69924497029643));
#8824=CARTESIAN_POINT('Ctrl Pts',(0.926498872654249,-3.32915782945394,0.986409013851733));
#8825=CARTESIAN_POINT('Ctrl Pts',(1.05296815545482,-5.36831643648831,2.77616539417007));
#8826=CARTESIAN_POINT('Ctrl Pts',(1.17943743825539,-7.98108430842242,2.04488337967265));
#8827=CARTESIAN_POINT('Ctrl Pts',(1.30590672105597,-8.79480343422335,-0.543436063249505));
#8828=CARTESIAN_POINT('Ctrl Pts',(1.43237600385654,-7.07048732287362,-2.63823207627928));
#8829=CARTESIAN_POINT('Ctrl Pts',(1.55884528665711,-4.37404239859673,-2.33719772161069));
#8830=CARTESIAN_POINT('Ctrl Pts',(1.68531456945769,-3.1541641155846,0.0863040566569423));
#8831=CARTESIAN_POINT('Ctrl Pts',(1.81178385225826,-4.51865613381102,2.43142876399945));
#8832=CARTESIAN_POINT('Ctrl Pts',(1.93825313505883,-7.22838975000144,2.56851846805628));
#8833=CARTESIAN_POINT('Ctrl Pts',(2.06472241785941,-8.82259484481252,0.373076972864443));
#8834=CARTESIAN_POINT('Ctrl Pts',(2.19119170065998,-7.85353659641036,-2.16116394203596));
#8835=CARTESIAN_POINT('Ctrl Pts',(2.31766098346055,-5.20123934640569,-2.73280247446258));
#8836=CARTESIAN_POINT('Ctrl Pts',(2.44413026626113,-3.27431491583545,-0.822720288456811));
#8837=CARTESIAN_POINT('Ctrl Pts',(2.5705995490617,-3.82264767510706,1.83449301891556));
#8838=CARTESIAN_POINT('Ctrl Pts',(2.69706883186227,-6.34828402045441,2.82576115214061));
#8839=CARTESIAN_POINT('Ctrl Pts',(2.82353811466284,-8.55763566412181,1.25089073827407));
#8840=CARTESIAN_POINT('Ctrl Pts',(2.95000739746342,-8.44433967699588,-1.45994224741015));
#8841=CARTESIAN_POINT('Ctrl Pts',(3.07647668026399,-6.11128275070704,-2.84496818625629));
#8842=CARTESIAN_POINT('Ctrl Pts',(3.20294596306457,-3.67716740419206,-1.6464132409673));
#8843=CARTESIAN_POINT('Ctrl Pts',(3.32941524586514,-3.35246963144664,1.04728734124313));
#8844=CARTESIAN_POINT('Ctrl Pts',(3.45588452866571,-5.43205492855872,2.78992226139257));
#8845=CARTESIAN_POINT('Ctrl Pts',(3.58235381146628,-8.02740417561515,1.99896476631015));
#8846=CARTESIAN_POINT('Ctrl Pts',(3.70882309426686,-8.78162117582619,-0.607298495315348));
#8847=CARTESIAN_POINT('Ctrl Pts',(3.83529237706743,-7.009784167373,-2.66206006012371));
#8848=CARTESIAN_POINT('Ctrl Pts',(3.96176165986801,-4.32093898895219,-2.29934380845422));
#8849=CARTESIAN_POINT('Ctrl Pts',(4.08823094266858,-3.15688763749726,0.151459309668061));
#8850=CARTESIAN_POINT('Ctrl Pts',(4.21470022546915,-4.57473185216246,2.46471875374903));
#8851=CARTESIAN_POINT('Ctrl Pts',(4.34116950826972,-7.28689477191502,2.53971054931996));
#8852=CARTESIAN_POINT('Ctrl Pts',(4.46763879107029,-8.83039902396766,0.308332926288854));
#8853=CARTESIAN_POINT('Ctrl Pts',(4.59410807387087,-7.80355298430152,-2.20304890121183));
#8854=CARTESIAN_POINT('Ctrl Pts',(4.72057735667144,-5.13885910054086,-2.713791476807));
#8855=CARTESIAN_POINT('Ctrl Pts',(4.84704663947202,-3.2561870247988,-0.760077749595094));
#8856=CARTESIAN_POINT('Ctrl Pts',(4.97351592227259,-3.86523446334132,1.8838800205445));
#8857=CARTESIAN_POINT('Ctrl Pts',(5.09998520507316,-6.41291146380764,2.81704312202853));
#8858=CARTESIAN_POINT('Ctrl Pts',(5.22645448787374,-8.58561409053185,1.19198473276934));
#8859=CARTESIAN_POINT('Ctrl Pts',(5.35292377067431,-8.41026123970837,-1.51554234011181));
#8860=CARTESIAN_POINT('Ctrl Pts',(5.47939305347488,-6.0460948583034,-2.84677064273715));
#8861=CARTESIAN_POINT('Ctrl Pts',(5.60586233627545,-3.64006867851535,-1.59278121102298));
#8862=CARTESIAN_POINT('Ctrl Pts',(5.73233161907603,-3.37715027584678,1.10764938171857));
#8863=CARTESIAN_POINT('Ctrl Pts',(5.85880090187659,-5.49610188391745,2.80219815803961));
#8864=CARTESIAN_POINT('Ctrl Pts',(5.98527018467719,-8.07265493217446,1.95200649600478));
#8865=CARTESIAN_POINT('Ctrl Pts',(6.11173946747773,-8.76698248344817,-0.67084705008174));
#8866=CARTESIAN_POINT('Ctrl Pts',(6.23820875027832,-6.94854975841818,-2.68448899869544));
#8867=CARTESIAN_POINT('Ctrl Pts',(6.36467803307889,-4.26871723512147,-2.26028489716367));
#8868=CARTESIAN_POINT('Ctrl Pts',(6.49114731587947,-3.1611023115593,0.216535777366369));
#8869=CARTESIAN_POINT('Ctrl Pts',(6.61761659868004,-4.63155551191118,2.49671534447367));
#8870=CARTESIAN_POINT('Ctrl Pts',(6.74408588148062,-7.34472454821811,2.50957042493907));
#8871=CARTESIAN_POINT('Ctrl Pts',(6.87055516428118,-8.83671837017649,0.243427025257224));
#8872=CARTESIAN_POINT('Ctrl Pts',(6.99702444708176,-7.7526231571314,-2.24377804102541));
#8873=CARTESIAN_POINT('Ctrl Pts',(7.12349372988232,-5.07693064454441,-2.69335678908615));
#8874=CARTESIAN_POINT('Ctrl Pts',(7.2499630126829,-3.23949859167201,-0.697036443094767));
#8875=CARTESIAN_POINT('Ctrl Pts',(7.37643229548348,-3.90894120213532,1.93227868903264));
#8876=CARTESIAN_POINT('Ctrl Pts',(7.50290157828405,-6.4773222821712,2.80684721123077));
#8877=CARTESIAN_POINT('Ctrl Pts',(7.62937086108462,-8.61223604669034,1.13245338321713));
#8878=CARTESIAN_POINT('Ctrl Pts',(7.7558401438852,-8.37491832417184,-1.57034734407812));
#8879=CARTESIAN_POINT('Ctrl Pts',(7.88230942668576,-5.98088278414455,-2.84707961958182));
#8880=CARTESIAN_POINT('Ctrl Pts',(8.00877870948635,-3.604208025297,-1.5383135718585));
#8881=CARTESIAN_POINT('Ctrl Pts',(8.13524799228691,-3.40320692770437,1.16743032425354));
#8882=CARTESIAN_POINT('Ctrl Pts',(8.26171727508749,-5.56041319327916,2.81300395819925));
#8883=CARTESIAN_POINT('Ctrl Pts',(8.38818655788806,-8.11681833154999,1.904024159265));
#8884=CARTESIAN_POINT('Ctrl Pts',(8.51465584068864,-8.7508921612297,-0.734043663859012));
#8885=CARTESIAN_POINT('Ctrl Pts',(8.6411251234892,-6.8868177348351,-2.70550959271215));
#8886=CARTESIAN_POINT('Ctrl Pts',(8.7675944062898,-4.21740372071637,-2.22004019135766));
#8887=CARTESIAN_POINT('Ctrl Pts',(8.89406368909034,-3.1668063940071,0.281498649285935));
#8888=CARTESIAN_POINT('Ctrl Pts',(9.02053297189093,-4.68909697642373,2.52740209472543));
#8889=CARTESIAN_POINT('Ctrl Pts',(9.1470022546915,-7.40184906626454,2.47811373711298));
#8890=CARTESIAN_POINT('Ctrl Pts',(9.27347153749207,-8.8415490990946,0.178393390388182));
#8891=CARTESIAN_POINT('Ctrl Pts',(9.39994082029265,-7.70077465063371,-2.28332999344895));
#8892=CARTESIAN_POINT('Ctrl Pts',(9.52641010309321,-5.01548494632383,-2.67150920278189));
#8893=CARTESIAN_POINT('Ctrl Pts',(9.6528793858938,-3.22426126128772,-0.633629269489662));
#8894=CARTESIAN_POINT('Ctrl Pts',(9.77934866869436,-3.95373944196641,1.97966328435488));
#8895=CARTESIAN_POINT('Ctrl Pts',(9.90581795149494,-6.54149324462344,2.79517944675582));
#8896=CARTESIAN_POINT('Ctrl Pts',(10.0322872342955,-8.63746735418908,1.07232661805306));
#8897=CARTESIAN_POINT('Ctrl Pts',(10.1587565170961,-8.33836816067471,-1.62432601029408));
#8898=CARTESIAN_POINT('Ctrl Pts',(10.2852257998966,-5.91560668162263,-2.84589973621517));
#8899=CARTESIAN_POINT('Ctrl Pts',(10.4116950826972,-3.56974602620135,-1.48302974350269));
#8900=CARTESIAN_POINT('Ctrl Pts',(10.5381643654978,-3.43035450070375,1.22658126998721));
#8901=CARTESIAN_POINT('Ctrl Pts',(10.6646336482984,-5.62547502968677,2.82236766479144));
#8902=CARTESIAN_POINT('Ctrl Pts',(10.791102931099,-8.15887273628766,1.85497754651723));
#8903=CARTESIAN_POINT('Ctrl Pts',(10.9175722138995,-8.73529907605575,-0.796721697098993));
#8904=CARTESIAN_POINT('Ctrl Pts',(11.0440414967001,-6.82064475399369,-2.72544044733314));
#8905=CARTESIAN_POINT('Ctrl Pts',(11.1283543519005,-5.05812841110215,-2.36012143829251));
#8906=CARTESIAN_POINT('Ctrl Pts',(11.1705107795007,-4.44695389653044,-1.84591438360752));
#8907=CARTESIAN_POINT('Ctrl Pts',(-0.170510779500669,-5.41460377569604,
-2.18769887591546));
#8908=CARTESIAN_POINT('Ctrl Pts',(-0.128354351900478,-4.69026584843874,
-1.9938766399557));
#8909=CARTESIAN_POINT('Ctrl Pts',(-0.0440414967000964,-3.46140763782832,
-0.833998423667675));
#8910=CARTESIAN_POINT('Ctrl Pts',(0.0824277861004769,-3.91608217883272,
1.6764954376545));
#8911=CARTESIAN_POINT('Ctrl Pts',(0.208897068901049,-6.26660809078911,2.6587763923236));
#8912=CARTESIAN_POINT('Ctrl Pts',(0.335366351701623,-8.3732954881826,1.22942200028608));
#8913=CARTESIAN_POINT('Ctrl Pts',(0.461835634502196,-8.32563477665615,-1.31787712209198));
#8914=CARTESIAN_POINT('Ctrl Pts',(0.58830491730277,-6.16554431541587,-2.66761123966984));
#8915=CARTESIAN_POINT('Ctrl Pts',(0.714774200103341,-3.85536339443742,-1.59522873126902));
#8916=CARTESIAN_POINT('Ctrl Pts',(0.841243482903916,-3.49264865183227,0.926027751845885));
#8917=CARTESIAN_POINT('Ctrl Pts',(0.967712765704488,-5.40698381504787,2.60622739919738));
#8918=CARTESIAN_POINT('Ctrl Pts',(1.09418204850506,-7.85981577883405,1.91970950414481));
#8919=CARTESIAN_POINT('Ctrl Pts',(1.22065133130563,-8.62372454499285,-0.510170597446061));
#8920=CARTESIAN_POINT('Ctrl Pts',(1.34712061410621,-7.00495935769013,-2.47673742244596));
#8921=CARTESIAN_POINT('Ctrl Pts',(1.47358989690678,-4.47357248252952,-2.19413034691488));
#8922=CARTESIAN_POINT('Ctrl Pts',(1.60005917970735,-3.32836686490007,0.0810211083221311));
#8923=CARTESIAN_POINT('Ctrl Pts',(1.72652846250793,-4.60933394681663,2.28259320472741));
#8924=CARTESIAN_POINT('Ctrl Pts',(1.8529977453085,-7.15319607040347,2.41129120795556));
#8925=CARTESIAN_POINT('Ctrl Pts',(1.97946702810907,-8.64981475413239,0.350239733818021));
#8926=CARTESIAN_POINT('Ctrl Pts',(2.10593631090965,-7.74007567168883,-2.02887216003762));
#8927=CARTESIAN_POINT('Ctrl Pts',(2.23240559371022,-5.2501340499489,-2.56551886299555));
#8928=CARTESIAN_POINT('Ctrl Pts',(2.35887487651079,-3.44116284899628,-0.772358938755779));
#8929=CARTESIAN_POINT('Ctrl Pts',(2.48534415931136,-3.95593039998305,1.72219781270033));
#8930=CARTESIAN_POINT('Ctrl Pts',(2.61181344211194,-6.32696443760774,2.65278724162544));
#8931=CARTESIAN_POINT('Ctrl Pts',(2.73828272491251,-8.40107457538256,1.17431970095814));
#8932=CARTESIAN_POINT('Ctrl Pts',(2.86475200771309,-8.29471379929668,-1.37057449618689));
#8933=CARTESIAN_POINT('Ctrl Pts',(2.99122129051366,-6.10447077633046,-2.67081855153036));
#8934=CARTESIAN_POINT('Ctrl Pts',(3.11769057331424,-3.81935544342696,-1.54563100167637));
#8935=CARTESIAN_POINT('Ctrl Pts',(3.2441598561148,-3.51453346359658,0.983179521404702));
#8936=CARTESIAN_POINT('Ctrl Pts',(3.37062913891538,-5.4668206694249,2.61914216441911));
#8937=CARTESIAN_POINT('Ctrl Pts',(3.49709842171595,-7.90330025827405,1.87660171650009));
#8938=CARTESIAN_POINT('Ctrl Pts',(3.62356770451653,-8.61134921494586,-0.570123805053538));
#8939=CARTESIAN_POINT('Ctrl Pts',(3.75003698731709,-6.94797203718836,-2.49910681891398));
#8940=CARTESIAN_POINT('Ctrl Pts',(3.87650627011767,-4.42371970304562,-2.15859359328975));
#8941=CARTESIAN_POINT('Ctrl Pts',(4.00297555291824,-3.33092367129424,0.142187999155009));
#8942=CARTESIAN_POINT('Ctrl Pts',(4.12944483571882,-4.66197709045071,2.31384540734709));
#8943=CARTESIAN_POINT('Ctrl Pts',(4.25591411851939,-7.2081198121308,2.38424671439544));
#8944=CARTESIAN_POINT('Ctrl Pts',(4.38238340131996,-8.65714121443088,0.289458878154826));
#8945=CARTESIAN_POINT('Ctrl Pts',(4.50885268412053,-7.69315171691924,-2.06819320641608));
#8946=CARTESIAN_POINT('Ctrl Pts',(4.63532196692111,-5.19157229916742,-2.54767158952975));
#8947=CARTESIAN_POINT('Ctrl Pts',(4.76179124972168,-3.42414462435858,-0.71355095077367));
#8948=CARTESIAN_POINT('Ctrl Pts',(4.88826053252226,-3.99591031421044,1.76856167743254));
#8949=CARTESIAN_POINT('Ctrl Pts',(5.01472981532283,-6.3876358277061,2.64460287012047));
#8950=CARTESIAN_POINT('Ctrl Pts',(5.1411990981234,-8.42734035250428,1.11901952113236));
#8951=CARTESIAN_POINT('Ctrl Pts',(5.26766838092397,-8.26272141254368,-1.4227711287439));
#8952=CARTESIAN_POINT('Ctrl Pts',(5.39413766372455,-6.04327324406706,-2.67251067386434));
#8953=CARTESIAN_POINT('Ctrl Pts',(5.52060694652512,-3.78452764983187,-1.49528196043805));
#8954=CARTESIAN_POINT('Ctrl Pts',(5.64707622932569,-3.53770332653075,1.03984660762691));
#8955=CARTESIAN_POINT('Ctrl Pts',(5.77354551212626,-5.52694710506219,2.63066661402806));
#8956=CARTESIAN_POINT('Ctrl Pts',(5.90001479492685,-7.94578107077427,1.83251791265116));
#8957=CARTESIAN_POINT('Ctrl Pts',(6.0264840777274,-8.59760660391693,-0.629782348798582));
#8958=CARTESIAN_POINT('Ctrl Pts',(6.15295336052799,-6.8904859829616,-2.52016281016122));
#8959=CARTESIAN_POINT('Ctrl Pts',(6.27942264332856,-4.37469461039316,-2.12192560333425));
#8960=CARTESIAN_POINT('Ctrl Pts',(6.40589192612913,-3.33488035162828,0.203280927376966));
#8961=CARTESIAN_POINT('Ctrl Pts',(6.53236120892971,-4.71532239158831,2.34388338404782));
#8962=CARTESIAN_POINT('Ctrl Pts',(6.65883049173027,-7.26240964219896,2.3559515637745));
#8963=CARTESIAN_POINT('Ctrl Pts',(6.78529977453086,-8.66307373317385,0.228526075666379));
#8964=CARTESIAN_POINT('Ctrl Pts',(6.91176905733142,-7.64533946794951,-2.10642918484546));
#8965=CARTESIAN_POINT('Ctrl Pts',(7.038238340132,-5.13343468274627,-2.52848777463746));
#8966=CARTESIAN_POINT('Ctrl Pts',(7.16470762293256,-3.40847774379157,-0.654368605000115));
#8967=CARTESIAN_POINT('Ctrl Pts',(7.29117690573314,-4.03694162322887,1.81399770806795));
#8968=CARTESIAN_POINT('Ctrl Pts',(7.41764618853371,-6.44810385312578,2.63503108375044));
#8969=CARTESIAN_POINT('Ctrl Pts',(7.54411547133429,-8.45233269327263,1.06313227657554));
#8970=CARTESIAN_POINT('Ctrl Pts',(7.67058475413486,-8.22954195031416,-1.47422134249921));
#8971=CARTESIAN_POINT('Ctrl Pts',(7.79705403693543,-5.98205301029128,-2.67280073724457));
#8972=CARTESIAN_POINT('Ctrl Pts',(7.92352331973601,-3.75086214230591,-1.44414846030215));
#8973=CARTESIAN_POINT('Ctrl Pts',(8.04999260253658,-3.56216496708905,1.09596816677885));
#8974=CARTESIAN_POINT('Ctrl Pts',(8.17646188533715,-5.58732171274542,2.64081095647447));
#8975=CARTESIAN_POINT('Ctrl Pts',(8.30293116813773,-7.9872410867142,1.78747272876143));
#8976=CARTESIAN_POINT('Ctrl Pts',(8.4294004509383,-8.58250122196968,-0.689110494992141));
#8977=CARTESIAN_POINT('Ctrl Pts',(8.55586973373887,-6.83253277469527,-2.53989666614431));
#8978=CARTESIAN_POINT('Ctrl Pts',(8.68233901653945,-4.32652216091571,-2.08414440515185));
#8979=CARTESIAN_POINT('Ctrl Pts',(8.80880829934001,-3.34023526887996,0.264267213382427));
#8980=CARTESIAN_POINT('Ctrl Pts',(8.9352775821406,-4.76934155835606,2.37269169981547));
#8981=CARTESIAN_POINT('Ctrl Pts',(9.06174686494116,-7.31603738513214,2.32642044078287));
#8982=CARTESIAN_POINT('Ctrl Pts',(9.18821614774174,-8.66760875766876,0.16747335833872));
#8983=CARTESIAN_POINT('Ctrl Pts',(9.31468543054231,-7.59666477496275,-2.1435600353036));
#8984=CARTESIAN_POINT('Ctrl Pts',(9.44115471334288,-5.07575027294792,-2.50797754921931));
#8985=CARTESIAN_POINT('Ctrl Pts',(9.56762399614347,-3.39417313931032,-0.594842788021662));
#8986=CARTESIAN_POINT('Ctrl Pts',(9.69409327894402,-4.07899761900233,1.85848174021101));
#8987=CARTESIAN_POINT('Ctrl Pts',(9.82056256174462,-6.50834670498434,2.62407754059128));
#8988=CARTESIAN_POINT('Ctrl Pts',(9.94703184454517,-8.47601951144958,1.00668606370768));
#8989=CARTESIAN_POINT('Ctrl Pts',(10.0735011273458,-8.19522913964682,-1.52489580129031));
#8990=CARTESIAN_POINT('Ctrl Pts',(10.1999704101463,-5.92077266753408,-2.67169307832608));
#8991=CARTESIAN_POINT('Ctrl Pts',(10.3264396929469,-3.71850967279424,-1.39224873253521));
#8992=CARTESIAN_POINT('Ctrl Pts',(10.4529089757475,-3.58765075000433,1.15149829325592));
#8993=CARTESIAN_POINT('Ctrl Pts',(10.579378258548,-5.64840090530495,2.64960148052965));
#8994=CARTESIAN_POINT('Ctrl Pts',(10.7058475413486,-8.02672120634771,1.74142841661435));
#8995=CARTESIAN_POINT('Ctrl Pts',(10.8323168241492,-8.56786263959136,-0.747951804627684));
#8996=CARTESIAN_POINT('Ctrl Pts',(10.9587861069498,-6.7704104544194,-2.55860748917802));
#8997=CARTESIAN_POINT('Ctrl Pts',(11.0430989621501,-5.11578339436617,-2.21565082931592));
#8998=CARTESIAN_POINT('Ctrl Pts',(11.0852553897503,-4.54202083363656,-1.73292003899813));
#8999=CARTESIAN_POINT('Ctrl Pts',(-0.255766169251004,-5.45277429782831,
-2.04505086266398));
#9000=CARTESIAN_POINT('Ctrl Pts',(-0.213609741650813,-4.77566652979606,
-1.8638667265762));
#9001=CARTESIAN_POINT('Ctrl Pts',(-0.129296886450431,-3.62693551778741,
-0.779617896484163));
#9002=CARTESIAN_POINT('Ctrl Pts',(-0.00282760364985816,-4.0519631907222,
1.5671802361707));
#9003=CARTESIAN_POINT('Ctrl Pts',(0.123641679150715,-6.24922401892871,2.48541196167901));
#9004=CARTESIAN_POINT('Ctrl Pts',(0.250110961951288,-8.21854572349833,1.14925804000838));
#9005=CARTESIAN_POINT('Ctrl Pts',(0.376580244751862,-8.1739927092351,-1.2319454816612));
#9006=CARTESIAN_POINT('Ctrl Pts',(0.503049527552435,-6.15475006582368,-2.49367073640612));
#9007=CARTESIAN_POINT('Ctrl Pts',(0.629518810353007,-3.99520354990758,-1.49121249224162));
#9008=CARTESIAN_POINT('Ctrl Pts',(0.755988093153581,-3.65613947421059,0.865646489840036));
#9009=CARTESIAN_POINT('Ctrl Pts',(0.882457375954153,-5.44565119360746,2.43628940422469));
#9010=CARTESIAN_POINT('Ctrl Pts',(1.00892665875473,-7.73854724924566,1.79453562861697));
#9011=CARTESIAN_POINT('Ctrl Pts',(1.1353959415553,-8.45264565576239,-0.476905131642614));
#9012=CARTESIAN_POINT('Ctrl Pts',(1.26186522435587,-6.93943139250662,-2.31524276861265));
#9013=CARTESIAN_POINT('Ctrl Pts',(1.38833450715645,-4.57310256646231,-2.05106297221908));
#9014=CARTESIAN_POINT('Ctrl Pts',(1.51480378995702,-3.50256961421554,0.0757381599873213));
#9015=CARTESIAN_POINT('Ctrl Pts',(1.64127307275759,-4.70001175982226,2.13375764545536));
#9016=CARTESIAN_POINT('Ctrl Pts',(1.76774235555817,-7.07800239080548,2.25406394785483));
#9017=CARTESIAN_POINT('Ctrl Pts',(1.89421163835874,-8.4770346634523,0.327402494771599));
#9018=CARTESIAN_POINT('Ctrl Pts',(2.02068092115931,-7.62661474696728,-1.89658037803929));
#9019=CARTESIAN_POINT('Ctrl Pts',(2.14715020395988,-5.29902875349213,-2.39823525152852));
#9020=CARTESIAN_POINT('Ctrl Pts',(2.27361948676046,-3.60801078215711,-0.721997589054746));
#9021=CARTESIAN_POINT('Ctrl Pts',(2.40008876956103,-4.08921312485905,1.6099026064851));
#9022=CARTESIAN_POINT('Ctrl Pts',(2.5265580523616,-6.30564485476107,2.47981333111027));
#9023=CARTESIAN_POINT('Ctrl Pts',(2.65302733516218,-8.24451348664331,1.0977486636422));
#9024=CARTESIAN_POINT('Ctrl Pts',(2.77949661796275,-8.14508792159745,-1.28120674496364));
#9025=CARTESIAN_POINT('Ctrl Pts',(2.90596590076332,-6.09765880195391,-2.49666891680443));
#9026=CARTESIAN_POINT('Ctrl Pts',(3.0324351835639,-3.96154348266185,-1.44484876238543));
#9027=CARTESIAN_POINT('Ctrl Pts',(3.15890446636447,-3.67659729574652,0.919071701566275));
#9028=CARTESIAN_POINT('Ctrl Pts',(3.28537374916505,-5.50158641029108,2.44836206744565));
#9029=CARTESIAN_POINT('Ctrl Pts',(3.41184303196561,-7.77919634093294,1.75423866669003));
#9030=CARTESIAN_POINT('Ctrl Pts',(3.53831231476619,-8.44107725406553,-0.532949114791734));
#9031=CARTESIAN_POINT('Ctrl Pts',(3.66478159756675,-6.88615990700371,-2.33615357770425));
#9032=CARTESIAN_POINT('Ctrl Pts',(3.79125088036734,-4.52650041713906,-2.01784337812529));
#9033=CARTESIAN_POINT('Ctrl Pts',(3.91772016316791,-3.50495970509121,0.132916688641959));
#9034=CARTESIAN_POINT('Ctrl Pts',(4.04418944596848,-4.74922232873896,2.16297206094515));
#9035=CARTESIAN_POINT('Ctrl Pts',(4.17065872876906,-7.12934485234659,2.22878287947092));
#9036=CARTESIAN_POINT('Ctrl Pts',(4.29712801156963,-8.48388340489409,0.270584830020798));
#9037=CARTESIAN_POINT('Ctrl Pts',(4.4235972943702,-7.58275044953696,-1.93333751162033));
#9038=CARTESIAN_POINT('Ctrl Pts',(4.55006657717077,-5.24428549779397,-2.38155170225249));
#9039=CARTESIAN_POINT('Ctrl Pts',(4.67653585997135,-3.59210222391837,-0.66702415195225));
#9040=CARTESIAN_POINT('Ctrl Pts',(4.80300514277192,-4.12658616507955,1.65324333432059));
#9041=CARTESIAN_POINT('Ctrl Pts',(4.92947442557249,-6.36236019160457,2.47216261821241));
#9042=CARTESIAN_POINT('Ctrl Pts',(5.05594370837307,-8.26906661447669,1.04605430949538));
#9043=CARTESIAN_POINT('Ctrl Pts',(5.18241299117363,-8.11518158537901,-1.32999991737599));
#9044=CARTESIAN_POINT('Ctrl Pts',(5.30888227397421,-6.04045162983072,-2.49825070499153));
#9045=CARTESIAN_POINT('Ctrl Pts',(5.43535155677479,-3.9289866211484,-1.39778270985311));
#9046=CARTESIAN_POINT('Ctrl Pts',(5.56182083957535,-3.69825637721472,0.972043833535256));
#9047=CARTESIAN_POINT('Ctrl Pts',(5.68829012237594,-5.55779232620694,2.45913507001652));
#9048=CARTESIAN_POINT('Ctrl Pts',(5.8147594051765,-7.81890720937406,1.71302932929755));
#9049=CARTESIAN_POINT('Ctrl Pts',(5.94122868797707,-8.4282307243857,-0.588717647515425));
#9050=CARTESIAN_POINT('Ctrl Pts',(6.06769797077766,-6.83242220750502,-2.35583662162701));
#9051=CARTESIAN_POINT('Ctrl Pts',(6.19416725357822,-4.48067198566484,-1.98356630950483));
#9052=CARTESIAN_POINT('Ctrl Pts',(6.3206365363788,-3.50865839169727,0.190026077387566));
#9053=CARTESIAN_POINT('Ctrl Pts',(6.44710581917937,-4.79908927126543,2.19105142362198));
#9054=CARTESIAN_POINT('Ctrl Pts',(6.57357510197995,-7.1800947361798,2.20233270260992));
#9055=CARTESIAN_POINT('Ctrl Pts',(6.70004438478052,-8.4894290961712,0.213625126075533));
#9056=CARTESIAN_POINT('Ctrl Pts',(6.82651366758109,-7.53805577876764,-1.96908032866552));
#9057=CARTESIAN_POINT('Ctrl Pts',(6.95298295038167,-5.18993872094813,-2.36361876018877));
#9058=CARTESIAN_POINT('Ctrl Pts',(7.07945223318223,-3.57745689591113,-0.611700766905466));
#9059=CARTESIAN_POINT('Ctrl Pts',(7.20592151598281,-4.16494204432244,1.69571672710326));
#9060=CARTESIAN_POINT('Ctrl Pts',(7.33239079878337,-6.41888542408033,2.46321495627009));
#9061=CARTESIAN_POINT('Ctrl Pts',(7.45886008158396,-8.29242933985495,0.99381116993395));
#9062=CARTESIAN_POINT('Ctrl Pts',(7.58532936438452,-8.08416557645646,-1.37809534092029));
#9063=CARTESIAN_POINT('Ctrl Pts',(7.7117986471851,-5.98322323643802,-2.49852185490731));
#9064=CARTESIAN_POINT('Ctrl Pts',(7.83826792998567,-3.89751625931481,-1.34998334874579));
#9065=CARTESIAN_POINT('Ctrl Pts',(7.96473721278624,-3.72112300647373,1.02450600930416));
#9066=CARTESIAN_POINT('Ctrl Pts',(8.09120649558683,-5.61423023221168,2.46861795474968));
#9067=CARTESIAN_POINT('Ctrl Pts',(8.21767577838738,-7.8576638418784,1.67092129825785));
#9068=CARTESIAN_POINT('Ctrl Pts',(8.34414506118797,-8.41411028270966,-0.644177326125271));
#9069=CARTESIAN_POINT('Ctrl Pts',(8.47061434398854,-6.77824781455544,-2.37428373957647));
#9070=CARTESIAN_POINT('Ctrl Pts',(8.59708362678912,-4.43564060111505,-1.94824861894604));
#9071=CARTESIAN_POINT('Ctrl Pts',(8.72355290958969,-3.51366414375281,0.247035777478924));
#9072=CARTESIAN_POINT('Ctrl Pts',(8.85002219239026,-4.8495861402884,2.21798130490551));
#9073=CARTESIAN_POINT('Ctrl Pts',(8.97649147519083,-7.23022570399973,2.17472714445275));
#9074=CARTESIAN_POINT('Ctrl Pts',(9.1029607579914,-8.4936684162429,0.156553326289256));
#9075=CARTESIAN_POINT('Ctrl Pts',(9.22943004079198,-7.49255489929179,-2.00379007715825));
#9076=CARTESIAN_POINT('Ctrl Pts',(9.35589932359255,-5.13601559957201,-2.34444589565673));
#9077=CARTESIAN_POINT('Ctrl Pts',(9.48236860639313,-3.56408501733291,-0.55605630655366));
#9078=CARTESIAN_POINT('Ctrl Pts',(9.60883788919369,-4.20425579603823,1.73730019606714));
#9079=CARTESIAN_POINT('Ctrl Pts',(9.73530717199427,-6.47520016534523,2.45297563442673));
#9080=CARTESIAN_POINT('Ctrl Pts',(9.86177645479484,-8.31457166871008,0.9410455093623));
#9081=CARTESIAN_POINT('Ctrl Pts',(9.98824573759542,-8.05209011861891,-1.42546559228654));
#9082=CARTESIAN_POINT('Ctrl Pts',(10.114715020396,-5.92593865344554,-2.49748642043699));
#9083=CARTESIAN_POINT('Ctrl Pts',(10.2411843031966,-3.86727331938714,-1.30146772156772));
#9084=CARTESIAN_POINT('Ctrl Pts',(10.3676535859971,-3.7449469993049,1.07641531652463));
#9085=CARTESIAN_POINT('Ctrl Pts',(10.4941228687977,-5.67132678092312,2.47683529626786));
#9086=CARTESIAN_POINT('Ctrl Pts',(10.6205921515983,-7.89456967640777,1.62787928671148));
#9087=CARTESIAN_POINT('Ctrl Pts',(10.7470614343989,-8.40042620312697,-0.699181912156376));
#9088=CARTESIAN_POINT('Ctrl Pts',(10.8735307171994,-6.72017615484511,-2.39177453102291));
#9089=CARTESIAN_POINT('Ctrl Pts',(10.9578435723998,-5.1734383776302,-2.07118022033933));
#9090=CARTESIAN_POINT('Ctrl Pts',(11.,-4.63708777074269,-1.61992569438875));
#9091=CARTESIAN_POINT('Ctrl Pts',(0.710943720977493,-3.88529148023119,0.00143577679747337));
#9092=CARTESIAN_POINT('Ctrl Pts',(0.725958511702855,-3.88370462621288,0.251703649744779));
#9093=CARTESIAN_POINT('Ctrl Pts',(0.740973302428217,-3.92480148471753,0.50146841535006));
#9094=CARTESIAN_POINT('Ctrl Pts',(0.75598809315358,-4.01090210672623,0.7346104785572));
#9095=CARTESIAN_POINT('Ctrl Pts',(0.798144520753771,-4.25264338067621,1.38919412796826));
#9096=CARTESIAN_POINT('Ctrl Pts',(0.840300948353962,-4.84914728714184,1.91274176609648));
#9097=CARTESIAN_POINT('Ctrl Pts',(0.882457375954153,-5.52954858298102,2.0675566225593));
#9098=CARTESIAN_POINT('Ctrl Pts',(0.924613803554344,-6.2099498788202,2.22237147902212));
#9099=CARTESIAN_POINT('Ctrl Pts',(0.966770231154535,-6.97424856403293,2.00845355381954));
#9100=CARTESIAN_POINT('Ctrl Pts',(1.00892665875473,-7.47541430772541,1.52292113117499));
#9101=CARTESIAN_POINT('Ctrl Pts',(1.05108308635492,-7.9765800514179,1.03738870853044));
#9102=CARTESIAN_POINT('Ctrl Pts',(1.09323951395511,-8.21461285359015,0.280241788443912));
#9103=CARTESIAN_POINT('Ctrl Pts',(1.1353959415553,-8.08142687746697,-0.404721277761024));
#9104=CARTESIAN_POINT('Ctrl Pts',(1.17755236915549,-7.9482409013438,-1.08968434396596));
#9105=CARTESIAN_POINT('Ctrl Pts',(1.21970879675568,-7.44383614692521,-1.7024635562893));
#9106=CARTESIAN_POINT('Ctrl Pts',(1.26186522435587,-6.79724563204187,-1.96482319638538));
#9107=CARTESIAN_POINT('Ctrl Pts',(1.30402165195606,-6.15065511715852,-2.22718283648146));
#9108=CARTESIAN_POINT('Ctrl Pts',(1.34617807955626,-5.36187884181042,-2.13912290435027));
#9109=CARTESIAN_POINT('Ctrl Pts',(1.38833450715645,-4.78906854542857,-1.74062608291694));
#9110=CARTESIAN_POINT('Ctrl Pts',(1.4292042450968,-4.23374144502328,-1.35429209806172));
#9111=CARTESIAN_POINT('Ctrl Pts',(1.47007398303714,-3.88139817629141,-0.676182206719062));
#9112=CARTESIAN_POINT('Ctrl Pts',(1.51094372097749,-3.87968050865492,0.000387557652718817));
#9113=CARTESIAN_POINT('Ctrl Pts',(0.,-5.33826273143149,-2.47299490241842));
#9114=CARTESIAN_POINT('Ctrl Pts',(-2.92724693099176E-17,-5.25697989275057,
-2.4435642712672));
#9115=CARTESIAN_POINT('Ctrl Pts',(-2.99936341022307E-16,-5.17756935254689,
-2.40977678328915));
#9116=CARTESIAN_POINT('Ctrl Pts',(-1.89084858881472E-16,-5.10023122457203,
-2.37194495869841));
#9117=CARTESIAN_POINT('Ctrl Pts',(-7.18194080198928E-17,-5.01841824137493,
-2.33192414993816));
#9118=CARTESIAN_POINT('Ctrl Pts',(-4.57952225898383E-17,-4.93892346844573,
-2.28737700375529));
#9119=CARTESIAN_POINT('Ctrl Pts',(-1.42247325030098E-16,-4.86201628003916,
-2.2386224339937));
#9120=CARTESIAN_POINT('Ctrl Pts',(-2.26642914665326E-16,-4.79472249018341,
-2.19596218545231));
#9121=CARTESIAN_POINT('Ctrl Pts',(-2.00387407623276E-16,-4.7294100208876,
-2.1500794498512));
#9122=CARTESIAN_POINT('Ctrl Pts',(-2.35922392732846E-16,-4.66628671304646,
-2.10116352691532));
#9123=CARTESIAN_POINT('Ctrl Pts',(-2.53035131662012E-16,-4.6358881443092,
-2.07760687095783));
#9124=CARTESIAN_POINT('Ctrl Pts',(-3.2047257499942E-16,-4.60599768971522,
-2.0533464896154));
#9125=CARTESIAN_POINT('Ctrl Pts',(-3.19189119579733E-16,-4.57664107890252,
-2.02840217529484));
#9126=CARTESIAN_POINT('Ctrl Pts',(-3.1838209901331E-16,-4.55818201260159,
-2.0127175053303));
#9127=CARTESIAN_POINT('Ctrl Pts',(7.43895006162374E-17,-4.53993404802187,
-1.99676241071069));
#9128=CARTESIAN_POINT('Ctrl Pts',(8.32667268468867E-17,-4.52190394786633,
-1.98054167968357));
#9129=CARTESIAN_POINT('Ctrl Pts',(8.90116125221388E-17,-4.51023579146075,
-1.97004445421036));
#9130=CARTESIAN_POINT('Ctrl Pts',(7.79192238295981E-17,-4.4986578632022,
-1.95943488921183));
#9131=CARTESIAN_POINT('Ctrl Pts',(6.93889390390723E-17,-4.48718711125359,
-1.94872872076412));
#9132=CARTESIAN_POINT('Ctrl Pts',(2.2232716586874E-17,-4.4237757077816,
-1.88954400731919));
#9133=CARTESIAN_POINT('Ctrl Pts',(4.19397816253999E-17,-4.3635270875017,
-1.82731321714168));
#9134=CARTESIAN_POINT('Ctrl Pts',(-1.38777878078145E-17,-4.30667267111207,
-1.76231318129999));
#9135=CARTESIAN_POINT('Ctrl Pts',(-6.93621648361292E-17,-4.25015763638879,
-1.69770115085661));
#9136=CARTESIAN_POINT('Ctrl Pts',(2.58690954382853E-17,-4.19699589124401,
-1.63035201337592));
#9137=CARTESIAN_POINT('Ctrl Pts',(8.32667268468867E-17,-4.14745830932095,
-1.56051094849616));
#9138=CARTESIAN_POINT('Ctrl Pts',(1.34697385004543E-16,-4.10307058147718,
-1.49793045788973));
#9139=CARTESIAN_POINT('Ctrl Pts',(-9.33899128459785E-17,-4.061592963968,
-1.43334849733583));
#9140=CARTESIAN_POINT('Ctrl Pts',(-6.93889390390723E-17,-4.02325540423893,
-1.36693099493323));
#9141=CARTESIAN_POINT('Ctrl Pts',(-5.86560681904612E-17,-4.00611142997633,
-1.33723009691511));
#9142=CARTESIAN_POINT('Ctrl Pts',(7.82310118249411E-18,-3.98959585928372,
-1.30716204921597));
#9143=CARTESIAN_POINT('Ctrl Pts',(2.77555756156289E-17,-3.97373166622007,
-1.27674142037156));
#9144=CARTESIAN_POINT('Ctrl Pts',(3.74452042303345E-17,-3.9660197215955,
-1.26195326164511));
#9145=CARTESIAN_POINT('Ctrl Pts',(-9.49971474458872E-17,-3.95846173087556,
-1.24708178147702));
#9146=CARTESIAN_POINT('Ctrl Pts',(-1.11022302462516E-16,-3.95106046924767,
-1.23212865136607));
#9147=CARTESIAN_POINT('Ctrl Pts',(-1.24039512540166E-16,-3.94504843520807,
-1.21998224555778));
#9148=CARTESIAN_POINT('Ctrl Pts',(9.31053158590645E-17,-3.93913962598101,
-1.20778137348506));
#9149=CARTESIAN_POINT('Ctrl Pts',(8.32667268468867E-17,-3.93334209561816,
-1.19554126456453));
#9150=CARTESIAN_POINT('Ctrl Pts',(2.31250162516845E-17,-3.89790272592621,
-1.12071944941997));
#9151=CARTESIAN_POINT('Ctrl Pts',(-2.12799513447933E-16,-3.86655381569021,
-1.04430634320813));
#9152=CARTESIAN_POINT('Ctrl Pts',(-1.2490009027033E-16,-3.83953904065545,
-0.96652881623346));
#9153=CARTESIAN_POINT('Ctrl Pts',(-3.70006670927268E-17,-3.81252426562069,
-0.888751289258792));
#9154=CARTESIAN_POINT('Ctrl Pts',(-1.0547503387958E-16,-3.78984315653003,
-0.809608619610107));
#9155=CARTESIAN_POINT('Ctrl Pts',(-5.55111512312578E-17,-3.771792971052,
-0.729317871740391));
#9156=CARTESIAN_POINT('Ctrl Pts',(-3.97331530418015E-18,-3.75351269548682,
-0.648003638256219));
#9157=CARTESIAN_POINT('Ctrl Pts',(-7.84506068365862E-17,-3.73998283358267,
-0.565510657724717));
#9158=CARTESIAN_POINT('Ctrl Pts',(-1.66533453693773E-16,-3.73112919653385,
-0.482230005571742));
#9159=CARTESIAN_POINT('Ctrl Pts',(-1.95786173270394E-16,-3.72818886284729,
-0.454572116998511));
#9160=CARTESIAN_POINT('Ctrl Pts',(-1.59064674227402E-16,-3.7257646987008,
-0.426827461643137));
#9161=CARTESIAN_POINT('Ctrl Pts',(-1.66533453693773E-16,-3.72385518185906,
-0.399010789812195));
#9162=CARTESIAN_POINT('Ctrl Pts',(-1.70624142804513E-16,-3.72280932961687,
-0.383775454899953));
#9163=CARTESIAN_POINT('Ctrl Pts',(-4.49435376951814E-17,-3.72191787183054,
-0.368518521180014));
#9164=CARTESIAN_POINT('Ctrl Pts',(-5.55111512312578E-17,-3.72118063008209,
-0.353242451045553));
#9165=CARTESIAN_POINT('Ctrl Pts',(-6.45230566500116E-17,-3.72055192116072,
-0.34021524308114));
#9166=CARTESIAN_POINT('Ctrl Pts',(2.46893114276546E-16,-3.72003567571262,
-0.32717962863387));
#9167=CARTESIAN_POINT('Ctrl Pts',(2.4980018054066E-16,-3.71963163365472,
-0.314144903841315));
#9168=CARTESIAN_POINT('Ctrl Pts',(2.68015743063415E-16,-3.71709992206001,
-0.232469832530885));
#9169=CARTESIAN_POINT('Ctrl Pts',(5.488286943559E-16,-3.71896449420722,
-0.150735215678331));
#9170=CARTESIAN_POINT('Ctrl Pts',(4.44089209850063E-16,-3.72509763830452,
-0.0693027887965301));
#9171=CARTESIAN_POINT('Ctrl Pts',(3.39217825146735E-16,-3.73123850597352,
0.0122321873124179));
#9172=CARTESIAN_POINT('Ctrl Pts',(2.59200975553029E-16,-3.74165909148088,
0.093465234547049));
#9173=CARTESIAN_POINT('Ctrl Pts',(3.33066907387547E-16,-3.75628187779841,
0.174020871474803));
#9174=CARTESIAN_POINT('Ctrl Pts',(4.05749365005722E-16,-3.77067037897056,
0.253285852251375));
#9175=CARTESIAN_POINT('Ctrl Pts',(1.15570041343854E-16,-3.7891279795921,
0.331895826436378));
#9176=CARTESIAN_POINT('Ctrl Pts',(8.32667268468867E-17,-3.81162326334501,
0.409467154655233));
#9177=CARTESIAN_POINT('Ctrl Pts',(7.02983539418161E-17,-3.82065413936675,
0.440608662167665));
#9178=CARTESIAN_POINT('Ctrl Pts',(-1.41317173045025E-16,-3.83033620254681,
0.471582407310852));
#9179=CARTESIAN_POINT('Ctrl Pts',(-1.66533453693773E-16,-3.84066913389938,
0.502361889653307));
#9180=CARTESIAN_POINT('Ctrl Pts',(-1.78089117460353E-16,-3.84540432391796,
0.516466957478861));
#9181=CARTESIAN_POINT('Ctrl Pts',(-1.91790833069298E-16,-3.85027647415249,
0.530531683564752));
#9182=CARTESIAN_POINT('Ctrl Pts',(-1.66533453693773E-16,-3.85528015633242,
0.544538943406607));
#9183=CARTESIAN_POINT('Ctrl Pts',(-3.24796012030796E-17,-3.88183726120405,
0.618882647744295));
#9184=CARTESIAN_POINT('Ctrl Pts',(2.04582574808049E-16,-3.91212927413511,
0.691710442324472));
#9185=CARTESIAN_POINT('Ctrl Pts',(3.88578058618805E-16,-3.94610117464232,
0.762666157003909));
#9186=CARTESIAN_POINT('Ctrl Pts',(5.25025058613771E-16,-3.97129398814151,
0.815285352866705));
#9187=CARTESIAN_POINT('Ctrl Pts',(3.51076268717821E-16,-3.99851141404213,
0.866874595241459));
#9188=CARTESIAN_POINT('Ctrl Pts',(3.60822483003176E-16,-4.02774432096395,
0.917275939864036));
#9189=CARTESIAN_POINT('Ctrl Pts',(3.64283941088971E-16,-4.03812665805127,
0.93517644325651));
#9190=CARTESIAN_POINT('Ctrl Pts',(1.25791190295242E-16,-4.04876332126932,
0.952926991687769));
#9191=CARTESIAN_POINT('Ctrl Pts',(1.11022302462516E-16,-4.05965421258269,
0.970520102081179));
#9192=CARTESIAN_POINT('Ctrl Pts',(1.00739750509289E-16,-4.06723678460943,
0.982768964262814));
#9193=CARTESIAN_POINT('Ctrl Pts',(2.31163055125436E-16,-4.07494162572207,
0.994939826680167));
#9194=CARTESIAN_POINT('Ctrl Pts',(2.4980018054066E-16,-4.08276363356959,
1.00702274898775));
#9195=CARTESIAN_POINT('Ctrl Pts',(3.47541887158804E-16,-4.12378586093371,
1.0703911827438));
#9196=CARTESIAN_POINT('Ctrl Pts',(3.68255127129089E-16,-4.16806493610171,
1.13140389034015));
#9197=CARTESIAN_POINT('Ctrl Pts',(4.44089209850063E-16,-4.21556997754234,
1.1897206136822));
#9198=CARTESIAN_POINT('Ctrl Pts',(5.08458397066477E-16,-4.25589301959016,
1.23922078495035));
#9199=CARTESIAN_POINT('Ctrl Pts',(7.76827601613562E-17,-4.29854102111365,
1.28677822183849));
#9200=CARTESIAN_POINT('Ctrl Pts',(5.55111512312578E-17,-4.34351204228601,
1.33216059575643));
#9201=CARTESIAN_POINT('Ctrl Pts',(5.00618174492108E-17,-4.35456501122752,
1.3433146668967));
#9202=CARTESIAN_POINT('Ctrl Pts',(-1.66995712675634E-17,-4.3657583778192,
1.35433722656524));
#9203=CARTESIAN_POINT('Ctrl Pts',(0.,-4.3770892093283,1.36522705282965));
#9204=CARTESIAN_POINT('Origin',(6.,-6.,0.));
#9205=CARTESIAN_POINT('Origin',(12.,-6.,0.));
#9206=CARTESIAN_POINT('Origin',(12.,6.,0.));
#9207=CARTESIAN_POINT('Origin',(80.,-7.,-6.));
#9208=CARTESIAN_POINT('',(80.,-7.,-6.));
#9209=CARTESIAN_POINT('',(20.,-7.,-6.));
#9210=CARTESIAN_POINT('',(20.,-7.,-6.));
#9211=CARTESIAN_POINT('',(20.,-7.,6.));
#9212=CARTESIAN_POINT('',(20.,-7.,-6.));
#9213=CARTESIAN_POINT('',(80.,-7.,6.));
#9214=CARTESIAN_POINT('',(20.,-7.,6.));
#9215=CARTESIAN_POINT('',(80.,-7.,-6.));
#9216=CARTESIAN_POINT('Origin',(80.,-5.00000000000001,-6.));
#9217=CARTESIAN_POINT('',(82.,-5.,-6.));
#9218=CARTESIAN_POINT('Origin',(80.,-5.00000000000001,-6.));
#9219=CARTESIAN_POINT('',(82.,-5.,6.));
#9220=CARTESIAN_POINT('Origin',(80.,-5.00000000000001,6.));
#9221=CARTESIAN_POINT('',(82.,-5.,-6.));
#9222=CARTESIAN_POINT('Origin',(82.,5.,-6.));
#9223=CARTESIAN_POINT('',(82.,5.,-6.));
#9224=CARTESIAN_POINT('',(82.,-5.,-6.));
#9225=CARTESIAN_POINT('',(82.,5.,6.));
#9226=CARTESIAN_POINT('',(82.,-5.,6.));
#9227=CARTESIAN_POINT('',(82.,5.,-6.));
#9228=CARTESIAN_POINT('Origin',(80.,5.00000000000001,-6.));
#9229=CARTESIAN_POINT('',(80.,7.,-6.));
#9230=CARTESIAN_POINT('Origin',(80.,5.00000000000001,-6.));
#9231=CARTESIAN_POINT('',(80.,7.,6.));
#9232=CARTESIAN_POINT('Origin',(80.,5.00000000000001,6.));
#9233=CARTESIAN_POINT('',(80.,7.,-6.));
#9234=CARTESIAN_POINT('Origin',(20.,7.,-6.));
#9235=CARTESIAN_POINT('',(20.,7.,-6.));
#9236=CARTESIAN_POINT('',(80.,7.,-6.));
#9237=CARTESIAN_POINT('',(20.,7.,6.));
#9238=CARTESIAN_POINT('',(80.,7.,6.));
#9239=CARTESIAN_POINT('',(20.,7.,-6.));
#9240=CARTESIAN_POINT('Origin',(20.,5.,-6.));
#9241=CARTESIAN_POINT('',(18.,5.,-6.));
#9242=CARTESIAN_POINT('Origin',(20.,5.,-6.));
#9243=CARTESIAN_POINT('',(18.,5.,6.));
#9244=CARTESIAN_POINT('Origin',(20.,5.,6.));
#9245=CARTESIAN_POINT('',(18.,5.,-6.));
#9246=CARTESIAN_POINT('Origin',(18.,-5.,-6.));
#9247=CARTESIAN_POINT('',(18.,-5.,-6.));
#9248=CARTESIAN_POINT('',(18.,5.,-6.));
#9249=CARTESIAN_POINT('',(18.,-5.,6.));
#9250=CARTESIAN_POINT('',(18.,5.,6.));
#9251=CARTESIAN_POINT('',(18.,-5.,-6.));
#9252=CARTESIAN_POINT('Origin',(20.,-5.,-6.));
#9253=CARTESIAN_POINT('Origin',(20.,-5.,-6.));
#9254=CARTESIAN_POINT('Origin',(20.,-5.,6.));
#9255=CARTESIAN_POINT('Origin',(22.,10.,-6.));
#9256=CARTESIAN_POINT('',(20.,10.,-6.));
#9257=CARTESIAN_POINT('',(22.,8.,-6.));
#9258=CARTESIAN_POINT('Origin',(22.,10.,-6.));
#9259=CARTESIAN_POINT('',(20.,10.,6.));
#9260=CARTESIAN_POINT('',(20.,10.,-6.));
#9261=CARTESIAN_POINT('',(22.,8.,6.));
#9262=CARTESIAN_POINT('Origin',(22.,10.,6.));
#9263=CARTESIAN_POINT('',(22.,8.,-6.));
#9264=CARTESIAN_POINT('Origin',(78.,8.,-6.));
#9265=CARTESIAN_POINT('',(78.,8.,-6.));
#9266=CARTESIAN_POINT('',(78.,8.,-6.));
#9267=CARTESIAN_POINT('',(78.,8.,6.));
#9268=CARTESIAN_POINT('',(78.,8.,6.));
#9269=CARTESIAN_POINT('',(78.,8.,-6.));
#9270=CARTESIAN_POINT('Origin',(78.,10.,-6.));
#9271=CARTESIAN_POINT('',(80.,10.,-6.));
#9272=CARTESIAN_POINT('Origin',(78.,10.,-6.));
#9273=CARTESIAN_POINT('',(80.,10.,6.));
#9274=CARTESIAN_POINT('Origin',(78.,10.,6.));
#9275=CARTESIAN_POINT('',(80.,10.,-6.));
#9276=CARTESIAN_POINT('Origin',(80.,12.,-6.));
#9277=CARTESIAN_POINT('',(80.,12.,-6.));
#9278=CARTESIAN_POINT('',(80.,12.,-6.));
#9279=CARTESIAN_POINT('',(80.,12.,6.));
#9280=CARTESIAN_POINT('',(80.,12.,6.));
#9281=CARTESIAN_POINT('',(80.,12.,-6.));
#9282=CARTESIAN_POINT('Origin',(96.,12.,-6.));
#9283=CARTESIAN_POINT('',(96.,12.,-6.));
#9284=CARTESIAN_POINT('',(96.,12.,-6.));
#9285=CARTESIAN_POINT('',(96.,12.,6.));
#9286=CARTESIAN_POINT('',(96.,12.,6.));
#9287=CARTESIAN_POINT('',(96.,12.,-6.));
#9288=CARTESIAN_POINT('Origin',(96.,-12.,-6.));
#9289=CARTESIAN_POINT('',(96.,-12.,-6.));
#9290=CARTESIAN_POINT('',(96.,-12.,-6.));
#9291=CARTESIAN_POINT('',(96.,-12.,6.));
#9292=CARTESIAN_POINT('',(96.,-12.,6.));
#9293=CARTESIAN_POINT('',(96.,-12.,-6.));
#9294=CARTESIAN_POINT('Origin',(80.,-12.,-6.));
#9295=CARTESIAN_POINT('',(80.,-12.,-6.));
#9296=CARTESIAN_POINT('',(80.,-12.,-6.));
#9297=CARTESIAN_POINT('',(80.,-12.,6.));
#9298=CARTESIAN_POINT('',(80.,-12.,6.));
#9299=CARTESIAN_POINT('',(80.,-12.,-6.));
#9300=CARTESIAN_POINT('Origin',(80.,-10.,-6.));
#9301=CARTESIAN_POINT('',(80.,-10.,-6.));
#9302=CARTESIAN_POINT('',(80.,-10.,-6.));
#9303=CARTESIAN_POINT('',(80.,-10.,6.));
#9304=CARTESIAN_POINT('',(80.,-10.,6.));
#9305=CARTESIAN_POINT('',(80.,-10.,-6.));
#9306=CARTESIAN_POINT('Origin',(78.,-10.,-6.));
#9307=CARTESIAN_POINT('',(78.,-8.,-6.));
#9308=CARTESIAN_POINT('Origin',(78.,-10.,-6.));
#9309=CARTESIAN_POINT('',(78.,-8.,6.));
#9310=CARTESIAN_POINT('Origin',(78.,-10.,6.));
#9311=CARTESIAN_POINT('',(78.,-8.,-6.));
#9312=CARTESIAN_POINT('Origin',(22.,-8.,-6.));
#9313=CARTESIAN_POINT('',(22.,-8.,-6.));
#9314=CARTESIAN_POINT('',(22.,-8.,-6.));
#9315=CARTESIAN_POINT('',(22.,-8.,6.));
#9316=CARTESIAN_POINT('',(22.,-8.,6.));
#9317=CARTESIAN_POINT('',(22.,-8.,-6.));
#9318=CARTESIAN_POINT('Origin',(22.,-10.,-6.));
#9319=CARTESIAN_POINT('',(20.,-10.,-6.));
#9320=CARTESIAN_POINT('Origin',(22.,-10.,-6.));
#9321=CARTESIAN_POINT('',(20.,-10.,6.));
#9322=CARTESIAN_POINT('Origin',(22.,-10.,6.));
#9323=CARTESIAN_POINT('',(20.,-10.,-6.));
#9324=CARTESIAN_POINT('Origin',(20.,-12.,-6.));
#9325=CARTESIAN_POINT('',(20.,-12.,-6.));
#9326=CARTESIAN_POINT('',(20.,-12.,-6.));
#9327=CARTESIAN_POINT('',(20.,-12.,6.));
#9328=CARTESIAN_POINT('',(20.,-12.,6.));
#9329=CARTESIAN_POINT('',(20.,-12.,-6.));
#9330=CARTESIAN_POINT('Origin',(0.,-12.,-6.));
#9331=CARTESIAN_POINT('',(0.,-12.,-6.));
#9332=CARTESIAN_POINT('',(0.,-12.,-6.));
#9333=CARTESIAN_POINT('',(0.,-12.,6.));
#9334=CARTESIAN_POINT('',(0.,-12.,6.));
#9335=CARTESIAN_POINT('',(0.,-12.,-6.));
#9336=CARTESIAN_POINT('Origin',(0.,12.,-6.));
#9337=CARTESIAN_POINT('',(0.,12.,-6.));
#9338=CARTESIAN_POINT('',(0.,12.,-6.));
#9339=CARTESIAN_POINT('',(0.,12.,6.));
#9340=CARTESIAN_POINT('',(0.,12.,6.));
#9341=CARTESIAN_POINT('',(0.,12.,-6.));
#9342=CARTESIAN_POINT('Origin',(20.,12.,-6.));
#9343=CARTESIAN_POINT('',(20.,12.,-6.));
#9344=CARTESIAN_POINT('',(20.,12.,-6.));
#9345=CARTESIAN_POINT('',(20.,12.,6.));
#9346=CARTESIAN_POINT('',(20.,12.,6.));
#9347=CARTESIAN_POINT('',(20.,12.,-6.));
#9348=CARTESIAN_POINT('Origin',(20.,10.,-6.));
#9349=CARTESIAN_POINT('',(20.,10.,-6.));
#9350=CARTESIAN_POINT('',(20.,10.,6.));
#9351=CARTESIAN_POINT('Origin',(48.,0.,6.));
#9352=CARTESIAN_POINT('Origin',(48.,0.,-6.));
#13787=UNCERTAINTY_MEASURE_WITH_UNIT(LENGTH_MEASURE(0.01),#13802,
'DISTANCE_ACCURACY_VALUE',
'Maximum model space distance between geometric entities at asserted c
onnectivities');
#13792=UNCERTAINTY_MEASURE_WITH_UNIT(LENGTH_MEASURE(0.01),#13802,
'DISTANCE_ACCURACY_VALUE',
'Maximum model space distance between geometric entities at asserted c
onnectivities');
#13796=(
GEOMETRIC_REPRESENTATION_CONTEXT(3)
GLOBAL_UNCERTAINTY_ASSIGNED_CONTEXT((#13787))
GLOBAL_UNIT_ASSIGNED_CONTEXT((#13802,#13804,#13805))
REPRESENTATION_CONTEXT('','3D')
);
#13801=(
GEOMETRIC_REPRESENTATION_CONTEXT(3)
GLOBAL_UNCERTAINTY_ASSIGNED_CONTEXT((#13792))
GLOBAL_UNIT_ASSIGNED_CONTEXT((#13802,#13804,#13805))
REPRESENTATION_CONTEXT('','3D')
);
#13802=(
LENGTH_UNIT()
NAMED_UNIT(*)
SI_UNIT(.MILLI.,.METRE.)
);
#13804=(
NAMED_UNIT(*)
PLANE_ANGLE_UNIT()
SI_UNIT($,.RADIAN.)
);
#13805=(
NAMED_UNIT(*)
SI_UNIT($,.STERADIAN.)
SOLID_ANGLE_UNIT()
);
#13809=SHAPE_DEFINITION_REPRESENTATION(#13817,#13836);
#13817=PRODUCT_DEFINITION_SHAPE('',$,#13845);
#13836=SHAPE_REPRESENTATION('',(#3802),#13796);
#13841=PRODUCT_DEFINITION_CONTEXT('part definition',#13867,'design');
#13845=PRODUCT_DEFINITION('Flexure finger','Flexure finger',#13853,#13841);
#13853=PRODUCT_DEFINITION_FORMATION('',$,#13872);
#13867=APPLICATION_CONTEXT(
'Core Data for Automotive Mechanical Design Process');
#13868=PRODUCT_CONTEXT('part definition',#13867,'mechanical');
#13872=PRODUCT('Flexure finger','Flexure finger',$,(#13868));
#13879=PRESENTATION_STYLE_ASSIGNMENT((#13886));
#13886=SURFACE_STYLE_USAGE(.BOTH.,#13893);
#13893=SURFACE_SIDE_STYLE('',(#13900));
#13900=SURFACE_STYLE_FILL_AREA(#13907);
#13907=FILL_AREA_STYLE('Sky blue',(#13914));
#13914=FILL_AREA_STYLE_COLOUR('Sky blue',#13921);
#13921=COLOUR_RGB('Sky blue',0.317647058823529,0.686274509803922,0.890196078431372);
ENDSEC;
END-ISO-10303-21;
